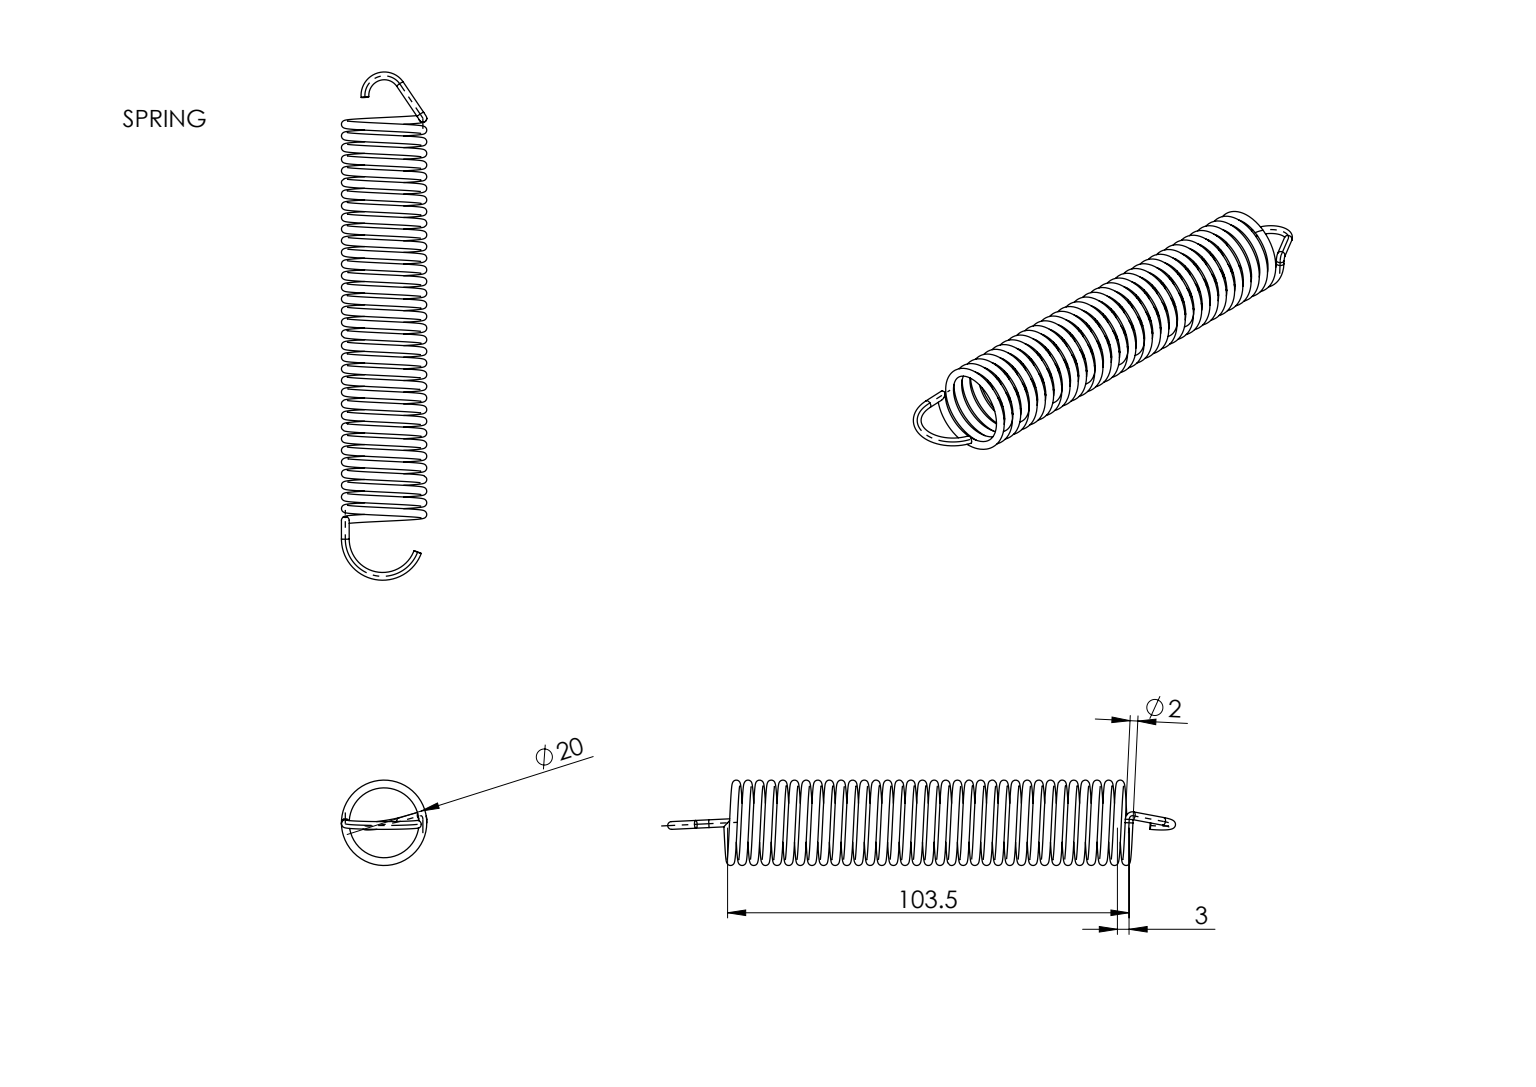
ISO-10303-21;
HEADER;
FILE_DESCRIPTION (('STEP AP214'),
    '1' );
FILE_NAME ('spring.step',
    '2026-10-08T07:58:12',
    ( '' ),
    ( '' ),
    'SwSTEP 2.0',
    'SolidWorks 2026',
    '' );
FILE_SCHEMA (( 'AUTOMOTIVE_DESIGN' ));
ENDSEC;

DATA;
#2=ORIENTED_EDGE ( 'NONE', *, *, #29028, .T. ) ;
#6=CARTESIAN_POINT ( 'NONE',  ( 2.517493886308900919, 214.5937144450984420, 40.40113791807857524 ) ) ;
#8=CARTESIAN_POINT ( 'NONE',  ( -10.00000000000000711, 206.9523078486584495, 26.49886208192143755 ) ) ;
#14=CARTESIAN_POINT ( 'NONE',  ( 6.500168698208244500, 202.3363017425938324, 1.298862081921434930 ) ) ;
#15=CARTESIAN_POINT ( 'NONE',  ( -8.118202686958039038, 201.1607312380087080, 39.20113791807857240 ) ) ;
#17=CARTESIAN_POINT ( 'NONE',  ( -8.118202686958039038, 201.1607312380087080, 30.20113791807856884 ) ) ;
#18=CARTESIAN_POINT ( 'NONE',  ( 6.220909254589680693, 198.5229672870052582, 103.4488620819214333 ) ) ;
#20=CARTESIAN_POINT ( 'NONE',  ( 4.903702542908435547, 213.8346818373419751, 96.54886208192142760 ) ) ;
#24=CARTESIAN_POINT ( 'NONE',  ( -12.00000000000000711, 207.0476921513413515, 12.50113791807856600 ) ) ;
#28=CARTESIAN_POINT ( 'NONE',  ( 0.05014649552810505201, 217.5146222423826714, 58.25113791807856245 ) ) ;
#35=CARTESIAN_POINT ( 'NONE',  ( -7.456977232089304408, 196.8216656703010301, 42.05113791807857382 ) ) ;
#38=CARTESIAN_POINT ( 'NONE',  ( -10.00000000000000711, 206.9523078486584495, 8.498862081921433997 ) ) ;
#41=CARTESIAN_POINT ( 'NONE',  ( -10.00000000000000711, 207.0476921513413515, 6.501137918078566003 ) ) ;
#42=CARTESIAN_POINT ( 'NONE',  ( -3.044812012440131443, 216.5253028482142952, 70.10113791807857808 ) ) ;
#45=CARTESIAN_POINT ( 'NONE',  ( -2.517493886309087880, 214.5937144450984135, 36.09886208192144608 ) ) ;
#48=CARTESIAN_POINT ( 'NONE',  ( 2.517493886308900919, 214.5937144450984420, 16.40113791807856458 ) ) ;
#49=CARTESIAN_POINT ( 'NONE',  ( -9.736236675708031640, 214.0148392665760753, 95.79886208192144181 ) ) ;
#54=CARTESIAN_POINT ( 'NONE',  ( 3.044812012440130555, 197.4746971517856764, 5.601137918078566535 ) ) ;
#55=CARTESIAN_POINT ( 'NONE',  ( 6.220909254589681581, 198.5229672870052582, 76.44886208192143329 ) ) ;
#58=CARTESIAN_POINT ( 'NONE',  ( 10.00000000000000711, 206.9523078486586201, 11.00113791807856600 ) ) ;
#61=CARTESIAN_POINT ( 'NONE',  ( -8.118202686958039038, 201.1607312380087080, 99.20113791807858661 ) ) ;
#63=CARTESIAN_POINT ( 'NONE',  ( 9.984503880673470277, 203.7031108863295401, 86.15113791807857524 ) ) ;
#66=CARTESIAN_POINT ( 'NONE',  ( -3.662846001189865142, 195.5725841191952838, 94.89886208192145034 ) ) ;
#71=CARTESIAN_POINT ( 'NONE',  ( -9.680171189290831535, 214.0920067884431148, 99.80113791807858092 ) ) ;
#74=CARTESIAN_POINT ( 'NONE',  ( -6.139770520408224463, 198.4640165459539105, 89.04886208192141339 ) ) ;
#76=CARTESIAN_POINT ( 'NONE',  ( 12.00000000000000711, 207.0476921513415220, 24.99886208192143400 ) ) ;
#78=CARTESIAN_POINT ( 'NONE',  ( 6.220909254589536808, 215.4770327129947702, 40.55113791807855250 ) ) ;
#80=CARTESIAN_POINT ( 'NONE',  ( -2.426778023690076225, 199.3768101843759553, 7.898862081921436129 ) ) ;
#83=CARTESIAN_POINT ( 'NONE',  ( 2.517493886309087436, 199.4062855549015865, 91.59886208192145318 ) ) ;
#86=CARTESIAN_POINT ( 'NONE',  ( 8.015496119326531499, 209.5516654185219636, 31.85113791807857453 ) ) ;
#92=CARTESIAN_POINT ( 'NONE',  ( 8.015496119326531499, 209.5516654185219636, 88.85113791807857808 ) ) ;
#96=CARTESIAN_POINT ( 'NONE',  ( 4.984841277089891776, 200.2242689037093726, 67.44886208192143329 ) ) ;
#99=CARTESIAN_POINT ( 'NONE',  ( 6.220909254589536808, 215.4770327129947987, 4.551137918078565825 ) ) ;
#104=CARTESIAN_POINT ( 'NONE',  ( -7.375838497908182134, 217.2372850707499765, 63.95113791807857240 ) ) ;
#106=CARTESIAN_POINT ( 'NONE',  ( -3.753561863808691168, 195.6020594897209435, 5.901137918078566358 ) ) ;
#107=CARTESIAN_POINT ( 'NONE',  ( 0.05014649552810506589, 217.5146222423826714, 88.25113791807858377 ) ) ;
#109=CARTESIAN_POINT ( 'NONE',  ( 12.00000000000000711, 207.0476921513415220, 48.99886208192143044 ) ) ;
#110=CARTESIAN_POINT ( 'NONE',  ( 3.135527875058981895, 197.5041725223112792, 61.59886208192143897 ) ) ;
#111=CARTESIAN_POINT ( 'NONE',  ( -0.05014649552807705357, 194.3824533091408000, 98.75113791807856956 ) ) ;
#113=CARTESIAN_POINT ( 'NONE',  ( -6.220909254589537696, 198.5229672870051161, 15.05113791807856671 ) ) ;
#114=CARTESIAN_POINT ( 'NONE',  ( 6.139770520408223575, 215.5359834540460611, 75.54886208192139918 ) ) ;
#117=CARTESIAN_POINT ( 'NONE',  ( -3.753561863808878130, 218.3979405102790281, 78.09886208192142476 ) ) ;
#119=CARTESIAN_POINT ( 'NONE',  ( -6.220909254589537696, 198.5229672870051161, 102.0511379180785383 ) ) ;
#122=CARTESIAN_POINT ( 'NONE',  ( 2.426778023690075337, 214.6231898156240447, 60.39886208192144323 ) ) ;
#130=CARTESIAN_POINT ( 'NONE',  ( 8.118202686958138514, 201.1607312380088501, 55.29886208192144181 ) ) ;
#135=CARTESIAN_POINT ( 'NONE',  ( -4.903702542908436435, 200.1653181626580249, 38.04886208192144892 ) ) ;
#136=CARTESIAN_POINT ( 'NONE',  ( 10.01549611932653860, 210.2015048109876716, 67.85113791807857808 ) ) ;
#138=CARTESIAN_POINT ( 'NONE',  ( 10.01549611932653860, 210.2015048109876716, 58.85113791807856387 ) ) ;
#140=CARTESIAN_POINT ( 'NONE',  ( -8.118202686958039038, 201.1607312380087080, 24.20113791807856884 ) ) ;
#141=CARTESIAN_POINT ( 'NONE',  ( -8.000000000000008882, 207.0476921513413515, 18.50113791807856956 ) ) ;
#145=CARTESIAN_POINT ( 'NONE',  ( -7.375838497908182134, 217.2372850707499765, 39.95113791807856529 ) ) ;
#147=CARTESIAN_POINT ( 'NONE',  ( 9.984503880673470277, 203.7031108863295401, 83.15113791807853261 ) ) ;
#148=CARTESIAN_POINT ( 'NONE',  ( -0.05014649552810635652, 196.4853777576173002, 56.75113791807856245 ) ) ;
#149=CARTESIAN_POINT ( 'NONE',  ( -9.736236675708031640, 214.0148392665760753, 23.79886208192143826 ) ) ;
#150=CARTESIAN_POINT ( 'NONE',  ( 0.05014649552828275014, 196.4853777576173002, 31.74886208192143044 ) ) ;
#153=CARTESIAN_POINT ( 'NONE',  ( -9.680171189290831535, 214.0920067884431148, 69.80113791807856671 ) ) ;
#154=CARTESIAN_POINT ( 'NONE',  ( -8.000000000000008882, 207.0476921513413515, 87.50113791807856956 ) ) ;
#156=CARTESIAN_POINT ( 'NONE',  ( 8.118202686958138514, 201.1607312380088501, 49.29886208192143471 ) ) ;
#160=CARTESIAN_POINT ( 'NONE',  ( -9.736236675708031640, 214.0148392665760753, 50.79886208192143471 ) ) ;
#164=EDGE_CURVE ( 'NONE', #11179, #4391, #29721, .T. ) ;
#167=CARTESIAN_POINT ( 'NONE',  ( -6.444103211791042618, 211.7408657792732356, 39.80113791807857382 ) ) ;
#169=CARTESIAN_POINT ( 'NONE',  ( -10.00000000000000711, 206.9523078486584495, 23.49886208192143755 ) ) ;
#176=CARTESIAN_POINT ( 'NONE',  ( -7.984503880673422316, 204.3529502787951628, 8.348862081921435419 ) ) ;
#178=CARTESIAN_POINT ( 'NONE',  ( -8.118202686958039038, 201.1607312380087080, 42.20113791807857240 ) ) ;
#180=CARTESIAN_POINT ( 'NONE',  ( -9.984503880673473830, 210.2968891136704315, 30.65113791807856813 ) ) ;
#181=CARTESIAN_POINT ( 'NONE',  ( -6.139770520408224463, 198.4640165459539105, 104.0488620819214276 ) ) ;
#184=CARTESIAN_POINT ( 'NONE',  ( -6.444103211790928043, 202.2591342207265939, 92.19886208192143329 ) ) ;
#188=CARTESIAN_POINT ( 'NONE',  ( 3.662846001190051659, 195.5725841191953691, 5.601137918078566535 ) ) ;
#192=CARTESIAN_POINT ( 'NONE',  ( 6.139770520408368348, 198.4640165459539674, 56.45113791807857950 ) ) ;
#193=CARTESIAN_POINT ( 'NONE',  ( -10.01549611932653860, 203.7984951890123000, 27.35113791807856742 ) ) ;
#200=CARTESIAN_POINT ( 'NONE',  ( 3.662846001190051659, 195.5725841191953691, 41.60113791807857098 ) ) ;
#202=CARTESIAN_POINT ( 'NONE',  ( -8.118202686958138514, 212.8392687619910930, 11.79886208192143471 ) ) ;
#205=CARTESIAN_POINT ( 'NONE',  ( 10.00000000000000711, 206.9523078486586201, 71.00113791807858377 ) ) ;
#208=CARTESIAN_POINT ( 'NONE',  ( 4.984841277089891776, 200.2242689037093726, 31.44886208192143684 ) ) ;
#211=CARTESIAN_POINT ( 'NONE',  ( -8.015496119326531499, 204.4483345814780364, 9.351137918078563871 ) ) ;
#214=CARTESIAN_POINT ( 'NONE',  ( 11.98450388067341876, 210.9467285061363953, 93.84886208192143897 ) ) ;
#219=CARTESIAN_POINT ( 'NONE',  ( -6.139770520408369237, 215.5359834540460042, 6.951137918078566180 ) ) ;
#221=CARTESIAN_POINT ( 'NONE',  ( 8.062137200540822946, 212.9164362838583315, 81.69886208192143329 ) ) ;
#225=CARTESIAN_POINT ( 'NONE',  ( 8.062137200540920645, 201.0835637161417822, 17.30113791807856671 ) ) ;
#232=CARTESIAN_POINT ( 'NONE',  ( -10.01549611932653860, 203.7984951890123284, 81.35113791807857808 ) ) ;
#236=CARTESIAN_POINT ( 'NONE',  ( 3.753561863808876797, 195.6020594897209719, 94.59886208192145318 ) ) ;
#242=CARTESIAN_POINT ( 'NONE',  ( -12.01549611932652972, 203.1486557965464499, 96.35113791807857808 ) ) ;
#246=CARTESIAN_POINT ( 'NONE',  ( -6.220909254589682469, 215.4770327129947134, 95.94886208192143329 ) ) ;
#247=CARTESIAN_POINT ( 'NONE',  ( -9.736236675708031640, 214.0148392665760753, 26.79886208192143826 ) ) ;
#249=CARTESIAN_POINT ( 'NONE',  ( 10.00000000000000711, 206.9523078486586201, 47.00113791807856956 ) ) ;
#251=CARTESIAN_POINT ( 'NONE',  ( -3.044812012439970683, 197.4746971517856196, 103.8988620819214361 ) ) ;
#254=CARTESIAN_POINT ( 'NONE',  ( -6.444103211790928043, 202.2591342207265939, 92.19886208192143329 ) ) ;
#256=CARTESIAN_POINT ( 'NONE',  ( 4.903702542908601636, 200.1653181626581102, 32.45113791807857240 ) ) ;
#262=CARTESIAN_POINT ( 'NONE',  ( 7.984503880673485376, 204.3529502787953902, 86.15113791807856103 ) ) ;
#266=CARTESIAN_POINT ( 'NONE',  ( 8.015496119326595448, 204.4483345814782638, 61.14886208192145034 ) ) ;
#269=CARTESIAN_POINT ( 'NONE',  ( 3.044812012440130555, 197.4746971517856764, -0.3988620819214342972 ) ) ;
#272=CARTESIAN_POINT ( 'NONE',  ( -7.375838497908182134, 217.2372850707499765, 66.95113791807857240 ) ) ;
#274=CARTESIAN_POINT ( 'NONE',  ( -8.062137200540920645, 212.9164362838581894, 87.80113791807856671 ) ) ;
#276=CARTESIAN_POINT ( 'NONE',  ( -9.680171189290716072, 199.9079932115567146, 50.19886208192144039 ) ) ;
#277=CARTESIAN_POINT ( 'NONE',  ( 3.044812012439969795, 216.5253028482143520, 57.39886208192143613 ) ) ;
#278=CARTESIAN_POINT ( 'NONE',  ( -12.01549611932652972, 203.1486557965464499, 93.35113791807857808 ) ) ;
#280=CARTESIAN_POINT ( 'NONE',  ( -10.00000000000000711, 207.0476921513413515, 12.50113791807856778 ) ) ;
#281=CARTESIAN_POINT ( 'NONE',  ( -3.044812012439970683, 197.4746971517856196, 76.89886208192143613 ) ) ;
#284=CARTESIAN_POINT ( 'NONE',  ( 8.118202686958039038, 212.8392687619912635, 100.7011379180785866 ) ) ;
#286=CARTESIAN_POINT ( 'NONE',  ( -0.05014649552828365914, 215.4116977939061144, 66.24886208192143044 ) ) ;
#289=DIRECTION ( 'NONE',  ( 0.000000000000000000, 0.9988620819214357738, 0.04769215134144196705 ) ) ;
#292=CARTESIAN_POINT ( 'NONE',  ( 6.444103211791042618, 202.2591342207267644, 59.30113791807857382 ) ) ;
#293=CARTESIAN_POINT ( 'NONE',  ( 3.135527875058981895, 197.5041725223112792, 52.59886208192143897 ) ) ;
#294=CARTESIAN_POINT ( 'NONE',  ( -9.945352646237287431, 205.9548993908332193, 104.4520571433695579 ) ) ;
#296=CARTESIAN_POINT ( 'NONE',  ( 2.426778023690075337, 214.6231898156240447, 36.39886208192144323 ) ) ;
#297=CARTESIAN_POINT ( 'NONE',  ( 9.984503880673470277, 203.7031108863295401, 83.15113791807853261 ) ) ;
#300=CARTESIAN_POINT ( 'NONE',  ( 9.984503880673470277, 203.7031108863295401, 56.15113791807856103 ) ) ;
#301=CARTESIAN_POINT ( 'NONE',  ( 8.118202686958039038, 212.8392687619912635, 25.70113791807856529 ) ) ;
#302=CARTESIAN_POINT ( 'NONE',  ( 4.984841277089725686, 213.7757310962907411, 13.55113791807856849 ) ) ;
#306=CARTESIAN_POINT ( 'NONE',  ( 7.375838497908181246, 196.7627149292499666, 35.45113791807855819 ) ) ;
#308=CARTESIAN_POINT ( 'NONE',  ( -6.220909254589537696, 198.5229672870051161, 90.05113791807858092 ) ) ;
#309=CARTESIAN_POINT ( 'NONE',  ( -10.00000000000000711, 207.0476921513413515, 60.50113791807857666 ) ) ;
#310=CARTESIAN_POINT ( 'NONE',  ( 12.01549611932659367, 203.1486557965466773, 22.14886208192143613 ) ) ;
#311=CARTESIAN_POINT ( 'NONE',  ( -0.05014649552828402690, 217.5146222423826714, 24.24886208192143044 ) ) ;
#313=CARTESIAN_POINT ( 'NONE',  ( 12.00000000000000711, 206.9523078486586485, 71.00113791807856956 ) ) ;
#314=CARTESIAN_POINT ( 'NONE',  ( 7.984503880673485376, 204.3529502787953902, 92.15113791807856103 ) ) ;
#315=CARTESIAN_POINT ( 'NONE',  ( -8.118202686958138514, 212.8392687619910930, 53.79886208192143471 ) ) ;
#318=CARTESIAN_POINT ( 'NONE',  ( -7.456977232089471386, 217.1783343296987709, 50.94886208192143329 ) ) ;
#323=CARTESIAN_POINT ( 'NONE',  ( 8.000000000000008882, 206.9523078486586485, 44.00113791807857666 ) ) ;
#326=CARTESIAN_POINT ( 'NONE',  ( 10.01549611932659545, 203.7984951890123853, 19.14886208192142902 ) ) ;
#332=CARTESIAN_POINT ( 'NONE',  ( 8.015496119326595448, 204.4483345814782638, 10.14886208192143435 ) ) ;
#333=CARTESIAN_POINT ( 'NONE',  ( -6.220909254589537696, 198.5229672870051161, 48.05113791807858092 ) ) ;
#336=CARTESIAN_POINT ( 'NONE',  ( 10.00000000000000711, 206.9523078486586201, 23.00113791807856600 ) ) ;
#339=CARTESIAN_POINT ( 'NONE',  ( 8.015496119326595448, 204.4483345814782638, 88.14886208192143613 ) ) ;
#343=CARTESIAN_POINT ( 'NONE',  ( 0.05014649552807549926, 219.6175466908591716, 7.251137918078565114 ) ) ;
#347=CARTESIAN_POINT ( 'NONE',  ( 6.139770520408368348, 198.4640165459539674, 59.45113791807855819 ) ) ;
#348=CARTESIAN_POINT ( 'NONE',  ( 8.062137200540920645, 201.0835637161417822, 32.30113791807857382 ) ) ;
#353=CARTESIAN_POINT ( 'NONE',  ( 10.01549611932659367, 203.7984951890124421, 4.148862081921434353 ) ) ;
#356=CARTESIAN_POINT ( 'NONE',  ( 7.375838497908181246, 196.7627149292499666, 38.45113791807856529 ) ) ;
#358=CARTESIAN_POINT ( 'NONE',  ( -10.01549611932659722, 210.2015048109875011, 23.64886208192142902 ) ) ;
#362=CARTESIAN_POINT ( 'NONE',  ( -6.139770520408369237, 215.5359834540460042, 66.95113791807858661 ) ) ;
#366=CARTESIAN_POINT ( 'NONE',  ( -2.517493886308901807, 199.4062855549015012, 17.90113791807856458 ) ) ;
#367=EDGE_CURVE ( 'NONE', #11826, #6694, #28121, .T. ) ;
#369=CARTESIAN_POINT ( 'NONE',  ( -12.00000000000000711, 206.9523078486584780, 101.4988620819214304 ) ) ;
#374=CARTESIAN_POINT ( 'NONE',  ( -6.139770520408369237, 215.5359834540460042, 9.951137918078567068 ) ) ;
#376=CARTESIAN_POINT ( 'NONE',  ( 6.220909254589681581, 198.5229672870052582, 82.44886208192141908 ) ) ;
#379=CARTESIAN_POINT ( 'NONE',  ( -10.01549611932653860, 203.7984951890123284, 9.351137918078569200 ) ) ;
#384=CARTESIAN_POINT ( 'NONE',  ( -6.220909254589537696, 198.5229672870051161, 99.05113791807858092 ) ) ;
#386=CARTESIAN_POINT ( 'NONE',  ( -8.118202686958039038, 201.1607312380087080, 81.20113791807857240 ) ) ;
#389=CARTESIAN_POINT ( 'NONE',  ( -7.456977232089471386, 217.1783343296987709, 92.94886208192144750 ) ) ;
#400=CARTESIAN_POINT ( 'NONE',  ( -8.062137200540822946, 201.0835637161416400, 95.19886208192143329 ) ) ;
#401=CARTESIAN_POINT ( 'NONE',  ( -3.753561863808878130, 218.3979405102790281, 33.09886208192143187 ) ) ;
#403=CARTESIAN_POINT ( 'NONE',  ( -8.118202686958039038, 201.1607312380087080, 39.20113791807857240 ) ) ;
#406=CARTESIAN_POINT ( 'NONE',  ( 4.984841277089891776, 200.2242689037093726, 1.448862081921434841 ) ) ;
#410=CARTESIAN_POINT ( 'NONE',  ( -2.517493886309087880, 214.5937144450984135, 90.09886208192143897 ) ) ;
#412=CARTESIAN_POINT ( 'NONE',  ( -8.000000000000008882, 207.0476921513413515, 27.50113791807856956 ) ) ;
#419=CARTESIAN_POINT ( 'NONE',  ( 7.984503880673485376, 204.3529502787953902, 89.15113791807856103 ) ) ;
#423=CARTESIAN_POINT ( 'NONE',  ( -8.015496119326597224, 209.5516654185217362, 77.64886208192143613 ) ) ;
#427=CARTESIAN_POINT ( 'NONE',  ( -9.984503880673475606, 210.2968891136704315, 15.65113791807856636 ) ) ;
#432=CARTESIAN_POINT ( 'NONE',  ( 12.01549611932652972, 210.8513442034534933, 76.85113791807856387 ) ) ;
#436=CARTESIAN_POINT ( 'NONE',  ( 10.01549611932653860, 210.2015048109876716, 97.85113791807857808 ) ) ;
#439=CARTESIAN_POINT ( 'NONE',  ( 7.375838497908012492, 217.2372850707501186, 51.54886208192144181 ) ) ;
#440=CARTESIAN_POINT ( 'NONE',  ( 6.139770520408223575, 215.5359834540460611, 69.54886208192142760 ) ) ;
#441=CARTESIAN_POINT ( 'NONE',  ( -3.753561863808878130, 218.3979405102790281, 6.098862081921433642 ) ) ;
#443=AXIS2_PLACEMENT_3D ( 'NONE', #26403, #3062, #13451 ) ;
#444=CARTESIAN_POINT ( 'NONE',  ( 3.135527875058820690, 216.4958274776887492, 10.40113791807856636 ) ) ;
#447=CARTESIAN_POINT ( 'NONE',  ( -3.044812012439970683, 197.4746971517856196, 79.89886208192143613 ) ) ;
#450=CARTESIAN_POINT ( 'NONE',  ( -6.139770520408369237, 215.5359834540460042, 99.95113791807855819 ) ) ;
#453=CARTESIAN_POINT ( 'NONE',  ( 6.444103211790928043, 211.7408657792734061, 60.69886208192144750 ) ) ;
#461=CARTESIAN_POINT ( 'NONE',  ( 8.015496119326531499, 209.5516654185219636, 58.85113791807857098 ) ) ;
#466=CARTESIAN_POINT ( 'NONE',  ( 7.984503880673422316, 209.6470497212048372, 36.84886208192142476 ) ) ;
#468=CARTESIAN_POINT ( 'NONE',  ( -10.00000000000000711, 207.0476921513413515, 84.50113791807856956 ) ) ;
#470=CARTESIAN_POINT ( 'NONE',  ( 8.118202686958039038, 212.8392687619912635, 70.70113791807857240 ) ) ;
#473=CARTESIAN_POINT ( 'NONE',  ( -2.426778023690262742, 214.6231898156240163, 19.10113791807856742 ) ) ;
#477=CARTESIAN_POINT ( 'NONE',  ( -12.01549611932652972, 203.1486557965464499, 39.35113791807856387 ) ) ;
#479=CARTESIAN_POINT ( 'NONE',  ( 3.044812012440130555, 197.4746971517856764, 98.60113791807857808 ) ) ;
#480=CARTESIAN_POINT ( 'NONE',  ( 10.01549611932653860, 210.2015048109876716, 61.85113791807857098 ) ) ;
#482=CARTESIAN_POINT ( 'NONE',  ( 9.736236675708031640, 199.9851607334238963, 22.29886208192143826 ) ) ;
#483=CARTESIAN_POINT ( 'NONE',  ( 10.00000000000000711, 207.0476921513415220, 36.99886208192143755 ) ) ;
#485=CARTESIAN_POINT ( 'NONE',  ( -11.98450388067348804, 210.9467285061362247, 69.65113791807856103 ) ) ;
#486=CARTESIAN_POINT ( 'NONE',  ( 8.015496119326531499, 209.5516654185219636, 85.85113791807857808 ) ) ;
#487=CARTESIAN_POINT ( 'NONE',  ( 6.139770520408223575, 215.5359834540460611, 48.54886208192143471 ) ) ;
#489=ORIENTED_EDGE ( 'NONE', *, *, #23335, .T. ) ;
#490=CARTESIAN_POINT ( 'NONE',  ( -3.662846001189865142, 195.5725841191952838, 52.89886208192143613 ) ) ;
#497=CARTESIAN_POINT ( 'NONE',  ( 11.98450388067341876, 210.9467285061363953, 54.84886208192143187 ) ) ;
#499=CARTESIAN_POINT ( 'NONE',  ( 6.500168698208129925, 211.6636982574063381, 37.70113791807857240 ) ) ;
#501=CARTESIAN_POINT ( 'NONE',  ( -3.044812012439970683, 197.4746971517856196, 22.89886208192143613 ) ) ;
#505=UNCERTAINTY_MEASURE_WITH_UNIT (LENGTH_MEASURE( 1.000000000000000082E-05 ), #16997, 'distance_accuracy_value', 'NONE');
#509=CARTESIAN_POINT ( 'NONE',  ( -4.984841277089891776, 213.7757310962905990, 2.948862081921435063 ) ) ;
#510=CARTESIAN_POINT ( 'NONE',  ( -9.984503880673473830, 210.2968891136704315, 54.65113791807858235 ) ) ;
#512=CARTESIAN_POINT ( 'NONE',  ( 0.05014649552810505201, 217.5146222423826714, 34.25113791807856956 ) ) ;
#515=CARTESIAN_POINT ( 'NONE',  ( -8.015496119326597224, 209.5516654185217362, 95.64886208192143613 ) ) ;
#519=CARTESIAN_POINT ( 'NONE',  ( 9.680171189290831535, 199.9079932115568852, 11.30113791807856671 ) ) ;
#520=AXIS2_PLACEMENT_3D ( 'NONE', #21332, #31728, #8401 ) ;
#523=CARTESIAN_POINT ( 'NONE',  ( -6.220909254589537696, 198.5229672870051161, 54.05113791807856671 ) ) ;
#524=CARTESIAN_POINT ( 'NONE',  ( -8.118202686958039038, 201.1607312380087080, 27.20113791807856884 ) ) ;
#530=CARTESIAN_POINT ( 'NONE',  ( -7.375838497908182134, 217.2372850707499765, 36.95113791807856529 ) ) ;
#532=CARTESIAN_POINT ( 'NONE',  ( 0.05014649552828275708, 196.4853777576173002, 25.74886208192143400 ) ) ;
#535=CARTESIAN_POINT ( 'NONE',  ( 3.135527875058820690, 216.4958274776887492, 82.40113791807857524 ) ) ;
#541=CARTESIAN_POINT ( 'NONE',  ( -6.444103211791042618, 211.7408657792732356, 9.801137918078564937 ) ) ;
#544=CARTESIAN_POINT ( 'NONE',  ( -9.680171189290716072, 199.9079932115567146, 98.19886208192144750 ) ) ;
#550=CARTESIAN_POINT ( 'NONE',  ( 6.139770520408223575, 215.5359834540460611, 81.54886208192144181 ) ) ;
#552=CARTESIAN_POINT ( 'NONE',  ( -8.118202686958039038, 201.1607312380087080, 18.20113791807856884 ) ) ;
#557=CARTESIAN_POINT ( 'NONE',  ( -6.220909254589537696, 198.5229672870051161, 87.05113791807856671 ) ) ;
#560=CARTESIAN_POINT ( 'NONE',  ( -9.736236675708031640, 214.0148392665760753, 95.79886208192144181 ) ) ;
#568=CARTESIAN_POINT ( 'NONE',  ( -8.062137200540822946, 201.0835637161416400, 92.19886208192143329 ) ) ;
#569=CARTESIAN_POINT ( 'NONE',  ( -7.375838497908014268, 196.7627149292498530, 35.04886208192143471 ) ) ;
#571=CARTESIAN_POINT ( 'NONE',  ( 3.044812012440130555, 197.4746971517856764, 56.60113791807857098 ) ) ;
#573=CARTESIAN_POINT ( 'NONE',  ( 8.015496119326595448, 204.4483345814782638, 7.148862081921435241 ) ) ;
#577=CARTESIAN_POINT ( 'NONE',  ( -4.903702542908436435, 200.1653181626580249, 95.04886208192144181 ) ) ;
#578=CARTESIAN_POINT ( 'NONE',  ( -4.984841277089726574, 200.2242689037092305, 33.05113791807857382 ) ) ;
#585=CARTESIAN_POINT ( 'NONE',  ( -4.984841277089726574, 200.2242689037092305, 96.05113791807858092 ) ) ;
#588=CARTESIAN_POINT ( 'NONE',  ( 7.984503880673422316, 209.6470497212048372, 69.84886208192143897 ) ) ;
#592=CARTESIAN_POINT ( 'NONE',  ( 10.01549611932653860, 210.2015048109876716, 10.85113791807856565 ) ) ;
#596=CARTESIAN_POINT ( 'NONE',  ( 0.05014649552807549926, 219.6175466908591716, 73.25113791807858377 ) ) ;
#599=CARTESIAN_POINT ( 'NONE',  ( 3.044812012440130555, 197.4746971517856764, 98.60113791807857808 ) ) ;
#602=CARTESIAN_POINT ( 'NONE',  ( -12.01549611932659722, 210.8513442034533227, 62.64886208192143613 ) ) ;
#603=CARTESIAN_POINT ( 'NONE',  ( -9.984503880673420539, 203.7031108863293980, 71.34886208192141055 ) ) ;
#604=CARTESIAN_POINT ( 'NONE',  ( -12.00000000000000711, 206.9523078486584780, 8.498862081921435774 ) ) ;
#606=CARTESIAN_POINT ( 'NONE',  ( -3.135527875058821579, 197.5041725223112223, 14.90113791807856636 ) ) ;
#607=CARTESIAN_POINT ( 'NONE',  ( -6.220909254589682469, 215.4770327129946850, 77.94886208192140487 ) ) ;
#609=CARTESIAN_POINT ( 'NONE',  ( 3.044812012440130555, 197.4746971517856764, 101.6011379180785781 ) ) ;
#612=CARTESIAN_POINT ( 'NONE',  ( -2.517493886309087880, 214.5937144450984135, 60.09886208192145318 ) ) ;
#621=CARTESIAN_POINT ( 'NONE',  ( -2.517493886308901807, 199.4062855549015012, 62.90113791807858945 ) ) ;
#627=CARTESIAN_POINT ( 'NONE',  ( 7.984503880673422316, 209.6470497212048372, 45.84886208192143897 ) ) ;
#628=CARTESIAN_POINT ( 'NONE',  ( -10.01549611932653860, 203.7984951890123284, 78.35113791807857808 ) ) ;
#630=CARTESIAN_POINT ( 'NONE',  ( -8.118202686958039038, 201.1607312380087080, 63.20113791807857240 ) ) ;
#632=CARTESIAN_POINT ( 'NONE',  ( 2.517493886308900919, 214.5937144450984420, 25.40113791807857169 ) ) ;
#635=CARTESIAN_POINT ( 'NONE',  ( -11.98450388067348804, 210.9467285061362247, 45.65113791807856813 ) ) ;
#638=CARTESIAN_POINT ( 'NONE',  ( 3.044812012440130555, 197.4746971517856764, 95.60113791807857808 ) ) ;
#639=CARTESIAN_POINT ( 'NONE',  ( 10.01549611932653860, 210.2015048109876716, 67.85113791807857808 ) ) ;
#640=CARTESIAN_POINT ( 'NONE',  ( -9.736236675708031640, 214.0148392665760753, 35.79886208192143471 ) ) ;
#641=CARTESIAN_POINT ( 'NONE',  ( 10.00000000000000711, 207.0476921513415220, 39.99886208192143755 ) ) ;
#644=CARTESIAN_POINT ( 'NONE',  ( -3.662846001190052991, 218.4274158808045740, 79.10113791807857808 ) ) ;
#645=CARTESIAN_POINT ( 'NONE',  ( -8.015496119326531499, 204.4483345814780364, 84.35113791807857808 ) ) ;
#647=CARTESIAN_POINT ( 'NONE',  ( 0.05014649552828275708, 196.4853777576173002, 46.74886208192143755 ) ) ;
#650=CARTESIAN_POINT ( 'NONE',  ( -3.662846001189865142, 195.5725841191952838, 64.89886208192143613 ) ) ;
#657=CARTESIAN_POINT ( 'NONE',  ( 4.903702542908601636, 200.1653181626581102, 47.45113791807857950 ) ) ;
#659=CARTESIAN_POINT ( 'NONE',  ( -10.00000000000000711, 206.9523078486584495, 35.49886208192143044 ) ) ;
#665=CARTESIAN_POINT ( 'NONE',  ( 4.984841277089891776, 200.2242689037093726, 19.44886208192143329 ) ) ;
#666=CARTESIAN_POINT ( 'NONE',  ( 6.139770520408368348, 198.4640165459539674, 47.45113791807857950 ) ) ;
#668=CARTESIAN_POINT ( 'NONE',  ( -6.220909254589537696, 198.5229672870051161, 39.05113791807856671 ) ) ;
#671=CARTESIAN_POINT ( 'NONE',  ( -2.517493886309087880, 214.5937144450984135, 96.09886208192143897 ) ) ;
#677=CARTESIAN_POINT ( 'NONE',  ( -3.662846001190052991, 218.4274158808045740, 22.10113791807856742 ) ) ;
#680=CARTESIAN_POINT ( 'NONE',  ( 3.135527875058820690, 216.4958274776887492, 64.40113791807857524 ) ) ;
#681=CARTESIAN_POINT ( 'NONE',  ( 8.062137200540920645, 201.0835637161417822, 41.30113791807857382 ) ) ;
#684=CARTESIAN_POINT ( 'NONE',  ( -10.01549611932659545, 210.2015048109875011, 8.648862081921434353 ) ) ;
#687=CARTESIAN_POINT ( 'NONE',  ( -0.05014649552807705357, 194.3824533091408000, 44.75113791807856956 ) ) ;
#689=CARTESIAN_POINT ( 'NONE',  ( 8.118202686958138514, 201.1607312380088501, 22.29886208192143826 ) ) ;
#693=CARTESIAN_POINT ( 'NONE',  ( -0.05014649552810635652, 196.4853777576173002, 83.75113791807856956 ) ) ;
#699=CARTESIAN_POINT ( 'NONE',  ( -6.500168698208129925, 202.3363017425936050, 21.20113791807856529 ) ) ;
#703=CARTESIAN_POINT ( 'NONE',  ( 3.135527875058981895, 197.5041725223112792, 7.598862081921435419 ) ) ;
#710=CARTESIAN_POINT ( 'NONE',  ( 10.01549611932659545, 203.7984951890123853, 85.14886208192143613 ) ) ;
#712=CARTESIAN_POINT ( 'NONE',  ( 10.01549611932653860, 210.2015048109876716, 25.85113791807856742 ) ) ;
#714=CARTESIAN_POINT ( 'NONE',  ( 3.662846001189864698, 218.4274158808046593, 75.39886208192143613 ) ) ;
#719=CARTESIAN_POINT ( 'NONE',  ( 10.00000000000000711, 206.9523078486586201, 86.00113791807858377 ) ) ;
#722=CARTESIAN_POINT ( 'NONE',  ( -8.062137200540920645, 212.9164362838581894, 39.80113791807857382 ) ) ;
#730=CARTESIAN_POINT ( 'NONE',  ( 7.456977232089302632, 217.1783343296989131, 7.551137918078564049 ) ) ;
#735=CARTESIAN_POINT ( 'NONE',  ( -6.139770520408224463, 198.4640165459539105, 98.04886208192142760 ) ) ;
#736=CARTESIAN_POINT ( 'NONE',  ( 12.01549611932659367, 203.1486557965466773, 37.14886208192143613 ) ) ;
#738=CARTESIAN_POINT ( 'NONE',  ( 10.01549611932653860, 210.2015048109876716, 55.85113791807857808 ) ) ;
#740=CARTESIAN_POINT ( 'NONE',  ( -4.984841277089891776, 213.7757310962905990, 14.94886208192143506 ) ) ;
#743=CARTESIAN_POINT ( 'NONE',  ( -6.444103211790928043, 202.2591342207265939, 86.19886208192144750 ) ) ;
#745=CARTESIAN_POINT ( 'NONE',  ( -2.426778023690262742, 214.6231898156240163, 34.10113791807857098 ) ) ;
#752=CARTESIAN_POINT ( 'NONE',  ( 4.903702542908601636, 200.1653181626581102, 95.45113791807858661 ) ) ;
#755=CARTESIAN_POINT ( 'NONE',  ( 8.000000000000008882, 207.0476921513415220, 75.99886208192144466 ) ) ;
#759=CARTESIAN_POINT ( 'NONE',  ( -9.984503880673475606, 210.2968891136704315, 6.651137918078565470 ) ) ;
#763=CARTESIAN_POINT ( 'NONE',  ( 7.456977232089302632, 217.1783343296989131, 73.55113791807856671 ) ) ;
#765=CARTESIAN_POINT ( 'NONE',  ( 10.01549611932653860, 210.2015048109876716, 100.8511379180785639 ) ) ;
#769=CARTESIAN_POINT ( 'NONE',  ( 10.00000000000000711, 207.0476921513415220, 0.9988620819214343305 ) ) ;
#770=CARTESIAN_POINT ( 'NONE',  ( 12.00000000000000711, 207.0476921513415220, 60.99886208192143044 ) ) ;
#771=CARTESIAN_POINT ( 'NONE',  ( -0.05014649552828402690, 217.5146222423826714, 66.24886208192143044 ) ) ;
#773=CARTESIAN_POINT ( 'NONE',  ( 7.456977232089471386, 196.8216656703012006, 4.448862081921434175 ) ) ;
#775=CARTESIAN_POINT ( 'NONE',  ( -8.118202686958039038, 201.1607312380087080, 21.20113791807856529 ) ) ;
#777=CARTESIAN_POINT ( 'NONE',  ( 8.118202686958138514, 201.1607312380088501, 82.29886208192144181 ) ) ;
#779=DIRECTION ( 'NONE',  ( -0.1461455375466716444, 0.9854922318508084755, -0.08629335326029916042 ) ) ;
#782=CARTESIAN_POINT ( 'NONE',  ( -7.984503880673422316, 204.3529502787951628, 62.34886208192144608 ) ) ;
#787=FACE_OUTER_BOUND ( 'NONE', #21644, .T. ) ;
#788=MECHANICAL_DESIGN_GEOMETRIC_PRESENTATION_REPRESENTATION('',(#15484),#5146);
#793=CARTESIAN_POINT ( 'NONE',  ( 4.984841277089725686, 213.7757310962907411, 67.55113791807856671 ) ) ;
#797=CARTESIAN_POINT ( 'NONE',  ( 8.015496119326595448, 204.4483345814782638, 40.14886208192143613 ) ) ;
#798=CARTESIAN_POINT ( 'NONE',  ( 0.05014649552810505201, 217.5146222423826714, 76.25113791807855534 ) ) ;
#799=CARTESIAN_POINT ( 'NONE',  ( -3.135527875058821579, 197.5041725223112223, 68.90113791807857524 ) ) ;
#800=DIRECTION ( 'NONE',  ( 0.9366133782696114407, 0.000000000000000000, 0.3503646381220365535 ) ) ;
#801=CARTESIAN_POINT ( 'NONE',  ( -2.517493886308901807, 199.4062855549015012, 23.90113791807857169 ) ) ;
#805=CARTESIAN_POINT ( 'NONE',  ( -11.98450388067348804, 210.9467285061362247, 51.65113791807857524 ) ) ;
#807=CARTESIAN_POINT ( 'NONE',  ( 6.220909254589536808, 215.4770327129947702, 94.55113791807858092 ) ) ;
#808=CARTESIAN_POINT ( 'NONE',  ( 6.220909254589536808, 215.4770327129947987, 64.55113791807858092 ) ) ;
#809=CARTESIAN_POINT ( 'NONE',  ( -12.01549611932659722, 210.8513442034533227, 29.64886208192143968 ) ) ;
#810=CARTESIAN_POINT ( 'NONE',  ( -8.062137200540822946, 201.0835637161416400, 38.19886208192143329 ) ) ;
#812=CARTESIAN_POINT ( 'NONE',  ( 3.662846001190051659, 195.5725841191953691, 77.60113791807854966 ) ) ;
#813=CARTESIAN_POINT ( 'NONE',  ( 2.426778023690261410, 199.3768101843759837, 101.6011379180785781 ) ) ;
#815=CARTESIAN_POINT ( 'NONE',  ( -6.220909254589682469, 215.4770327129946850, 47.94886208192144039 ) ) ;
#818=CARTESIAN_POINT ( 'NONE',  ( 3.753561863808876797, 195.6020594897209719, 61.59886208192143897 ) ) ;
#820=CARTESIAN_POINT ( 'NONE',  ( -6.444103211790928043, 202.2591342207265939, 32.19886208192144039 ) ) ;
#826=CARTESIAN_POINT ( 'NONE',  ( 7.984503880673485376, 204.3529502787953902, 56.15113791807857524 ) ) ;
#828=CARTESIAN_POINT ( 'NONE',  ( 3.044812012439969795, 216.5253028482143520, 30.39886208192143613 ) ) ;
#834=CARTESIAN_POINT ( 'NONE',  ( 2.517493886309087436, 199.4062855549015865, 16.59886208192143897 ) ) ;
#835=CARTESIAN_POINT ( 'NONE',  ( -3.044812012440131443, 216.5253028482142952, 49.10113791807857808 ) ) ;
#837=CARTESIAN_POINT ( 'NONE',  ( 8.062137200540920645, 201.0835637161417822, 35.30113791807857382 ) ) ;
#840=CARTESIAN_POINT ( 'NONE',  ( -4.903702542908436435, 200.1653181626580249, 104.0488620819214560 ) ) ;
#844=CARTESIAN_POINT ( 'NONE',  ( -7.456977232089304408, 196.8216656703010301, 21.05113791807857027 ) ) ;
#847=CARTESIAN_POINT ( 'NONE',  ( -6.139770520408369237, 215.5359834540460042, 66.95113791807858661 ) ) ;
#848=CARTESIAN_POINT ( 'NONE',  ( -10.01549611932653860, 203.7984951890123000, 39.35113791807857098 ) ) ;
#851=CARTESIAN_POINT ( 'NONE',  ( -3.662846001189865142, 195.5725841191952838, 4.898862081921434353 ) ) ;
#852=CARTESIAN_POINT ( 'NONE',  ( -3.044812012439970683, 197.4746971517856196, 10.89886208192143613 ) ) ;
#855=CARTESIAN_POINT ( 'NONE',  ( 0.05014649552807549926, 219.6175466908591716, 49.25113791807856956 ) ) ;
#857=CARTESIAN_POINT ( 'NONE',  ( -8.062137200540822946, 201.0835637161416400, 17.19886208192143684 ) ) ;
#860=VERTEX_POINT ( 'NONE', #29951 ) ;
#861=CARTESIAN_POINT ( 'NONE',  ( -9.984503880673473830, 210.2968891136704315, 84.65113791807857524 ) ) ;
#867=CARTESIAN_POINT ( 'NONE',  ( 4.903702542908601636, 200.1653181626581102, 23.45113791807856884 ) ) ;
#869=CARTESIAN_POINT ( 'NONE',  ( -9.984503880673420539, 203.7031108863293980, 2.348862081921433198 ) ) ;
#871=ORIENTED_EDGE ( 'NONE', *, *, #13443, .T. ) ;
#876=CARTESIAN_POINT ( 'NONE',  ( -8.062137200540822946, 201.0835637161416400, 86.19886208192144750 ) ) ;
#878=CARTESIAN_POINT ( 'NONE',  ( 6.139770520408368348, 198.4640165459539674, 26.45113791807856884 ) ) ;
#880=CARTESIAN_POINT ( 'NONE',  ( -7.456977232089471386, 217.1783343296987709, 77.94886208192143329 ) ) ;
#884=CARTESIAN_POINT ( 'NONE',  ( 6.220909254589536808, 215.4770327129947702, 91.55113791807858092 ) ) ;
#887=CARTESIAN_POINT ( 'NONE',  ( -3.135527875058821579, 197.5041725223112223, 32.90113791807857524 ) ) ;
#892=CARTESIAN_POINT ( 'NONE',  ( -12.01549611932652972, 203.1486557965464499, 24.35113791807856742 ) ) ;
#896=CARTESIAN_POINT ( 'NONE',  ( -12.01549611932659722, 210.8513442034533227, 29.64886208192143968 ) ) ;
#898=CARTESIAN_POINT ( 'NONE',  ( -8.062137200540920645, 212.9164362838581894, 48.80113791807857382 ) ) ;
#900=CARTESIAN_POINT ( 'NONE',  ( 4.903702542908435547, 213.8346818373419751, 12.54886208192143826 ) ) ;
#906=CARTESIAN_POINT ( 'NONE',  ( 0.05014649552828262524, 198.5883022060938572, 103.7488620819214304 ) ) ;
#907=CARTESIAN_POINT ( 'NONE',  ( -0.05014649552807731031, 198.5883022060938572, 38.75113791807856956 ) ) ;
#912=CARTESIAN_POINT ( 'NONE',  ( 9.984503880673420539, 210.2968891136705167, 63.84886208192142476 ) ) ;
#915=CARTESIAN_POINT ( 'NONE',  ( -6.500168698208129925, 202.3363017425936050, 102.2011379180785866 ) ) ;
#918=CARTESIAN_POINT ( 'NONE',  ( 6.500168698208244500, 202.3363017425938324, 73.29886208192142760 ) ) ;
#919=DIRECTION ( 'NONE',  ( 0.000000000000000000, 0.9949972439410068592, -0.09990237509589369735 ) ) ;
#923=CARTESIAN_POINT ( 'NONE',  ( 10.01549611932653860, 210.2015048109876716, 7.851137918078565647 ) ) ;
#924=ORIENTED_EDGE ( 'NONE', *, *, #32237, .F. ) ;
#928=CARTESIAN_POINT ( 'NONE',  ( -12.00000000000000711, 207.0476921513413515, 75.50113791807856956 ) ) ;
#929=CARTESIAN_POINT ( 'NONE',  ( 8.118202686958039038, 212.8392687619912635, 97.70113791807857240 ) ) ;
#932=CARTESIAN_POINT ( 'NONE',  ( -6.220909254589682469, 215.4770327129946850, 2.948862081921434175 ) ) ;
#933=CARTESIAN_POINT ( 'NONE',  ( -9.680171189290716072, 199.9079932115567146, 59.19886208192144750 ) ) ;
#934=CARTESIAN_POINT ( 'NONE',  ( 0.05014649552828275014, 196.4853777576173002, 70.74886208192143044 ) ) ;
#935=CARTESIAN_POINT ( 'NONE',  ( 9.680171189290716072, 214.0920067884432854, 6.698862081921434175 ) ) ;
#937=CARTESIAN_POINT ( 'NONE',  ( -6.220909254589537696, 198.5229672870051161, 27.05113791807856671 ) ) ;
#938=CARTESIAN_POINT ( 'NONE',  ( 9.984503880673420539, 210.2968891136705167, 90.84886208192143897 ) ) ;
#943=CARTESIAN_POINT ( 'NONE',  ( -2.517493886309087880, 214.5937144450984135, 72.09886208192142476 ) ) ;
#953=CARTESIAN_POINT ( 'NONE',  ( -8.015496119326531499, 204.4483345814780364, 69.35113791807857808 ) ) ;
#956=DIRECTION ( 'NONE',  ( 1.000000000000000000, 2.912190848224676732E-17, -6.099278249758083281E-16 ) ) ;
#958=CARTESIAN_POINT ( 'NONE',  ( -6.500168698208244500, 211.6636982574061676, 41.79886208192144181 ) ) ;
#959=CARTESIAN_POINT ( 'NONE',  ( 10.01549611932653860, 210.2015048109876716, 76.85113791807857808 ) ) ;
#960=CARTESIAN_POINT ( 'NONE',  ( -8.118202686958039038, 201.1607312380087080, 69.20113791807858661 ) ) ;
#962=CARTESIAN_POINT ( 'NONE',  ( 2.426778023690261410, 199.3768101843759837, 20.60113791807856742 ) ) ;
#966=CARTESIAN_POINT ( 'NONE',  ( 11.98450388067348271, 203.0532714938637753, 47.15113791807857524 ) ) ;
#969=CARTESIAN_POINT ( 'NONE',  ( 3.044812012440130555, 197.4746971517856764, 92.60113791807857808 ) ) ;
#970=CARTESIAN_POINT ( 'NONE',  ( -10.01549611932653860, 203.7984951890123000, 72.35113791807857808 ) ) ;
#973=CARTESIAN_POINT ( 'NONE',  ( -3.662846001189865142, 195.5725841191952838, 31.89886208192143613 ) ) ;
#974=CARTESIAN_POINT ( 'NONE',  ( 8.062137200540822946, 212.9164362838583315, 39.69886208192143329 ) ) ;
#976=CARTESIAN_POINT ( 'NONE',  ( -11.98450388067348804, 210.9467285061362247, 81.65113791807856103 ) ) ;
#977=CARTESIAN_POINT ( 'NONE',  ( 7.984503880673485376, 204.3529502787953902, 101.1511379180785895 ) ) ;
#979=CARTESIAN_POINT ( 'NONE',  ( 9.984503880673420539, 210.2968891136705167, 57.84886208192143897 ) ) ;
#983=CARTESIAN_POINT ( 'NONE',  ( 3.662846001189864698, 218.4274158808046593, 57.39886208192143613 ) ) ;
#986=CARTESIAN_POINT ( 'NONE',  ( 7.984503880673422316, 209.6470497212048372, 36.84886208192142476 ) ) ;
#992=CARTESIAN_POINT ( 'NONE',  ( -2.517493886308901807, 199.4062855549015012, 50.90113791807858235 ) ) ;
#996=CARTESIAN_POINT ( 'NONE',  ( 10.01549611932659545, 203.7984951890123853, 37.14886208192142192 ) ) ;
#1004=CARTESIAN_POINT ( 'NONE',  ( 7.984503880673422316, 209.6470497212048372, 18.84886208192143187 ) ) ;
#1005=CARTESIAN_POINT ( 'NONE',  ( -6.139770520408369237, 215.5359834540460042, 54.95113791807856529 ) ) ;
#1006=CARTESIAN_POINT ( 'NONE',  ( 3.044812012440130555, 197.4746971517856764, 41.60113791807857808 ) ) ;
#1009=CARTESIAN_POINT ( 'NONE',  ( -4.984841277089891776, 213.7757310962905990, 98.94886208192143329 ) ) ;
#1013=CARTESIAN_POINT ( 'NONE',  ( -11.98450388067348804, 210.9467285061362247, 21.65113791807856813 ) ) ;
#1016=CARTESIAN_POINT ( 'NONE',  ( -3.135527875058821579, 197.5041725223112223, 68.90113791807857524 ) ) ;
#1018=CARTESIAN_POINT ( 'NONE',  ( 3.044812012440130555, 197.4746971517856764, 41.60113791807857808 ) ) ;
#1021=CARTESIAN_POINT ( 'NONE',  ( -3.753561863808878130, 218.3979405102790281, 6.098862081921433642 ) ) ;
#1022=CARTESIAN_POINT ( 'NONE',  ( -10.00000000000000711, 206.9523078486584495, 11.49886208192143577 ) ) ;
#1025=CARTESIAN_POINT ( 'NONE',  ( -3.662846001190052991, 218.4274158808045740, 46.10113791807857098 ) ) ;
#1027=CARTESIAN_POINT ( 'NONE',  ( 8.015496119326531499, 209.5516654185219636, 67.85113791807857808 ) ) ;
#1030=CARTESIAN_POINT ( 'NONE',  ( 8.118202686958138514, 201.1607312380088501, 28.29886208192143471 ) ) ;
#1034=CARTESIAN_POINT ( 'NONE',  ( -10.01549611932653860, 203.7984951890123284, 78.35113791807857808 ) ) ;
#1040=CARTESIAN_POINT ( 'NONE',  ( 4.984841277089725686, 213.7757310962907411, 19.55113791807856671 ) ) ;
#1042=CARTESIAN_POINT ( 'NONE',  ( 8.118202686958138514, 201.1607312380088501, 4.298862081921434708 ) ) ;
#1050=CARTESIAN_POINT ( 'NONE',  ( -6.220909254589682469, 215.4770327129946850, 92.94886208192143329 ) ) ;
#1052=CARTESIAN_POINT ( 'NONE',  ( -3.044812012440131443, 216.5253028482142952, 19.10113791807856742 ) ) ;
#1056=CARTESIAN_POINT ( 'NONE',  ( -12.01549611932659722, 210.8513442034533227, 77.64886208192143613 ) ) ;
#1060=CARTESIAN_POINT ( 'NONE',  ( -8.062137200540920645, 212.9164362838581894, 96.80113791807858092 ) ) ;
#1064=CARTESIAN_POINT ( 'NONE',  ( -8.118202686958039038, 201.1607312380087080, 39.20113791807857240 ) ) ;
#1069=CARTESIAN_POINT ( 'NONE',  ( 0.05014649552807549926, 219.6175466908591716, 16.25113791807856600 ) ) ;
#1074=CARTESIAN_POINT ( 'NONE',  ( 9.680171189290716072, 214.0920067884432854, 33.69886208192142618 ) ) ;
#1077=CARTESIAN_POINT ( 'NONE',  ( -8.118202686958039038, 201.1607312380087080, 54.20113791807857240 ) ) ;
#1079=CARTESIAN_POINT ( 'NONE',  ( 7.984503880673422316, 209.6470497212048372, 15.84886208192143719 ) ) ;
#1082=CARTESIAN_POINT ( 'NONE',  ( 8.000000000000008882, 207.0476921513415220, 102.9988620819214304 ) ) ;
#1083=CARTESIAN_POINT ( 'NONE',  ( 0.05014649552807626948, 215.4116977939061144, 43.25113791807856956 ) ) ;
#1088=CARTESIAN_POINT ( 'NONE',  ( -3.135527875058982783, 216.4958274776886924, 63.09886208192143187 ) ) ;
#1091=CARTESIAN_POINT ( 'NONE',  ( 2.426778023690261410, 199.3768101843759837, 98.60113791807857808 ) ) ;
#1095=CARTESIAN_POINT ( 'NONE',  ( -8.000000000000008882, 206.9523078486584780, 74.49886208192144466 ) ) ;
#1097=CARTESIAN_POINT ( 'NONE',  ( -0.3755270751584372513, 206.7692714347155629, 108.3323677711371573 ) ) ;
#1099=CARTESIAN_POINT ( 'NONE',  ( -6.220909254589537696, 198.5229672870051445, 9.051137918078566713 ) ) ;
#1103=CARTESIAN_POINT ( 'NONE',  ( 12.00000000000000711, 206.9523078486586485, 77.00113791807858377 ) ) ;
#1104=CARTESIAN_POINT ( 'NONE',  ( 6.220909254589536808, 215.4770327129947987, 94.55113791807858092 ) ) ;
#1107=CARTESIAN_POINT ( 'NONE',  ( 9.680171189290716072, 214.0920067884432854, 102.6988620819214475 ) ) ;
#1108=CARTESIAN_POINT ( 'NONE',  ( 0.05014649552828288198, 194.3824533091408000, 61.74886208192143755 ) ) ;
#1109=CARTESIAN_POINT ( 'NONE',  ( -6.220909254589682469, 215.4770327129947134, 68.94886208192143329 ) ) ;
#1110=CARTESIAN_POINT ( 'NONE',  ( 12.00000000000000711, 207.0476921513415220, 6.998862081921433997 ) ) ;
#1112=CARTESIAN_POINT ( 'NONE',  ( -8.062137200540920645, 212.9164362838581894, 27.80113791807856671 ) ) ;
#1113=CARTESIAN_POINT ( 'NONE',  ( 8.062137200540822946, 212.9164362838583315, 87.69886208192144750 ) ) ;
#1118=CARTESIAN_POINT ( 'NONE',  ( -4.903702542908436435, 200.1653181626580249, 74.04886208192142760 ) ) ;
#1125=CARTESIAN_POINT ( 'NONE',  ( -6.500168698208129925, 202.3363017425936050, 69.20113791807857240 ) ) ;
#1128=CARTESIAN_POINT ( 'NONE',  ( 8.000000000000008882, 207.0476921513415220, 42.99886208192143755 ) ) ;
#1129=CARTESIAN_POINT ( 'NONE',  ( 0.05014649552810505201, 217.5146222423826714, 91.25113791807858377 ) ) ;
#1130=CARTESIAN_POINT ( 'NONE',  ( -10.01549611932653860, 203.7984951890123284, 69.35113791807857808 ) ) ;
#1132=CARTESIAN_POINT ( 'NONE',  ( -8.015496119326531499, 204.4483345814780364, 24.35113791807856742 ) ) ;
#1136=CARTESIAN_POINT ( 'NONE',  ( -3.662846001190052991, 218.4274158808045740, 49.10113791807857808 ) ) ;
#1138=CARTESIAN_POINT ( 'NONE',  ( 3.135527875058820690, 216.4958274776887492, 94.40113791807857524 ) ) ;
#1140=CARTESIAN_POINT ( 'NONE',  ( 8.062137200540920645, 201.0835637161417822, 65.30113791807858092 ) ) ;
#1141=CARTESIAN_POINT ( 'NONE',  ( 7.456977232089471386, 196.8216656703012006, 28.44886208192142973 ) ) ;
#1142=CARTESIAN_POINT ( 'NONE',  ( 0.05014649552828275014, 196.4853777576173002, 37.74886208192144466 ) ) ;
#1144=CARTESIAN_POINT ( 'NONE',  ( -3.662846001190052991, 218.4274158808045740, 82.10113791807857808 ) ) ;
#1145=CARTESIAN_POINT ( 'NONE',  ( 6.444103211791042618, 202.2591342207267644, 98.30113791807858092 ) ) ;
#1146=CARTESIAN_POINT ( 'NONE',  ( -8.062137200540822946, 201.0835637161416400, 62.19886208192143329 ) ) ;
#1149=CARTESIAN_POINT ( 'NONE',  ( 9.736236675708031640, 199.9851607334238963, 64.29886208192144181 ) ) ;
#1153=CARTESIAN_POINT ( 'NONE',  ( -7.984503880673422316, 204.3529502787951628, 41.34886208192143897 ) ) ;
#1158=CARTESIAN_POINT ( 'NONE',  ( -8.000000000000008882, 207.0476921513413515, 54.50113791807857666 ) ) ;
#1159=CARTESIAN_POINT ( 'NONE',  ( 10.00000000000000711, 207.0476921513415220, 33.99886208192143044 ) ) ;
#1165=CARTESIAN_POINT ( 'NONE',  ( 8.015496119326595448, 204.4483345814782638, 16.14886208192143968 ) ) ;
#1166=CARTESIAN_POINT ( 'NONE',  ( 8.062137200540920645, 201.0835637161417822, 59.30113791807857382 ) ) ;
#1167=CARTESIAN_POINT ( 'NONE',  ( -9.984503880673473830, 210.2968891136704315, 39.65113791807857524 ) ) ;
#1170=CARTESIAN_POINT ( 'NONE',  ( 2.517493886309087436, 199.4062855549015865, 103.5988620819214532 ) ) ;
#1173=CARTESIAN_POINT ( 'NONE',  ( 7.375838497908181246, 196.7627149292499666, 23.45113791807856884 ) ) ;
#1175=CARTESIAN_POINT ( 'NONE',  ( 0.05014649552810505201, 217.5146222423826714, 67.25113791807856956 ) ) ;
#1177=CARTESIAN_POINT ( 'NONE',  ( 9.984503880673473830, 203.7031108863295401, 44.15113791807856813 ) ) ;
#1180=CARTESIAN_POINT ( 'NONE',  ( 7.456977232089471386, 196.8216656703012006, 7.448862081921435951 ) ) ;
#1181=CARTESIAN_POINT ( 'NONE',  ( -3.135527875058982783, 216.4958274776886924, 12.09886208192143542 ) ) ;
#1184=CARTESIAN_POINT ( 'NONE',  ( -12.01549611932652972, 203.1486557965464499, 51.35113791807857098 ) ) ;
#1185=CARTESIAN_POINT ( 'NONE',  ( -4.984841277089726574, 200.2242689037092305, 66.05113791807858092 ) ) ;
#1187=CARTESIAN_POINT ( 'NONE',  ( 6.220909254589681581, 198.5229672870052582, 28.44886208192143684 ) ) ;
#1190=CARTESIAN_POINT ( 'NONE',  ( -10.01549611932653860, 203.7984951890123284, 81.35113791807857808 ) ) ;
#1193=DIRECTION ( 'NONE',  ( 5.620504062164857944E-16, -0.9988620819214347746, 0.04769215134146256169 ) ) ;
#1194=EDGE_LOOP ( 'NONE', ( #3412, #16477, #22110, #1374, #13596 ) ) ;
#1195=CARTESIAN_POINT ( 'NONE',  ( 2.426778023690261410, 199.3768101843759837, 26.60113791807856742 ) ) ;
#1198=CARTESIAN_POINT ( 'NONE',  ( 10.01549611932659545, 203.7984951890123853, 4.148862081921434353 ) ) ;
#1202=CARTESIAN_POINT ( 'NONE',  ( 6.444103211791042618, 202.2591342207267644, 47.30113791807858092 ) ) ;
#1207=CARTESIAN_POINT ( 'NONE',  ( 8.062137200540822946, 212.9164362838583315, 90.69886208192143329 ) ) ;
#1211=CARTESIAN_POINT ( 'NONE',  ( 8.118202686958039038, 212.8392687619912635, 19.70113791807856884 ) ) ;
#1213=CARTESIAN_POINT ( 'NONE',  ( 3.753561863808876797, 195.6020594897209719, 82.59886208192143897 ) ) ;
#1217=CARTESIAN_POINT ( 'NONE',  ( 0.05014649552810505201, 217.5146222423826714, 97.25113791807854113 ) ) ;
#1220=CARTESIAN_POINT ( 'NONE',  ( 9.984503880673470277, 203.7031108863295401, 35.15113791807856813 ) ) ;
#1228=CARTESIAN_POINT ( 'NONE',  ( -9.736236675707914401, 199.9851607334237542, 21.20113791807856529 ) ) ;
#1233=CARTESIAN_POINT ( 'NONE',  ( -7.375838497908014268, 196.7627149292498530, 47.04886208192144181 ) ) ;
#1235=CARTESIAN_POINT ( 'NONE',  ( 9.984503880673470277, 203.7031108863295401, 50.15113791807855392 ) ) ;
#1237=CARTESIAN_POINT ( 'NONE',  ( -8.015496119326597224, 209.5516654185217362, 14.64886208192143258 ) ) ;
#1243=CARTESIAN_POINT ( 'NONE',  ( 2.426778023690075337, 214.6231898156240447, 96.39886208192146455 ) ) ;
#1246=CARTESIAN_POINT ( 'NONE',  ( 2.426778023690261410, 199.3768101843759837, 44.60113791807857098 ) ) ;
#1252=CARTESIAN_POINT ( 'NONE',  ( 10.01549611932659545, 203.7984951890123853, 61.14886208192144323 ) ) ;
#1253=ADVANCED_FACE ( 'NONE', ( #13725 ), #13394, .T. ) ;
#1256=CARTESIAN_POINT ( 'NONE',  ( -8.015496119326531499, 204.4483345814780364, 99.35113791807857808 ) ) ;
#1261=CARTESIAN_POINT ( 'NONE',  ( 8.000000000000008882, 207.0476921513415220, 81.99886208192144466 ) ) ;
#1267=CARTESIAN_POINT ( 'NONE',  ( 10.00000000000000711, 206.9523078486586201, 20.00113791807856600 ) ) ;
#1271=CARTESIAN_POINT ( 'NONE',  ( -9.680171189290831535, 214.0920067884431148, 84.80113791807858092 ) ) ;
#1275=CARTESIAN_POINT ( 'NONE',  ( 3.753561863808876797, 195.6020594897209719, 58.59886208192143897 ) ) ;
#1277=CARTESIAN_POINT ( 'NONE',  ( -6.220909254589682469, 215.4770327129947134, 71.94886208192144750 ) ) ;
#1278=CARTESIAN_POINT ( 'NONE',  ( -12.01549611932659722, 210.8513442034533227, 11.64886208192143613 ) ) ;
#1280=CARTESIAN_POINT ( 'NONE',  ( -10.00000000000000711, 207.0476921513413515, 21.50113791807856956 ) ) ;
#1281=CARTESIAN_POINT ( 'NONE',  ( 9.984503880673420539, 210.2968891136705167, 87.84886208192141055 ) ) ;
#1284=LINE ( 'NONE', #32113, #20847 ) ;
#1288=CARTESIAN_POINT ( 'NONE',  ( -8.000000000000008882, 206.9523078486584780, 71.49886208192144466 ) ) ;
#1296=MANIFOLD_SOLID_BREP ( 'Fillet2', #22105 ) ;
#1299=CARTESIAN_POINT ( 'NONE',  ( -2.517493886308901807, 199.4062855549015012, 65.90113791807856103 ) ) ;
#1304=CARTESIAN_POINT ( 'NONE',  ( -7.984503880673422316, 204.3529502787951628, 44.34886208192144608 ) ) ;
#1305=CARTESIAN_POINT ( 'NONE',  ( -0.05014649552810635652, 196.4853777576173002, 74.75113791807858377 ) ) ;
#1311=CARTESIAN_POINT ( 'NONE',  ( 12.00000000000000711, 206.9523078486586485, 53.00113791807857666 ) ) ;
#1314=CARTESIAN_POINT ( 'NONE',  ( -6.139770520408369237, 215.5359834540460042, 99.95113791807855819 ) ) ;
#1315=CARTESIAN_POINT ( 'NONE',  ( 9.984503880673473830, 203.7031108863295401, 65.15113791807856103 ) ) ;
#1316=CARTESIAN_POINT ( 'NONE',  ( -12.00000000000000711, 206.9523078486584780, 32.49886208192143044 ) ) ;
#1317=CARTESIAN_POINT ( 'NONE',  ( 3.044812012439969795, 216.5253028482143520, 51.39886208192143613 ) ) ;
#1319=CARTESIAN_POINT ( 'NONE',  ( -0.05014649552807705357, 194.3824533091408000, 80.75113791807856956 ) ) ;
#1320=CARTESIAN_POINT ( 'NONE',  ( -0.05014649552807731031, 198.5883022060938572, 95.75113791807856956 ) ) ;
#1321=CARTESIAN_POINT ( 'NONE',  ( 8.118202686958138514, 201.1607312380088501, 61.29886208192143471 ) ) ;
#1324=CARTESIAN_POINT ( 'NONE',  ( 7.456977232089471386, 196.8216656703012006, 61.44886208192143329 ) ) ;
#1325=EDGE_LOOP ( 'NONE', ( #5593, #15241, #7416, #14552 ) ) ;
#1327=CARTESIAN_POINT ( 'NONE',  ( 8.015496119326595448, 204.4483345814782638, 46.14886208192143613 ) ) ;
#1332=CARTESIAN_POINT ( 'NONE',  ( -2.426778023690262742, 214.6231898156240163, 49.10113791807857808 ) ) ;
#1335=CARTESIAN_POINT ( 'NONE',  ( 9.984503880673420539, 210.2968891136705167, 30.84886208192142831 ) ) ;
#1341=CARTESIAN_POINT ( 'NONE',  ( 6.500168698208244500, 202.3363017425938324, 16.29886208192143471 ) ) ;
#1342=CARTESIAN_POINT ( 'NONE',  ( 9.984503880673470277, 203.7031108863295401, 62.15113791807856813 ) ) ;
#1343=CARTESIAN_POINT ( 'NONE',  ( -6.220909254589537696, 198.5229672870051161, 51.05113791807856671 ) ) ;
#1345=CARTESIAN_POINT ( 'NONE',  ( -0.05014649552828365914, 215.4116977939061144, 99.24886208192143044 ) ) ;
#1349=CARTESIAN_POINT ( 'NONE',  ( -0.05014649552807705357, 194.3824533091408000, 20.75113791807856600 ) ) ;
#1351=CARTESIAN_POINT ( 'NONE',  ( 3.044812012440130555, 197.4746971517856764, 62.60113791807857098 ) ) ;
#1352=CARTESIAN_POINT ( 'NONE',  ( -8.118202686958039038, 201.1607312380087080, 39.20113791807857240 ) ) ;
#1354=CARTESIAN_POINT ( 'NONE',  ( -12.00000000000000711, 206.9523078486584780, 8.498862081921435774 ) ) ;
#1355=CARTESIAN_POINT ( 'NONE',  ( 8.118202686958138514, 201.1607312380088501, 13.29886208192143648 ) ) ;
#1358=CARTESIAN_POINT ( 'NONE',  ( 3.662846001190051659, 195.5725841191953691, 50.60113791807857808 ) ) ;
#1359=CARTESIAN_POINT ( 'NONE',  ( -2.426778023690262742, 214.6231898156240163, 73.10113791807857808 ) ) ;
#1361=CARTESIAN_POINT ( 'NONE',  ( -10.00000000000000711, 206.9523078486584495, 29.49886208192143400 ) ) ;
#1364=CARTESIAN_POINT ( 'NONE',  ( 9.984503880673470277, 203.7031108863295401, 89.15113791807857524 ) ) ;
#1369=CARTESIAN_POINT ( 'NONE',  ( -2.517493886308901807, 199.4062855549015012, 26.90113791807856813 ) ) ;
#1372=CARTESIAN_POINT ( 'NONE',  ( 0.05014649552828275708, 196.4853777576173002, 1.748862081921434219 ) ) ;
#1374=ORIENTED_EDGE ( 'NONE', *, *, #24292, .T. ) ;
#1375=CARTESIAN_POINT ( 'NONE',  ( 7.984503880673485376, 204.3529502787953902, 47.15113791807857524 ) ) ;
#1378=CARTESIAN_POINT ( 'NONE',  ( -8.062137200540822946, 201.0835637161416400, 95.19886208192143329 ) ) ;
#1380=CARTESIAN_POINT ( 'NONE',  ( -9.984503880673473830, 210.2968891136704315, 27.65113791807855748 ) ) ;
#1382=CARTESIAN_POINT ( 'NONE',  ( -3.662846001189865142, 195.5725841191952838, 82.89886208192143613 ) ) ;
#1387=CARTESIAN_POINT ( 'NONE',  ( -4.945910536743085117, 206.2642604888503968, -6.000000000000014211 ) ) ;
#1388=CARTESIAN_POINT ( 'NONE',  ( -6.139770520408369237, 215.5359834540460042, 93.95113791807854398 ) ) ;
#1391=CARTESIAN_POINT ( 'NONE',  ( 3.044812012440130555, 197.4746971517856764, 38.60113791807857098 ) ) ;
#1399=CARTESIAN_POINT ( 'NONE',  ( 12.00000000000000711, 206.9523078486586485, 20.00113791807856956 ) ) ;
#1403=CARTESIAN_POINT ( 'NONE',  ( -9.736236675708031640, 214.0148392665760753, 41.79886208192143471 ) ) ;
#1404=CARTESIAN_POINT ( 'NONE',  ( -8.118202686958039038, 201.1607312380087080, 6.201137918078566180 ) ) ;
#1405=CARTESIAN_POINT ( 'NONE',  ( -0.05014649552810635652, 196.4853777576173002, 59.75113791807857666 ) ) ;
#1407=CARTESIAN_POINT ( 'NONE',  ( -8.000000000000008882, 206.9523078486584780, 17.49886208192143400 ) ) ;
#1410=CARTESIAN_POINT ( 'NONE',  ( -6.500168698208244500, 211.6636982574061676, 95.79886208192144181 ) ) ;
#1413=CARTESIAN_POINT ( 'NONE',  ( -7.984503880673488041, 209.6470497212046098, 39.65113791807857524 ) ) ;
#1418=CARTESIAN_POINT ( 'NONE',  ( 9.984503880673470277, 203.7031108863295401, -0.8488620819214341973 ) ) ;
#1419=CARTESIAN_POINT ( 'NONE',  ( -3.135527875058982783, 216.4958274776886924, 66.09886208192143897 ) ) ;
#1422=CARTESIAN_POINT ( 'NONE',  ( -9.984503880673473830, 210.2968891136704315, 6.651137918078564581 ) ) ;
#1426=CARTESIAN_POINT ( 'NONE',  ( 6.500168698208244500, 202.3363017425938324, 85.29886208192145602 ) ) ;
#1430=CARTESIAN_POINT ( 'NONE',  ( -3.044812012440131443, 216.5253028482142952, 19.10113791807856742 ) ) ;
#1434=CARTESIAN_POINT ( 'NONE',  ( -11.98450388067348804, 210.9467285061362247, 84.65113791807856103 ) ) ;
#1440=CARTESIAN_POINT ( 'NONE',  ( 7.375838497908012492, 217.2372850707501186, 69.54886208192141339 ) ) ;
#1441=CARTESIAN_POINT ( 'NONE',  ( -3.044812012439970683, 197.4746971517856196, 79.89886208192143613 ) ) ;
#1442=CARTESIAN_POINT ( 'NONE',  ( 11.98450388067341876, 210.9467285061363953, 12.84886208192143719 ) ) ;
#1444=CARTESIAN_POINT ( 'NONE',  ( 6.220909254589536808, 215.4770327129947702, 25.55113791807856671 ) ) ;
#1447=CARTESIAN_POINT ( 'NONE',  ( -8.118202686958138514, 212.8392687619910930, 89.79886208192144181 ) ) ;
#1452=CARTESIAN_POINT ( 'NONE',  ( 4.984841277089891776, 200.2242689037093726, 67.44886208192143329 ) ) ;
#1459=CARTESIAN_POINT ( 'NONE',  ( 7.984503880673485376, 204.3529502787953902, 80.15113791807857524 ) ) ;
#1463=CARTESIAN_POINT ( 'NONE',  ( 6.500168698208244500, 202.3363017425938324, 52.29886208192144892 ) ) ;
#1472=CARTESIAN_POINT ( 'NONE',  ( 7.375838497908181246, 196.7627149292499666, 56.45113791807857240 ) ) ;
#1475=CARTESIAN_POINT ( 'NONE',  ( 11.98450388067348271, 203.0532714938637753, 2.151137918078565914 ) ) ;
#1477=CARTESIAN_POINT ( 'NONE',  ( -6.139770520408368348, 215.5359834540460042, 78.95113791807857240 ) ) ;
#1478=CARTESIAN_POINT ( 'NONE',  ( -7.456977232089471386, 217.1783343296987709, 38.94886208192143329 ) ) ;
#1479=CARTESIAN_POINT ( 'NONE',  ( 6.139770520408223575, 215.5359834540460611, 48.54886208192143471 ) ) ;
#1481=CARTESIAN_POINT ( 'NONE',  ( 12.00000000000000711, 206.9523078486586485, 89.00113791807858377 ) ) ;
#1483=CARTESIAN_POINT ( 'NONE',  ( -6.444103211791042618, 211.7408657792732356, 93.80113791807858092 ) ) ;
#1484=CARTESIAN_POINT ( 'NONE',  ( -3.135527875058982783, 216.4958274776886924, 63.09886208192143187 ) ) ;
#1488=CARTESIAN_POINT ( 'NONE',  ( -0.05014649552828442242, 219.6175466908591716, 69.24886208192143044 ) ) ;
#1491=CARTESIAN_POINT ( 'NONE',  ( 4.903702542908435547, 213.8346818373419751, 42.54886208192144181 ) ) ;
#1496=CARTESIAN_POINT ( 'NONE',  ( -9.207158067219113562, 207.6631797465213651, 102.8962158735644579 ) ) ;
#1497=CARTESIAN_POINT ( 'NONE',  ( 8.000000000000008882, 206.9523078486586485, 62.00113791807856956 ) ) ;
#1499=CARTESIAN_POINT ( 'NONE',  ( -8.062137200540822946, 201.0835637161416400, 47.19886208192143329 ) ) ;
#1504=CARTESIAN_POINT ( 'NONE',  ( -6.500168698208244500, 211.6636982574061676, 26.79886208192143826 ) ) ;
#1505=CARTESIAN_POINT ( 'NONE',  ( 3.044812012440130555, 197.4746971517856764, 62.60113791807857098 ) ) ;
#1506=CARTESIAN_POINT ( 'NONE',  ( 3.044812012440130555, 197.4746971517856764, 44.60113791807857098 ) ) ;
#1510=CARTESIAN_POINT ( 'NONE',  ( -10.00000000000000711, 207.0476921513413515, 18.50113791807856956 ) ) ;
#1511=CARTESIAN_POINT ( 'NONE',  ( 7.984503880673422316, 209.6470497212048372, 99.84886208192143897 ) ) ;
#1514=CARTESIAN_POINT ( 'NONE',  ( -9.680171189290831535, 214.0920067884431148, 24.80113791807857027 ) ) ;
#1516=CARTESIAN_POINT ( 'NONE',  ( -3.044812012440131443, 216.5253028482142952, 76.10113791807856387 ) ) ;
#1517=CARTESIAN_POINT ( 'NONE',  ( -9.984503880673475606, 210.2968891136704315, 48.65113791807857524 ) ) ;
#1521=CARTESIAN_POINT ( 'NONE',  ( 7.456977232089471386, 196.8216656703012006, 1.448862081921433953 ) ) ;
#1522=CARTESIAN_POINT ( 'NONE',  ( -8.118202686958138514, 212.8392687619910930, 23.79886208192143471 ) ) ;
#1525=CARTESIAN_POINT ( 'NONE',  ( -7.375838497908182134, 217.2372850707499765, 57.95113791807855819 ) ) ;
#1526=CARTESIAN_POINT ( 'NONE',  ( -2.517493886308901807, 199.4062855549015012, 68.90113791807856103 ) ) ;
#1527=CARTESIAN_POINT ( 'NONE',  ( 3.135527875058981895, 197.5041725223112792, 28.59886208192143897 ) ) ;
#1529=CARTESIAN_POINT ( 'NONE',  ( -10.00000000000000711, 207.0476921513413515, 90.50113791807858377 ) ) ;
#1537=CARTESIAN_POINT ( 'NONE',  ( -6.444103211791042618, 211.7408657792732356, 30.80113791807857027 ) ) ;
#1539=CARTESIAN_POINT ( 'NONE',  ( 6.139770520408223575, 215.5359834540460611, 12.54886208192143648 ) ) ;
#1543=CARTESIAN_POINT ( 'NONE',  ( -7.984503880673488041, 209.6470497212046098, 45.65113791807857524 ) ) ;
#1546=CARTESIAN_POINT ( 'NONE',  ( 8.118202686958138514, 201.1607312380088501, 88.29886208192142760 ) ) ;
#1548=CARTESIAN_POINT ( 'NONE',  ( 6.139770520408368348, 198.4640165459539674, 29.45113791807856529 ) ) ;
#1549=CARTESIAN_POINT ( 'NONE',  ( -11.00000000000000178, 206.7692714347155629, 108.3323677711372000 ) ) ;
#1550=CARTESIAN_POINT ( 'NONE',  ( 3.135527875058820690, 216.4958274776887492, 19.40113791807856813 ) ) ;
#1555=CARTESIAN_POINT ( 'NONE',  ( -0.05014649552807705357, 194.3824533091408000, 2.751137918078565114 ) ) ;
#1559=CARTESIAN_POINT ( 'NONE',  ( -0.05014649552810635652, 196.4853777576173002, 44.75113791807858377 ) ) ;
#1567=CARTESIAN_POINT ( 'NONE',  ( -12.01549611932652972, 203.1486557965464499, 18.35113791807856387 ) ) ;
#1572=CARTESIAN_POINT ( 'NONE',  ( 11.98450388067341876, 210.9467285061363953, 42.84886208192143187 ) ) ;
#1573=CARTESIAN_POINT ( 'NONE',  ( 10.00000000000000711, 206.9523078486586201, 2.001137918078565558 ) ) ;
#1574=CARTESIAN_POINT ( 'NONE',  ( -3.044812012440131443, 216.5253028482142952, 64.10113791807857808 ) ) ;
#1575=CARTESIAN_POINT ( 'NONE',  ( 8.015496119326595448, 204.4483345814782638, 19.14886208192143968 ) ) ;
#1578=CARTESIAN_POINT ( 'NONE',  ( 4.984841277089891776, 200.2242689037093726, 100.4488620819214475 ) ) ;
#1581=CARTESIAN_POINT ( 'NONE',  ( 0.05014649552807626948, 215.4116977939061144, 40.25113791807856956 ) ) ;
#1586=CARTESIAN_POINT ( 'NONE',  ( -10.00000000000000711, 207.0476921513413515, 0.5011379180785656695 ) ) ;
#1588=CARTESIAN_POINT ( 'NONE',  ( -9.984503880673420539, 203.7031108863293980, 65.34886208192143897 ) ) ;
#1591=CARTESIAN_POINT ( 'NONE',  ( -8.118202686958039038, 201.1607312380087080, 3.201137918078566180 ) ) ;
#1596=CARTESIAN_POINT ( 'NONE',  ( 2.517493886309087436, 199.4062855549015865, 82.59886208192143897 ) ) ;
#1600=CARTESIAN_POINT ( 'NONE',  ( 10.01549611932653860, 210.2015048109876716, 16.85113791807856387 ) ) ;
#1604=CARTESIAN_POINT ( 'NONE',  ( 11.98450388067348271, 203.0532714938637753, 83.15113791807856103 ) ) ;
#1609=CARTESIAN_POINT ( 'NONE',  ( -11.98450388067341876, 203.0532714938636047, 74.34886208192142476 ) ) ;
#1610=CARTESIAN_POINT ( 'NONE',  ( -8.062137200540822946, 201.0835637161416400, 80.19886208192143329 ) ) ;
#1611=CARTESIAN_POINT ( 'NONE',  ( -12.01549611932659722, 210.8513442034533227, 17.64886208192143968 ) ) ;
#1613=CARTESIAN_POINT ( 'NONE',  ( 10.00000000000000711, 206.9523078486586201, 35.00113791807856956 ) ) ;
#1614=CARTESIAN_POINT ( 'NONE',  ( 9.984503880673420539, 210.2968891136705167, 93.84886208192143897 ) ) ;
#1619=CARTESIAN_POINT ( 'NONE',  ( -2.426778023690076225, 199.3768101843759553, 70.89886208192143613 ) ) ;
#1627=CARTESIAN_POINT ( 'NONE',  ( 8.015496119326531499, 209.5516654185219636, 79.85113791807857808 ) ) ;
#1630=CARTESIAN_POINT ( 'NONE',  ( 0.05014649552828262524, 198.5883022060938572, 55.74886208192144466 ) ) ;
#1637=CARTESIAN_POINT ( 'NONE',  ( 11.98450388067348271, 203.0532714938637753, 62.15113791807858945 ) ) ;
#1639=CARTESIAN_POINT ( 'NONE',  ( -0.05014649552807705357, 194.3824533091408000, -0.2488620819214344970 ) ) ;
#1641=CARTESIAN_POINT ( 'NONE',  ( -0.05014649552810635652, 196.4853777576173002, 80.75113791807855534 ) ) ;
#1642=CARTESIAN_POINT ( 'NONE',  ( -12.01549611932659722, 210.8513442034533227, 44.64886208192143613 ) ) ;
#1643=CARTESIAN_POINT ( 'NONE',  ( 0.05014649552828275014, 196.4853777576173002, 46.74886208192143755 ) ) ;
#1645=CARTESIAN_POINT ( 'NONE',  ( -12.00000000000000711, 207.0476921513413515, 84.50113791807856956 ) ) ;
#1646=CARTESIAN_POINT ( 'NONE',  ( -9.984503880673473830, 210.2968891136704315, 0.6511379180785656917 ) ) ;
#1647=CARTESIAN_POINT ( 'NONE',  ( 6.139770520408223575, 215.5359834540460611, 60.54886208192143471 ) ) ;
#1649=CARTESIAN_POINT ( 'NONE',  ( 9.680171189290716072, 214.0920067884432854, 69.69886208192143329 ) ) ;
#1652=CARTESIAN_POINT ( 'NONE',  ( -2.426778023690076225, 199.3768101843759553, 46.89886208192144323 ) ) ;
#1654=EDGE_CURVE ( 'NONE', #6694, #31012, #5880, .T. ) ;
#1659=CARTESIAN_POINT ( 'NONE',  ( 6.444103211791042618, 202.2591342207267644, 62.30113791807858092 ) ) ;
#1660=PRODUCT_DEFINITION ( 'UNKNOWN', '', #2328, #24753 ) ;
#1663=CARTESIAN_POINT ( 'NONE',  ( -0.05014649552828403384, 217.5146222423826714, 39.24886208192142334 ) ) ;
#1666=PRESENTATION_STYLE_ASSIGNMENT (( #4217 ) ) ;
#1669=CARTESIAN_POINT ( 'NONE',  ( -8.000000000000008882, 206.9523078486584780, 26.49886208192143400 ) ) ;
#1671=CARTESIAN_POINT ( 'NONE',  ( -3.135527875058821579, 197.5041725223112223, 56.90113791807857524 ) ) ;
#1672=CARTESIAN_POINT ( 'NONE',  ( -6.220909254589537696, 198.5229672870051161, 45.05113791807855961 ) ) ;
#1674=CARTESIAN_POINT ( 'NONE',  ( 10.00000000000000711, 206.9523078486586201, 17.00113791807856600 ) ) ;
#1675=CARTESIAN_POINT ( 'NONE',  ( 0.05014649552807626948, 215.4116977939061144, 10.25113791807856600 ) ) ;
#1679=CARTESIAN_POINT ( 'NONE',  ( 3.662846001190051659, 195.5725841191953691, 29.60113791807856742 ) ) ;
#1681=CARTESIAN_POINT ( 'NONE',  ( -8.062137200540920645, 212.9164362838581894, 72.80113791807856671 ) ) ;
#1682=CARTESIAN_POINT ( 'NONE',  ( 8.062137200540920645, 201.0835637161417822, 50.30113791807857382 ) ) ;
#1685=CARTESIAN_POINT ( 'NONE',  ( -0.05014649552828442242, 219.6175466908591716, 18.24886208192143755 ) ) ;
#1686=CARTESIAN_POINT ( 'NONE',  ( -9.984503880673420539, 203.7031108863293980, 17.34886208192143542 ) ) ;
#1689=CARTESIAN_POINT ( 'NONE',  ( 9.736236675707914401, 214.0148392665762458, 61.70113791807857240 ) ) ;
#1690=CARTESIAN_POINT ( 'NONE',  ( -2.426778023690262742, 214.6231898156240163, 67.10113791807857808 ) ) ;
#1691=CARTESIAN_POINT ( 'NONE',  ( -6.220909254589682469, 215.4770327129946850, 29.94886208192142973 ) ) ;
#1696=CARTESIAN_POINT ( 'NONE',  ( 6.220909254589536808, 215.4770327129947702, 91.55113791807858092 ) ) ;
#1701=CARTESIAN_POINT ( 'NONE',  ( -2.426778023690262742, 214.6231898156240163, 28.10113791807856742 ) ) ;
#1703=CARTESIAN_POINT ( 'NONE',  ( 10.00000000000000711, 207.0476921513415220, 15.99886208192143400 ) ) ;
#1706=CARTESIAN_POINT ( 'NONE',  ( -4.984841277089726574, 200.2242689037092305, 48.05113791807858092 ) ) ;
#1709=CARTESIAN_POINT ( 'NONE',  ( -8.118202686958138514, 212.8392687619910930, 95.79886208192144181 ) ) ;
#1711=CARTESIAN_POINT ( 'NONE',  ( 8.062137200540920645, 201.0835637161417822, 29.30113791807857027 ) ) ;
#1713=CARTESIAN_POINT ( 'NONE',  ( 6.139770520408368348, 198.4640165459539674, 20.45113791807855819 ) ) ;
#1718=CARTESIAN_POINT ( 'NONE',  ( -9.736236675707914401, 199.9851607334237542, 0.2011379180785655418 ) ) ;
#1721=CARTESIAN_POINT ( 'NONE',  ( -8.062137200540920645, 212.9164362838581894, 42.80113791807857382 ) ) ;
#1727=CARTESIAN_POINT ( 'NONE',  ( 12.01549611932652972, 210.8513442034534933, 28.85113791807856032 ) ) ;
#1729=CARTESIAN_POINT ( 'NONE',  ( -6.139770520408224463, 198.4640165459539389, 2.048862081921434264 ) ) ;
#1734=CARTESIAN_POINT ( 'NONE',  ( 0.05014649552810505201, 217.5146222423826714, 64.25113791807856956 ) ) ;
#1736=CARTESIAN_POINT ( 'NONE',  ( 0.05014649552828262524, 198.5883022060938572, 19.74886208192143400 ) ) ;
#1740=CARTESIAN_POINT ( 'NONE',  ( -7.984503880673488041, 209.6470497212046098, 0.6511379180785660248 ) ) ;
#1742=CARTESIAN_POINT ( 'NONE',  ( 7.375838497908012492, 217.2372850707501186, 87.54886208192142760 ) ) ;
#1747=CARTESIAN_POINT ( 'NONE',  ( 6.139770520408368348, 198.4640165459539674, -0.5488620819214343749 ) ) ;
#1748=CARTESIAN_POINT ( 'NONE',  ( -8.118202686958138514, 212.8392687619910930, 68.79886208192144181 ) ) ;
#1751=CARTESIAN_POINT ( 'NONE',  ( 0.05014649552810505201, 217.5146222423826714, 7.251137918078566003 ) ) ;
#1756=CARTESIAN_POINT ( 'NONE',  ( 10.01549611932653860, 210.2015048109876716, 85.85113791807857808 ) ) ;
#1758=CARTESIAN_POINT ( 'NONE',  ( -6.500168698208244500, 211.6636982574061676, 86.79886208192142760 ) ) ;
#1761=CARTESIAN_POINT ( 'NONE',  ( -9.736236675708031640, 214.0148392665760753, 83.79886208192144181 ) ) ;
#1763=CARTESIAN_POINT ( 'NONE',  ( -6.220909254589537696, 198.5229672870051445, 18.05113791807856671 ) ) ;
#1768=CARTESIAN_POINT ( 'NONE',  ( 7.456977232089302632, 217.1783343296989131, 82.55113791807858092 ) ) ;
#1769=CARTESIAN_POINT ( 'NONE',  ( -9.996365641501871124, 207.8097375604742467, 102.5363179372327096 ) ) ;
#1771=CARTESIAN_POINT ( 'NONE',  ( 0.05014649552828288198, 194.3824533091408000, 67.74886208192143044 ) ) ;
#1772=CARTESIAN_POINT ( 'NONE',  ( -10.00000000000000711, 206.9523078486584495, 80.49886208192143044 ) ) ;
#1773=CARTESIAN_POINT ( 'NONE',  ( -7.456977232089471386, 217.1783343296987709, 14.94886208192143506 ) ) ;
#1775=CARTESIAN_POINT ( 'NONE',  ( 10.00000000000000711, 206.9523078486586201, 29.00113791807856956 ) ) ;
#1777=CARTESIAN_POINT ( 'NONE',  ( 10.00000000000000711, 207.0476921513415220, 93.99886208192144466 ) ) ;
#1782=CARTESIAN_POINT ( 'NONE',  ( 7.984503880673422316, 209.6470497212048372, 81.84886208192142476 ) ) ;
#1783=ORIENTED_EDGE ( 'NONE', *, *, #27467, .F. ) ;
#1791=CARTESIAN_POINT ( 'NONE',  ( 2.517493886308900919, 214.5937144450984420, 76.40113791807856103 ) ) ;
#1796=CARTESIAN_POINT ( 'NONE',  ( -0.05014649552828365914, 215.4116977939061144, 57.24886208192145887 ) ) ;
#1805=CARTESIAN_POINT ( 'NONE',  ( 7.375838497908181246, 196.7627149292499666, 53.45113791807857240 ) ) ;
#1807=CARTESIAN_POINT ( 'NONE',  ( -11.98450388067348804, 210.9467285061362247, 0.6511379180785656917 ) ) ;
#1809=CARTESIAN_POINT ( 'NONE',  ( 3.135527875058820690, 216.4958274776887492, 82.40113791807857524 ) ) ;
#1810=CARTESIAN_POINT ( 'NONE',  ( -12.01549611932659722, 210.8513442034533227, 41.64886208192143613 ) ) ;
#1811=CARTESIAN_POINT ( 'NONE',  ( 10.01549611932659367, 203.7984951890124421, 43.14886208192142902 ) ) ;
#1814=CARTESIAN_POINT ( 'NONE',  ( 9.736236675707914401, 214.0148392665762458, 82.70113791807858661 ) ) ;
#1816=CARTESIAN_POINT ( 'NONE',  ( -8.062137200540920645, 212.9164362838581894, 6.801137918078565825 ) ) ;
#1819=CARTESIAN_POINT ( 'NONE',  ( -3.044812012439970683, 197.4746971517856196, 64.89886208192145034 ) ) ;
#1822=CARTESIAN_POINT ( 'NONE',  ( -7.456977232089471386, 217.1783343296987709, 74.94886208192143329 ) ) ;
#1825=CARTESIAN_POINT ( 'NONE',  ( -6.500168698208244500, 211.6636982574061676, 44.79886208192144181 ) ) ;
#1836=CARTESIAN_POINT ( 'NONE',  ( 3.135527875058981895, 197.5041725223112792, 40.59886208192143187 ) ) ;
#1842=CARTESIAN_POINT ( 'NONE',  ( -2.426778023690076225, 199.3768101843759553, 22.89886208192143613 ) ) ;
#1844=CARTESIAN_POINT ( 'NONE',  ( 3.044812012440130555, 197.4746971517856764, 59.60113791807857808 ) ) ;
#1845=CARTESIAN_POINT ( 'NONE',  ( -8.118202686958039038, 201.1607312380087080, 48.20113791807857950 ) ) ;
#1846=CARTESIAN_POINT ( 'NONE',  ( 10.01549611932653860, 210.2015048109876716, 13.85113791807856742 ) ) ;
#1847=CARTESIAN_POINT ( 'NONE',  ( -8.015496119326531499, 204.4483345814780364, 3.351137918078566535 ) ) ;
#1851=CARTESIAN_POINT ( 'NONE',  ( 0.05014649552807549926, 219.6175466908591716, 28.25113791807856245 ) ) ;
#1854=CARTESIAN_POINT ( 'NONE',  ( 3.044812012440130555, 197.4746971517856764, 74.60113791807856387 ) ) ;
#1855=CARTESIAN_POINT ( 'NONE',  ( 6.139770520408367460, 198.4640165459539389, 50.45113791807857240 ) ) ;
#1859=CARTESIAN_POINT ( 'NONE',  ( 11.98450388067341876, 210.9467285061363953, 9.848862081921433642 ) ) ;
#1860=CARTESIAN_POINT ( 'NONE',  ( -6.220909254589682469, 215.4770327129947134, 14.94886208192143329 ) ) ;
#1863=CARTESIAN_POINT ( 'NONE',  ( -3.753561863808691168, 195.6020594897209435, 62.90113791807858945 ) ) ;
#1864=CARTESIAN_POINT ( 'NONE',  ( -6.500168698208129925, 202.3363017425936050, 78.20113791807857240 ) ) ;
#1866=CARTESIAN_POINT ( 'NONE',  ( -6.220909254589682469, 215.4770327129946850, 38.94886208192144039 ) ) ;
#1867=CARTESIAN_POINT ( 'NONE',  ( -9.521242624480144912, 207.9188892840786878, 102.6634595774070533 ) ) ;
#1877=CARTESIAN_POINT ( 'NONE',  ( 2.426778023690261410, 199.3768101843759837, 32.60113791807857098 ) ) ;
#1880=CARTESIAN_POINT ( 'NONE',  ( -3.135527875058982783, 216.4958274776886924, 12.09886208192143542 ) ) ;
#1883=CARTESIAN_POINT ( 'NONE',  ( -2.517493886308901807, 199.4062855549015012, 47.90113791807857524 ) ) ;
#1887=CARTESIAN_POINT ( 'NONE',  ( -3.135527875058982783, 216.4958274776886924, 102.0988620819214390 ) ) ;
#1889=CARTESIAN_POINT ( 'NONE',  ( -6.139770520408369237, 215.5359834540460042, 27.95113791807856174 ) ) ;
#1891=CARTESIAN_POINT ( 'NONE',  ( 6.139770520408368348, 198.4640165459539674, 17.45113791807855819 ) ) ;
#1896=CARTESIAN_POINT ( 'NONE',  ( 3.662846001190051659, 195.5725841191953691, -0.3988620819214345747 ) ) ;
#1900=CARTESIAN_POINT ( 'NONE',  ( -6.220909254589537696, 198.5229672870051161, 51.05113791807856671 ) ) ;
#1907=CARTESIAN_POINT ( 'NONE',  ( -9.680171189290831535, 214.0920067884431148, 24.80113791807857027 ) ) ;
#1910=CARTESIAN_POINT ( 'NONE',  ( -11.00000000000000355, 206.9999999999998863, 103.5000000000000142 ) ) ;
#1911=CARTESIAN_POINT ( 'NONE',  ( 10.01549611932659545, 203.7984951890123853, 7.148862081921433465 ) ) ;
#1915=CARTESIAN_POINT ( 'NONE',  ( -3.135527875058821579, 197.5041725223112223, 62.90113791807858235 ) ) ;
#1917=CARTESIAN_POINT ( 'NONE',  ( 2.426778023690075337, 214.6231898156240447, 21.39886208192143613 ) ) ;
#1920=CARTESIAN_POINT ( 'NONE',  ( 8.000000000000008882, 206.9523078486586485, 2.001137918078566003 ) ) ;
#1922=CARTESIAN_POINT ( 'NONE',  ( 3.753561863808876797, 195.6020594897209719, 91.59886208192145318 ) ) ;
#1927=CARTESIAN_POINT ( 'NONE',  ( 0.05014649552810505201, 217.5146222423826714, 1.251137918078566003 ) ) ;
#1928=CARTESIAN_POINT ( 'NONE',  ( 8.118202686958138514, 201.1607312380088501, 73.29886208192142760 ) ) ;
#1931=CARTESIAN_POINT ( 'NONE',  ( 0.05014649552810505201, 217.5146222423826714, 4.251137918078566003 ) ) ;
#1934=CARTESIAN_POINT ( 'NONE',  ( 10.00000000000000711, 206.9523078486586201, 86.00113791807858377 ) ) ;
#1936=CARTESIAN_POINT ( 'NONE',  ( 6.139770520408368348, 198.4640165459539674, 71.45113791807857240 ) ) ;
#1939=CARTESIAN_POINT ( 'NONE',  ( 11.98450388067341876, 210.9467285061363953, 87.84886208192142476 ) ) ;
#1941=CARTESIAN_POINT ( 'NONE',  ( -8.062137200540920645, 212.9164362838581894, 21.80113791807856671 ) ) ;
#1946=CARTESIAN_POINT ( 'NONE',  ( 3.753561863808689836, 218.3979405102790565, 88.40113791807857524 ) ) ;
#1950=CARTESIAN_POINT ( 'NONE',  ( 3.753561863808876797, 195.6020594897209719, 73.59886208192142476 ) ) ;
#1951=CARTESIAN_POINT ( 'NONE',  ( 10.00000000000000711, 207.0476921513415220, 78.99886208192144466 ) ) ;
#1952=CARTESIAN_POINT ( 'NONE',  ( -7.375838497908014268, 196.7627149292498530, 14.04886208192143471 ) ) ;
#1954=CARTESIAN_POINT ( 'NONE',  ( -8.118202686958039038, 201.1607312380087080, 30.20113791807856884 ) ) ;
#1956=CARTESIAN_POINT ( 'NONE',  ( -6.139770520408224463, 198.4640165459539389, 95.04886208192144181 ) ) ;
#1960=CARTESIAN_POINT ( 'NONE',  ( -6.500168698208244500, 211.6636982574061676, 77.79886208192142760 ) ) ;
#1963=ORIENTED_EDGE ( 'NONE', *, *, #19778, .T. ) ;
#1967=CARTESIAN_POINT ( 'NONE',  ( -0.3755270751584372513, 206.7692714347155629, 108.3323677711371573 ) ) ;
#1968=CARTESIAN_POINT ( 'NONE',  ( 8.015496119326531499, 209.5516654185219636, 82.85113791807857808 ) ) ;
#1972=CARTESIAN_POINT ( 'NONE',  ( -8.015496119326597224, 209.5516654185217362, 56.64886208192143613 ) ) ;
#1979=CARTESIAN_POINT ( 'NONE',  ( -0.05014649552807705357, 194.3824533091408000, 59.75113791807856245 ) ) ;
#1982=CARTESIAN_POINT ( 'NONE',  ( 3.662846001190051659, 195.5725841191953691, 2.601137918078566091 ) ) ;
#1983=CARTESIAN_POINT ( 'NONE',  ( 3.135527875058820690, 216.4958274776887492, 73.40113791807857524 ) ) ;
#1985=CARTESIAN_POINT ( 'NONE',  ( 12.00000000000000711, 207.0476921513415220, 42.99886208192143044 ) ) ;
#1986=CARTESIAN_POINT ( 'NONE',  ( 8.118202686958138514, 201.1607312380088501, 43.29886208192143471 ) ) ;
#1988=CARTESIAN_POINT ( 'NONE',  ( 9.736236675707914401, 214.0148392665762458, 85.70113791807858661 ) ) ;
#1990=CARTESIAN_POINT ( 'NONE',  ( 3.135527875058820690, 216.4958274776887492, 4.401137918078565470 ) ) ;
#1991=CARTESIAN_POINT ( 'NONE',  ( -0.05014649552828403384, 217.5146222423826714, 72.24886208192140202 ) ) ;
#1995=CARTESIAN_POINT ( 'NONE',  ( -9.736236675708031640, 214.0148392665760753, 71.79886208192142760 ) ) ;
#1998=CARTESIAN_POINT ( 'NONE',  ( -8.015496119326597224, 209.5516654185217362, 56.64886208192143613 ) ) ;
#2008=CARTESIAN_POINT ( 'NONE',  ( 9.984503880673420539, 210.2968891136705167, 39.84886208192141765 ) ) ;
#2014=CARTESIAN_POINT ( 'NONE',  ( -7.984503880673422316, 204.3529502787951628, 29.34886208192143897 ) ) ;
#2015=CARTESIAN_POINT ( 'NONE',  ( -9.984503880673473830, 210.2968891136704315, 69.65113791807854682 ) ) ;
#2017=CARTESIAN_POINT ( 'NONE',  ( 3.135527875058820690, 216.4958274776887492, 49.40113791807857524 ) ) ;
#2020=CARTESIAN_POINT ( 'NONE',  ( -8.062137200540920645, 212.9164362838581894, 21.80113791807856671 ) ) ;
#2021=CARTESIAN_POINT ( 'NONE',  ( 8.000000000000008882, 206.9523078486586485, 8.001137918078566003 ) ) ;
#2024=CARTESIAN_POINT ( 'NONE',  ( 12.00000000000000711, 206.9523078486586485, 29.00113791807856956 ) ) ;
#2028=CARTESIAN_POINT ( 'NONE',  ( 10.00000000000000711, 206.9523078486586201, 74.00113791807858377 ) ) ;
#2029=CARTESIAN_POINT ( 'NONE',  ( -9.984503880673475606, 210.2968891136704315, 45.65113791807856813 ) ) ;
#2033=CARTESIAN_POINT ( 'NONE',  ( 11.98450388067341876, 210.9467285061363953, 15.84886208192143719 ) ) ;
#2034=CARTESIAN_POINT ( 'NONE',  ( -3.044812012439970683, 197.4746971517856196, 22.89886208192143613 ) ) ;
#2037=CARTESIAN_POINT ( 'NONE',  ( -11.98450388067348804, 210.9467285061362247, 57.65113791807858945 ) ) ;
#2038=CARTESIAN_POINT ( 'NONE',  ( 6.500168698208129925, 211.6636982574063381, 76.70113791807857240 ) ) ;
#2039=CARTESIAN_POINT ( 'NONE',  ( -3.044812012439970683, 197.4746971517856196, 37.89886208192143613 ) ) ;
#2050=CARTESIAN_POINT ( 'NONE',  ( 7.984503880673485376, 204.3529502787953902, 29.15113791807857169 ) ) ;
#2052=CARTESIAN_POINT ( 'NONE',  ( 10.00000000000000711, 207.0476921513415220, 9.998862081921435774 ) ) ;
#2055=CARTESIAN_POINT ( 'NONE',  ( -2.426778023690262742, 214.6231898156240163, 61.10113791807857808 ) ) ;
#2059=CARTESIAN_POINT ( 'NONE',  ( 3.135527875058981895, 197.5041725223112792, 100.5988620819214390 ) ) ;
#2061=CARTESIAN_POINT ( 'NONE',  ( -10.00000000000000711, 207.0476921513413515, 39.50113791807856956 ) ) ;
#2062=DIRECTION ( 'NONE',  ( -0.08583835255247916629, -0.09953364313786493278, -0.9913247858874408847 ) ) ;
#2064=CARTESIAN_POINT ( 'NONE',  ( 6.220909254589536808, 215.4770327129947702, 16.55113791807857027 ) ) ;
#2068=CARTESIAN_POINT ( 'NONE',  ( -9.949154985843399857, 217.7087784572769067, 102.9933096652613074 ) ) ;
#2072=CARTESIAN_POINT ( 'NONE',  ( -8.062137200540920645, 212.9164362838581894, 45.80113791807856671 ) ) ;
#2078=CARTESIAN_POINT ( 'NONE',  ( -12.00000000000000711, 207.0476921513413515, 33.50113791807857666 ) ) ;
#2079=AXIS2_PLACEMENT_3D ( 'NONE', #27844, #33644, #25468 ) ;
#2082=CARTESIAN_POINT ( 'NONE',  ( 8.118202686958138514, 201.1607312380088501, 13.29886208192143648 ) ) ;
#2086=CARTESIAN_POINT ( 'NONE',  ( 10.01549611932653860, 210.2015048109876716, 7.851137918078566535 ) ) ;
#2087=CARTESIAN_POINT ( 'NONE',  ( 6.139770520408368348, 198.4640165459539674, 59.45113791807855819 ) ) ;
#2089=CARTESIAN_POINT ( 'NONE',  ( 8.000000000000008882, 207.0476921513415220, 21.99886208192143400 ) ) ;
#2093=CARTESIAN_POINT ( 'NONE',  ( 8.000000000000008882, 206.9523078486586485, 5.001137918078565114 ) ) ;
#2097=CARTESIAN_POINT ( 'NONE',  ( -9.736236675708031640, 214.0148392665760753, 92.79886208192142760 ) ) ;
#2104=CARTESIAN_POINT ( 'NONE',  ( 8.118202686958138514, 201.1607312380088501, 67.29886208192144181 ) ) ;
#2107=CARTESIAN_POINT ( 'NONE',  ( 10.00000000000000711, 206.9523078486586201, -0.9988620819214343305 ) ) ;
#2108=CARTESIAN_POINT ( 'NONE',  ( 8.551039143100586770, 208.8253170565643302, -0.4549153643320096307 ) ) ;
#2112=CARTESIAN_POINT ( 'NONE',  ( 8.118202686958039038, 212.8392687619912635, 91.70113791807857240 ) ) ;
#2114=CARTESIAN_POINT ( 'NONE',  ( 8.118202686958039038, 212.8392687619912635, 73.70113791807857240 ) ) ;
#2118=CARTESIAN_POINT ( 'NONE',  ( 3.662846001189864698, 218.4274158808046593, 84.39886208192143613 ) ) ;
#2121=CARTESIAN_POINT ( 'NONE',  ( 3.135527875058820690, 216.4958274776887492, 34.40113791807856813 ) ) ;
#2125=CARTESIAN_POINT ( 'NONE',  ( 3.753561863808689836, 218.3979405102790565, 97.40113791807858945 ) ) ;
#2128=CARTESIAN_POINT ( 'NONE',  ( 3.044812012439969795, 216.5253028482143520, 90.39886208192143613 ) ) ;
#2129=CARTESIAN_POINT ( 'NONE',  ( 9.680171189290716072, 214.0920067884432854, 27.69886208192143684 ) ) ;
#2132=CARTESIAN_POINT ( 'NONE',  ( 3.135527875058820690, 216.4958274776887492, 37.40113791807857524 ) ) ;
#2134=CARTESIAN_POINT ( 'NONE',  ( 10.01549611932659545, 203.7984951890123853, 94.14886208192143613 ) ) ;
#2138=CARTESIAN_POINT ( 'NONE',  ( -2.426778023690076225, 199.3768101843759553, 79.89886208192143613 ) ) ;
#2146=CARTESIAN_POINT ( 'NONE',  ( -7.984503880673488041, 209.6470497212046098, 78.65113791807858945 ) ) ;
#2150=CARTESIAN_POINT ( 'NONE',  ( -6.444103211790928043, 202.2591342207265939, 53.19886208192144039 ) ) ;
#2151=AXIS2_PLACEMENT_3D ( 'NONE', #32067, #18460, #11129 ) ;
#2157=CARTESIAN_POINT ( 'NONE',  ( 0.05014649552807549926, 219.6175466908591716, 64.25113791807856956 ) ) ;
#2159=CARTESIAN_POINT ( 'NONE',  ( 3.753561863808689836, 218.3979405102790565, 7.401137918078566358 ) ) ;
#2160=CARTESIAN_POINT ( 'NONE',  ( 9.984503880673473830, 203.7031108863295401, 77.15113791807857524 ) ) ;
#2161=CARTESIAN_POINT ( 'NONE',  ( -3.753561863808878130, 218.3979405102790281, 39.09886208192143187 ) ) ;
#2162=CARTESIAN_POINT ( 'NONE',  ( 8.062137200540822946, 212.9164362838583315, 60.69886208192143329 ) ) ;
#2164=CARTESIAN_POINT ( 'NONE',  ( -0.05014649552807705357, 194.3824533091408000, 83.75113791807856956 ) ) ;
#2166=CARTESIAN_POINT ( 'NONE',  ( 3.044812012440130555, 197.4746971517856764, 8.601137918078565647 ) ) ;
#2167=CARTESIAN_POINT ( 'NONE',  ( 3.044812012439969795, 216.5253028482143520, 66.39886208192143613 ) ) ;
#2170=CARTESIAN_POINT ( 'NONE',  ( -11.98450388067341876, 203.0532714938636047, 71.34886208192142476 ) ) ;
#2173=CARTESIAN_POINT ( 'NONE',  ( -6.444103211790928043, 202.2591342207265939, 50.19886208192144750 ) ) ;
#2181=CARTESIAN_POINT ( 'NONE',  ( 8.118202686958138514, 201.1607312380088501, 46.29886208192143471 ) ) ;
#2187=CARTESIAN_POINT ( 'NONE',  ( -0.05014649552828365914, 215.4116977939061144, 27.24886208192143755 ) ) ;
#2188=CARTESIAN_POINT ( 'NONE',  ( 3.044812012440130555, 197.4746971517856764, 68.60113791807857808 ) ) ;
#2191=CARTESIAN_POINT ( 'NONE',  ( -9.984503880673473830, 210.2968891136704315, 54.65113791807858235 ) ) ;
#2193=CARTESIAN_POINT ( 'NONE',  ( 8.118202686958039038, 212.8392687619912635, 19.70113791807856884 ) ) ;
#2194=CARTESIAN_POINT ( 'NONE',  ( 0.05014649552807626948, 215.4116977939061144, 7.251137918078565114 ) ) ;
#2197=CARTESIAN_POINT ( 'NONE',  ( 3.662846001190051659, 195.5725841191953691, 32.60113791807857098 ) ) ;
#2199=CARTESIAN_POINT ( 'NONE',  ( -6.139770520408369237, 215.5359834540460042, 75.95113791807857240 ) ) ;
#2200=CARTESIAN_POINT ( 'NONE',  ( 9.984503880673473830, 203.7031108863295401, 47.15113791807857524 ) ) ;
#2202=CARTESIAN_POINT ( 'NONE',  ( 7.456977232089471386, 196.8216656703012006, 10.44886208192143506 ) ) ;
#2203=CARTESIAN_POINT ( 'NONE',  ( 8.062137200540822946, 212.9164362838583315, 24.69886208192143684 ) ) ;
#2206=CARTESIAN_POINT ( 'NONE',  ( 3.662846001190051659, 195.5725841191953691, 53.60113791807856387 ) ) ;
#2207=CARTESIAN_POINT ( 'NONE',  ( 7.984503880673485376, 204.3529502787953902, 80.15113791807857524 ) ) ;
#2208=CARTESIAN_POINT ( 'NONE',  ( 8.118202686958138514, 201.1607312380088501, 40.29886208192143471 ) ) ;
#2211=CARTESIAN_POINT ( 'NONE',  ( -3.662846001189865142, 195.5725841191952838, 43.89886208192143613 ) ) ;
#2217=CARTESIAN_POINT ( 'NONE',  ( -6.500168698208129925, 202.3363017425936050, 36.20113791807857240 ) ) ;
#2219=CARTESIAN_POINT ( 'NONE',  ( 10.01549611932659545, 203.7984951890123853, 13.14886208192143258 ) ) ;
#2222=CARTESIAN_POINT ( 'NONE',  ( 2.517493886308900919, 214.5937144450984420, 55.40113791807858235 ) ) ;
#2226=CARTESIAN_POINT ( 'NONE',  ( 10.00000000000000711, 207.0476921513415220, 96.99886208192143044 ) ) ;
#2228=CARTESIAN_POINT ( 'NONE',  ( 8.062137200540920645, 201.0835637161417822, 38.30113791807857382 ) ) ;
#2229=DIRECTION ( 'NONE',  ( 0.000000000000000000, 0.9949972439410067482, -0.09990237509589337817 ) ) ;
#2231=CARTESIAN_POINT ( 'NONE',  ( -10.00000000000000711, 207.0476921513413515, 21.50113791807856956 ) ) ;
#2232=CARTESIAN_POINT ( 'NONE',  ( -10.00000000000000711, 206.9523078486584495, 101.4988620819214304 ) ) ;
#2236=CARTESIAN_POINT ( 'NONE',  ( 8.118202686958039038, 212.8392687619912635, 100.7011379180785866 ) ) ;
#2240=CARTESIAN_POINT ( 'NONE',  ( 0.05014649552810505201, 217.5146222423826714, 49.25113791807857666 ) ) ;
#2247=CARTESIAN_POINT ( 'NONE',  ( 7.456977232089302632, 217.1783343296989131, 25.55113791807857027 ) ) ;
#2249=CARTESIAN_POINT ( 'NONE',  ( -10.01549611932659722, 210.2015048109875011, 8.648862081921436129 ) ) ;
#2252=CARTESIAN_POINT ( 'NONE',  ( 0.05014649552810505201, 217.5146222423826714, 10.25113791807856778 ) ) ;
#2253=CARTESIAN_POINT ( 'NONE',  ( -10.00000000000000711, 207.0476921513413515, 75.50113791807858377 ) ) ;
#2256=CARTESIAN_POINT ( 'NONE',  ( 8.000000000000008882, 207.0476921513415220, 24.99886208192143400 ) ) ;
#2260=CARTESIAN_POINT ( 'NONE',  ( -4.984841277089726574, 200.2242689037092305, 3.051137918078566269 ) ) ;
#2262=CARTESIAN_POINT ( 'NONE',  ( -12.00000000000000711, 206.9523078486584780, 86.49886208192144466 ) ) ;
#2267=CARTESIAN_POINT ( 'NONE',  ( 10.00000000000000711, 206.9523078486586201, 8.001137918078566003 ) ) ;
#2268=CARTESIAN_POINT ( 'NONE',  ( 9.984503880673420539, 210.2968891136705167, 69.84886208192143897 ) ) ;
#2271=CARTESIAN_POINT ( 'NONE',  ( 3.044812012440130555, 197.4746971517856764, 17.60113791807856742 ) ) ;
#2274=CARTESIAN_POINT ( 'NONE',  ( 8.118202686958039038, 212.8392687619912635, 94.70113791807857240 ) ) ;
#2276=CARTESIAN_POINT ( 'NONE',  ( 0.05014649552810505201, 217.5146222423826714, 76.25113791807855534 ) ) ;
#2279=CARTESIAN_POINT ( 'NONE',  ( -11.98450388067341876, 203.0532714938636047, 83.34886208192143897 ) ) ;
#2281=CARTESIAN_POINT ( 'NONE',  ( 10.01549611932653860, 210.2015048109876716, 28.85113791807856387 ) ) ;
#2286=CARTESIAN_POINT ( 'NONE',  ( -3.753561863808691168, 195.6020594897209435, 98.90113791807858945 ) ) ;
#2289=ORIENTED_EDGE ( 'NONE', *, *, #7532, .F. ) ;
#2290=CARTESIAN_POINT ( 'NONE',  ( 3.135527875058981895, 197.5041725223112792, 85.59886208192143897 ) ) ;
#2292=CARTESIAN_POINT ( 'NONE',  ( 11.98450388067341876, 210.9467285061363953, 21.84886208192143542 ) ) ;
#2294=CARTESIAN_POINT ( 'NONE',  ( -10.00000000000000711, 207.0476921513413515, 30.50113791807856600 ) ) ;
#2297=CARTESIAN_POINT ( 'NONE',  ( -10.00000000000000711, 206.9523078486584495, 95.49886208192144466 ) ) ;
#2301=CARTESIAN_POINT ( 'NONE',  ( -2.426778023690076225, 199.3768101843759553, 82.89886208192143613 ) ) ;
#2307=CARTESIAN_POINT ( 'NONE',  ( -6.444103211791042618, 211.7408657792732356, 60.80113791807858092 ) ) ;
#2310=CARTESIAN_POINT ( 'NONE',  ( 0.05014649552807626948, 215.4116977939061144, 88.25113791807856956 ) ) ;
#2315=CARTESIAN_POINT ( 'NONE',  ( 7.984503880673422316, 209.6470497212048372, 63.84886208192143187 ) ) ;
#2317=CARTESIAN_POINT ( 'NONE',  ( 9.984503880673473830, 203.7031108863295401, 2.151137918078566358 ) ) ;
#2322=CARTESIAN_POINT ( 'NONE',  ( -7.456977232089304408, 196.8216656703010301, 63.05113791807858092 ) ) ;
#2324=CARTESIAN_POINT ( 'NONE',  ( 12.01549611932652972, 210.8513442034534933, 10.85113791807856565 ) ) ;
#2326=CARTESIAN_POINT ( 'NONE',  ( 6.139770520408367460, 198.4640165459539389, 92.45113791807857240 ) ) ;
#2327=CARTESIAN_POINT ( 'NONE',  ( 3.662846001189864698, 218.4274158808046593, 48.39886208192143613 ) ) ;
#2328=PRODUCT_DEFINITION_FORMATION_WITH_SPECIFIED_SOURCE ( 'ANY', '', #23052, .NOT_KNOWN. ) ;
#2329=CARTESIAN_POINT ( 'NONE',  ( -6.220909254589682469, 215.4770327129947134, 56.94886208192143329 ) ) ;
#2331=CARTESIAN_POINT ( 'NONE',  ( -3.753561863808691168, 195.6020594897209435, 98.90113791807858945 ) ) ;
#2333=CARTESIAN_POINT ( 'NONE',  ( -3.044812012440131443, 216.5253028482142952, 4.101137918078565647 ) ) ;
#2335=CARTESIAN_POINT ( 'NONE',  ( 0.05014649552828275708, 196.4853777576173002, 70.74886208192143044 ) ) ;
#2338=CARTESIAN_POINT ( 'NONE',  ( 9.680171189290716072, 214.0920067884432854, 81.69886208192144750 ) ) ;
#2339=CARTESIAN_POINT ( 'NONE',  ( 3.044812012440130555, 197.4746971517856764, 92.60113791807857808 ) ) ;
#2343=CARTESIAN_POINT ( 'NONE',  ( 4.903702542908435547, 213.8346818373419751, 54.54886208192144181 ) ) ;
#2350=CARTESIAN_POINT ( 'NONE',  ( -0.05014649552828403384, 217.5146222423826714, 48.24886208192142334 ) ) ;
#2355=CARTESIAN_POINT ( 'NONE',  ( -6.500168698208244500, 211.6636982574061676, 38.79886208192143471 ) ) ;
#2356=CARTESIAN_POINT ( 'NONE',  ( -8.062137200540920645, 212.9164362838581894, 69.80113791807856671 ) ) ;
#2358=CARTESIAN_POINT ( 'NONE',  ( 6.139770520408368348, 198.4640165459539674, 53.45113791807855108 ) ) ;
#2360=CARTESIAN_POINT ( 'NONE',  ( 3.135527875058820690, 216.4958274776887492, 31.40113791807857524 ) ) ;
#2361=CARTESIAN_POINT ( 'NONE',  ( -2.426778023690262742, 214.6231898156240163, 1.101137918078566091 ) ) ;
#2366=CARTESIAN_POINT ( 'NONE',  ( -7.375838497908182134, 217.2372850707499765, 36.95113791807856529 ) ) ;
#2369=CARTESIAN_POINT ( 'NONE',  ( 3.044812012440130555, 197.4746971517856764, 86.60113791807857808 ) ) ;
#2370=CARTESIAN_POINT ( 'NONE',  ( -3.044812012440131443, 216.5253028482142952, 61.10113791807857098 ) ) ;
#2373=CARTESIAN_POINT ( 'NONE',  ( -9.680171189290716072, 199.9079932115567146, 17.19886208192143684 ) ) ;
#2374=CARTESIAN_POINT ( 'NONE',  ( 6.220909254589680693, 198.5229672870052582, 25.44886208192143684 ) ) ;
#2377=CARTESIAN_POINT ( 'NONE',  ( -0.05014649552807705357, 194.3824533091408000, 71.75113791807856956 ) ) ;
#2378=CARTESIAN_POINT ( 'NONE',  ( 0.05014649552807626948, 215.4116977939061144, 76.25113791807856956 ) ) ;
#2379=CARTESIAN_POINT ( 'NONE',  ( -9.984503880673420539, 203.7031108863293980, 38.34886208192143897 ) ) ;
#2382=CARTESIAN_POINT ( 'NONE',  ( -7.456977232089471386, 217.1783343296987709, 38.94886208192143329 ) ) ;
#2390=CARTESIAN_POINT ( 'NONE',  ( 4.984841277089725686, 213.7757310962907411, 37.55113791807855961 ) ) ;
#2393=CARTESIAN_POINT ( 'NONE',  ( 8.062137200540822946, 212.9164362838583315, 27.69886208192143684 ) ) ;
#2400=CARTESIAN_POINT ( 'NONE',  ( -3.135527875058982783, 216.4958274776886924, 99.09886208192143897 ) ) ;
#2401=CARTESIAN_POINT ( 'NONE',  ( -3.044812012440131443, 216.5253028482142952, 46.10113791807857098 ) ) ;
#2402=CARTESIAN_POINT ( 'NONE',  ( 10.01549611932653860, 210.2015048109876716, 22.85113791807856742 ) ) ;
#2404=AXIS2_PLACEMENT_3D ( 'NONE', #8872, #11941, #4266 ) ;
#2405=CARTESIAN_POINT ( 'NONE',  ( 8.000000000000008882, 207.0476921513415220, 84.99886208192144466 ) ) ;
#2409=CARTESIAN_POINT ( 'NONE',  ( 9.736236675707914401, 214.0148392665762458, 13.70113791807856707 ) ) ;
#2412=CARTESIAN_POINT ( 'NONE',  ( -9.984503880673473830, 210.2968891136704315, 60.65113791807856103 ) ) ;
#2419=CARTESIAN_POINT ( 'NONE',  ( 0.05014649552807549926, 219.6175466908591716, 25.25113791807856956 ) ) ;
#2423=CARTESIAN_POINT ( 'NONE',  ( -6.139770520408224463, 198.4640165459539389, 8.048862081921434708 ) ) ;
#2426=CARTESIAN_POINT ( 'NONE',  ( -8.062137200540920645, 212.9164362838581894, 12.80113791807856671 ) ) ;
#2427=CARTESIAN_POINT ( 'NONE',  ( 10.00000000000000711, 206.9523078486586201, 74.00113791807858377 ) ) ;
#2429=CARTESIAN_POINT ( 'NONE',  ( -7.984503880673422316, 204.3529502787951628, 35.34886208192144608 ) ) ;
#2435=CARTESIAN_POINT ( 'NONE',  ( 2.517493886308900919, 214.5937144450984420, 7.401137918078566358 ) ) ;
#2436=CARTESIAN_POINT ( 'NONE',  ( 12.01549611932659367, 203.1486557965466773, 97.14886208192146455 ) ) ;
#2442=CARTESIAN_POINT ( 'NONE',  ( 3.135527875058820690, 216.4958274776887492, 10.40113791807856636 ) ) ;
#2443=AXIS2_PLACEMENT_3D ( 'NONE', #24136, #3023, #21414 ) ;
#2444=CARTESIAN_POINT ( 'NONE',  ( 6.139770520408223575, 215.5359834540460611, 75.54886208192139918 ) ) ;
#2447=CARTESIAN_POINT ( 'NONE',  ( -0.05014649552810635652, 196.4853777576173002, 8.751137918078562450 ) ) ;
#2450=CARTESIAN_POINT ( 'NONE',  ( 6.220909254589536808, 215.4770327129947702, 100.5511379180785809 ) ) ;
#2452=CARTESIAN_POINT ( 'NONE',  ( 10.00000000000000711, 206.9523078486586201, 80.00113791807856956 ) ) ;
#2455=CARTESIAN_POINT ( 'NONE',  ( -0.05014649552828442242, 219.6175466908591716, 93.24886208192143044 ) ) ;
#2460=CARTESIAN_POINT ( 'NONE',  ( 9.736236675707914401, 214.0148392665762458, 91.70113791807857240 ) ) ;
#2464=CARTESIAN_POINT ( 'NONE',  ( 3.135527875058981895, 197.5041725223112792, 82.59886208192143897 ) ) ;
#2465=CARTESIAN_POINT ( 'NONE',  ( 7.375838497908012492, 217.2372850707501186, 21.54886208192143471 ) ) ;
#2467=CARTESIAN_POINT ( 'NONE',  ( -3.135527875058821579, 197.5041725223112223, 44.90113791807857524 ) ) ;
#2469=CARTESIAN_POINT ( 'NONE',  ( 6.500168698208244500, 202.3363017425938324, 1.298862081921434930 ) ) ;
#2473=CARTESIAN_POINT ( 'NONE',  ( -8.015496119326597224, 209.5516654185217362, 83.64886208192143613 ) ) ;
#2479=CARTESIAN_POINT ( 'NONE',  ( -8.000000000000008882, 207.0476921513413515, 57.50113791807857666 ) ) ;
#2482=CARTESIAN_POINT ( 'NONE',  ( 2.426778023690261410, 199.3768101843759837, 89.60113791807857808 ) ) ;
#2486=CARTESIAN_POINT ( 'NONE',  ( -7.984503880673422316, 204.3529502787951628, 62.34886208192144608 ) ) ;
#2487=CARTESIAN_POINT ( 'NONE',  ( -1.474514954580286030E-14, 206.9977241638431167, -6.000000000000014211 ) ) ;
#2494=CARTESIAN_POINT ( 'NONE',  ( 12.01549611932652972, 210.8513442034534933, 70.85113791807857808 ) ) ;
#2496=CARTESIAN_POINT ( 'NONE',  ( 12.01549611932652972, 210.8513442034534933, 7.851137918078565647 ) ) ;
#2497=CARTESIAN_POINT ( 'NONE',  ( -8.118202686958039038, 201.1607312380087080, 84.20113791807858661 ) ) ;
#2498=CARTESIAN_POINT ( 'NONE',  ( 9.736236675708031640, 199.9851607334238963, 52.29886208192143471 ) ) ;
#2499=CARTESIAN_POINT ( 'NONE',  ( -0.05014649552828402690, 217.5146222423826714, 57.24886208192143755 ) ) ;
#2501=CARTESIAN_POINT ( 'NONE',  ( 12.00000000000000711, 206.9523078486586485, 95.00113791807856956 ) ) ;
#2503=CARTESIAN_POINT ( 'NONE',  ( -6.220909254589537696, 198.5229672870051161, 18.05113791807856671 ) ) ;
#2504=CARTESIAN_POINT ( 'NONE',  ( -0.05014649552828403384, 217.5146222423826714, 66.24886208192143044 ) ) ;
#2506=CARTESIAN_POINT ( 'NONE',  ( 12.00000000000000711, 207.0476921513415220, 81.99886208192144466 ) ) ;
#2507=CARTESIAN_POINT ( 'NONE',  ( -9.984503880673473830, 210.2968891136704315, 87.65113791807854682 ) ) ;
#2510=CARTESIAN_POINT ( 'NONE',  ( -8.015496119326597224, 209.5516654185217362, 47.64886208192145034 ) ) ;
#2519=CARTESIAN_POINT ( 'NONE',  ( -6.139770520408224463, 198.4640165459539389, 50.04886208192143471 ) ) ;
#2524=CARTESIAN_POINT ( 'NONE',  ( -6.500168698208244500, 211.6636982574061676, 32.79886208192143471 ) ) ;
#2526=CARTESIAN_POINT ( 'NONE',  ( -6.220909254589537696, 198.5229672870051161, 69.05113791807858092 ) ) ;
#2529=CARTESIAN_POINT ( 'NONE',  ( 10.00000000000000711, 206.9523078486586201, 53.00113791807857666 ) ) ;
#2531=CARTESIAN_POINT ( 'NONE',  ( -0.05014649552810635652, 196.4853777576173002, 26.75113791807856956 ) ) ;
#2532=CARTESIAN_POINT ( 'NONE',  ( 7.984503880673485376, 204.3529502787953902, 11.15113791807856636 ) ) ;
#2536=CARTESIAN_POINT ( 'NONE',  ( -11.98450388067348804, 210.9467285061362247, 39.65113791807857524 ) ) ;
#2539=CARTESIAN_POINT ( 'NONE',  ( 10.01549611932653860, 210.2015048109876716, 88.85113791807857808 ) ) ;
#2540=CARTESIAN_POINT ( 'NONE',  ( 6.220909254589536808, 215.4770327129947987, 58.55113791807858092 ) ) ;
#2542=CARTESIAN_POINT ( 'NONE',  ( 7.456977232089471386, 196.8216656703012006, 22.44886208192143329 ) ) ;
#2543=CARTESIAN_POINT ( 'NONE',  ( -9.984503880673420539, 203.7031108863293980, 32.34886208192143187 ) ) ;
#2545=CARTESIAN_POINT ( 'NONE',  ( 11.98450388067348271, 203.0532714938637753, 68.15113791807856103 ) ) ;
#2546=CARTESIAN_POINT ( 'NONE',  ( 4.903702542908601636, 200.1653181626581102, 80.45113791807857240 ) ) ;
#2547=CARTESIAN_POINT ( 'NONE',  ( 3.044812012439969795, 216.5253028482143520, 39.39886208192143613 ) ) ;
#2551=CARTESIAN_POINT ( 'NONE',  ( -7.375838497908014268, 196.7627149292498530, 50.04886208192142760 ) ) ;
#2559=CARTESIAN_POINT ( 'NONE',  ( 4.903702542908601636, 200.1653181626581102, 38.45113791807856529 ) ) ;
#2561=CARTESIAN_POINT ( 'NONE',  ( -8.118202686958138514, 212.8392687619910930, 23.79886208192143471 ) ) ;
#2567=CARTESIAN_POINT ( 'NONE',  ( -2.517493886309087880, 214.5937144450984135, 3.098862081921434974 ) ) ;
#2568=CARTESIAN_POINT ( 'NONE',  ( 10.00000000000000711, 206.9523078486586201, 44.00113791807857666 ) ) ;
#2570=CARTESIAN_POINT ( 'NONE',  ( -0.05014649552810635652, 196.4853777576173002, 29.75113791807856956 ) ) ;
#2575=CARTESIAN_POINT ( 'NONE',  ( -8.000000000000008882, 206.9523078486584780, 92.49886208192144466 ) ) ;
#2579=CARTESIAN_POINT ( 'NONE',  ( 7.456977232089302632, 217.1783343296989131, 7.551137918078564049 ) ) ;
#2582=CARTESIAN_POINT ( 'NONE',  ( -8.062137200540920645, 212.9164362838581894, 57.80113791807857382 ) ) ;
#2589=CARTESIAN_POINT ( 'NONE',  ( 9.736236675707914401, 214.0148392665762458, 37.70113791807857240 ) ) ;
#2591=CARTESIAN_POINT ( 'NONE',  ( -0.05014649552828403384, 217.5146222423826714, 12.24886208192143755 ) ) ;
#2593=EDGE_LOOP ( 'NONE', ( #30834, #2607, #27081, #23781 ) ) ;
#2594=CARTESIAN_POINT ( 'NONE',  ( 0.05014649552810505201, 217.5146222423826714, 13.25113791807856778 ) ) ;
#2595=CARTESIAN_POINT ( 'NONE',  ( -3.135527875058821579, 197.5041725223112223, 74.90113791807857524 ) ) ;
#2598=CARTESIAN_POINT ( 'NONE',  ( 6.500168698208244500, 202.3363017425938324, 34.29886208192144181 ) ) ;
#2603=CARTESIAN_POINT ( 'NONE',  ( -2.517493886308901807, 199.4062855549015012, 14.90113791807856636 ) ) ;
#2604=CARTESIAN_POINT ( 'NONE',  ( -3.662846001189865142, 195.5725841191952838, 97.89886208192146455 ) ) ;
#2606=AXIS2_PLACEMENT_3D ( 'NONE', #2487, #31106, #7768 ) ;
#2607=ORIENTED_EDGE ( 'NONE', *, *, #7532, .T. ) ;
#2610=CARTESIAN_POINT ( 'NONE',  ( -10.01549611932653860, 203.7984951890123284, 9.351137918078569200 ) ) ;
#2611=CARTESIAN_POINT ( 'NONE',  ( 6.139770520408223575, 215.5359834540460611, 84.54886208192141339 ) ) ;
#2614=CARTESIAN_POINT ( 'NONE',  ( -3.044812012440131443, 216.5253028482142952, 13.10113791807856742 ) ) ;
#2617=CARTESIAN_POINT ( 'NONE',  ( -10.00000000000000711, 207.0476921513413515, 96.50113791807856956 ) ) ;
#2619=CARTESIAN_POINT ( 'NONE',  ( 10.00000000000000711, 206.9523078486586201, 83.00113791807856956 ) ) ;
#2623=CARTESIAN_POINT ( 'NONE',  ( -7.375838497908014268, 196.7627149292498530, 92.04886208192142760 ) ) ;
#2631=CARTESIAN_POINT ( 'NONE',  ( 12.00000000000000711, 206.9523078486586485, 98.00113791807856956 ) ) ;
#2635=CARTESIAN_POINT ( 'NONE',  ( 10.00000000000000711, 207.0476921513415220, 90.99886208192144466 ) ) ;
#2636=CARTESIAN_POINT ( 'NONE',  ( -3.662846001189865142, 195.5725841191952838, 19.89886208192143613 ) ) ;
#2638=CARTESIAN_POINT ( 'NONE',  ( 10.01549611932653860, 210.2015048109876716, 40.85113791807857098 ) ) ;
#2640=CARTESIAN_POINT ( 'NONE',  ( 0.05014649552828262524, 198.5883022060938572, 1.748862081921434886 ) ) ;
#2643=CARTESIAN_POINT ( 'NONE',  ( 8.000000000000008882, 207.0476921513415220, 87.99886208192144466 ) ) ;
#2644=CIRCLE ( 'NONE', #443, 0.9999999999999992228 ) ;
#2647=CARTESIAN_POINT ( 'NONE',  ( 8.000000000000008882, 206.9523078486586485, 35.00113791807857666 ) ) ;
#2653=CARTESIAN_POINT ( 'NONE',  ( 4.984841277089725686, 213.7757310962907411, 88.55113791807858092 ) ) ;
#2658=CARTESIAN_POINT ( 'NONE',  ( 8.000000000000008882, 207.0476921513415220, 63.99886208192143044 ) ) ;
#2662=CARTESIAN_POINT ( 'NONE',  ( -8.062137200540920645, 212.9164362838581894, 0.8011379180785658249 ) ) ;
#2666=CARTESIAN_POINT ( 'NONE',  ( 7.375838497908181246, 196.7627149292499666, 71.45113791807854398 ) ) ;
#2668=AXIS2_PLACEMENT_3D ( 'NONE', #29695, #24760, #11645 ) ;
#2669=CARTESIAN_POINT ( 'NONE',  ( -3.753561863808691168, 195.6020594897209435, 11.90113791807856813 ) ) ;
#2670=CARTESIAN_POINT ( 'NONE',  ( 10.00000000000000711, 206.9523078486586201, 83.00113791807856956 ) ) ;
#2674=CARTESIAN_POINT ( 'NONE',  ( 7.456977232089471386, 196.8216656703012006, 49.44886208192144039 ) ) ;
#2675=CARTESIAN_POINT ( 'NONE',  ( 0.05014649552828275014, 196.4853777576173002, 58.74886208192143044 ) ) ;
#2676=CARTESIAN_POINT ( 'NONE',  ( -3.662846001190052991, 218.4274158808045740, 94.10113791807857808 ) ) ;
#2678=CARTESIAN_POINT ( 'NONE',  ( -9.984503880673473830, 210.2968891136704315, 9.651137918078568134 ) ) ;
#2679=CARTESIAN_POINT ( 'NONE',  ( 0.05014649552828275708, 196.4853777576173002, 79.74886208192143044 ) ) ;
#2683=CARTESIAN_POINT ( 'NONE',  ( 0.05014649552828288198, 194.3824533091408000, 79.74886208192143044 ) ) ;
#2687=CARTESIAN_POINT ( 'NONE',  ( 2.517493886309087436, 199.4062855549015865, 58.59886208192145318 ) ) ;
#2697=CARTESIAN_POINT ( 'NONE',  ( -3.044812012439970683, 197.4746971517856196, 49.89886208192143613 ) ) ;
#2702=CARTESIAN_POINT ( 'NONE',  ( 4.984841277089891776, 200.2242689037093726, 37.44886208192144039 ) ) ;
#2703=CARTESIAN_POINT ( 'NONE',  ( -6.220909254589537696, 198.5229672870051161, 75.05113791807858092 ) ) ;
#2705=CARTESIAN_POINT ( 'NONE',  ( 10.00000000000000711, 206.9523078486586201, 56.00113791807856956 ) ) ;
#2706=CARTESIAN_POINT ( 'NONE',  ( -3.044812012440131443, 216.5253028482142952, 28.10113791807857098 ) ) ;
#2707=CARTESIAN_POINT ( 'NONE',  ( 2.517493886308900919, 214.5937144450984420, 16.40113791807856458 ) ) ;
#2712=CARTESIAN_POINT ( 'NONE',  ( -9.736236675707914401, 199.9851607334237542, 39.20113791807857240 ) ) ;
#2714=CARTESIAN_POINT ( 'NONE',  ( 10.00000000000000711, 206.9523078486586201, 86.00113791807858377 ) ) ;
#2715=CARTESIAN_POINT ( 'NONE',  ( 0.05014649552810506589, 217.5146222423826714, 58.25113791807856956 ) ) ;
#2716=CARTESIAN_POINT ( 'NONE',  ( 12.01549611932659367, 203.1486557965466773, 19.14886208192143968 ) ) ;
#2717=CARTESIAN_POINT ( 'NONE',  ( -3.135527875058982783, 216.4958274776886924, 33.09886208192143187 ) ) ;
#2719=CARTESIAN_POINT ( 'NONE',  ( -3.662846001190052991, 218.4274158808045740, 70.10113791807857808 ) ) ;
#2721=CARTESIAN_POINT ( 'NONE',  ( -2.426778023690262742, 214.6231898156240163, 85.10113791807857808 ) ) ;
#2723=CARTESIAN_POINT ( 'NONE',  ( -0.05014649552828403384, 217.5146222423826714, 51.24886208192143755 ) ) ;
#2727=CARTESIAN_POINT ( 'NONE',  ( 9.736236675708031640, 199.9851607334238963, 55.29886208192143471 ) ) ;
#2734=CARTESIAN_POINT ( 'NONE',  ( -2.426778023690262742, 214.6231898156240163, 46.10113791807857098 ) ) ;
#2737=CARTESIAN_POINT ( 'NONE',  ( 8.062137200540822946, 212.9164362838583315, 18.69886208192143329 ) ) ;
#2743=CARTESIAN_POINT ( 'NONE',  ( -6.444103211790928043, 202.2591342207265939, 5.198862081921435063 ) ) ;
#2744=CARTESIAN_POINT ( 'NONE',  ( -8.062137200540920645, 212.9164362838581894, 42.80113791807857382 ) ) ;
#2746=CARTESIAN_POINT ( 'NONE',  ( -0.05014649552810635652, 196.4853777576173002, 26.75113791807856956 ) ) ;
#2747=CARTESIAN_POINT ( 'NONE',  ( 8.118202686958138514, 201.1607312380088501, 103.2988620819214418 ) ) ;
#2749=CARTESIAN_POINT ( 'NONE',  ( -2.517493886309087880, 214.5937144450984135, 90.09886208192143897 ) ) ;
#2752=CARTESIAN_POINT ( 'NONE',  ( -12.01549611932652972, 203.1486557965464499, 12.35113791807856565 ) ) ;
#2755=CARTESIAN_POINT ( 'NONE',  ( 10.01549611932653860, 210.2015048109876716, 55.85113791807857808 ) ) ;
#2758=CARTESIAN_POINT ( 'NONE',  ( 10.01549611932659367, 203.7984951890124421, 1.148862081921434131 ) ) ;
#2761=CARTESIAN_POINT ( 'NONE',  ( 3.753561863808689836, 218.3979405102790565, 34.40113791807856813 ) ) ;
#2763=CARTESIAN_POINT ( 'NONE',  ( 6.139770520408223575, 215.5359834540460611, 12.54886208192143648 ) ) ;
#2767=CARTESIAN_POINT ( 'NONE',  ( 8.118202686958039038, 212.8392687619912635, 73.70113791807857240 ) ) ;
#2769=CARTESIAN_POINT ( 'NONE',  ( -4.903702542908436435, 200.1653181626580249, 29.04886208192143471 ) ) ;
#2772=CARTESIAN_POINT ( 'NONE',  ( 0.05014649552807626948, 215.4116977939061144, 13.25113791807856423 ) ) ;
#2773=CARTESIAN_POINT ( 'NONE',  ( -0.05014649552828442242, 219.6175466908591716, 99.24886208192143044 ) ) ;
#2779=CARTESIAN_POINT ( 'NONE',  ( -8.118202686958039038, 201.1607312380087080, 6.201137918078566180 ) ) ;
#2780=CARTESIAN_POINT ( 'NONE',  ( -8.118202686958138514, 212.8392687619910930, 77.79886208192144181 ) ) ;
#2783=CARTESIAN_POINT ( 'NONE',  ( -8.118202686958039038, 201.1607312380087080, 12.20113791807856707 ) ) ;
#2788=CARTESIAN_POINT ( 'NONE',  ( 6.220909254589536808, 215.4770327129947702, 88.55113791807853829 ) ) ;
#2791=CARTESIAN_POINT ( 'NONE',  ( -9.680171189290716072, 199.9079932115567146, 95.19886208192144750 ) ) ;
#2796=CARTESIAN_POINT ( 'NONE',  ( -0.05014649552807705357, 194.3824533091408000, 92.75113791807858377 ) ) ;
#2799=CARTESIAN_POINT ( 'NONE',  ( -6.220909254589682469, 215.4770327129947134, 98.94886208192143329 ) ) ;
#2800=CARTESIAN_POINT ( 'NONE',  ( 0.05014649552828288198, 194.3824533091408000, 22.74886208192143755 ) ) ;
#2802=CARTESIAN_POINT ( 'NONE',  ( -6.139770520408369237, 215.5359834540460042, 39.95113791807857240 ) ) ;
#2804=CARTESIAN_POINT ( 'NONE',  ( -2.517493886309087880, 214.5937144450984135, 3.098862081921434974 ) ) ;
#2807=CARTESIAN_POINT ( 'NONE',  ( -6.500168698208244500, 211.6636982574061676, 92.79886208192142760 ) ) ;
#2809=CARTESIAN_POINT ( 'NONE',  ( 8.015496119326531499, 209.5516654185219636, 28.85113791807856032 ) ) ;
#2815=CARTESIAN_POINT ( 'NONE',  ( 2.517493886308900919, 214.5937144450984420, 85.40113791807856103 ) ) ;
#2818=CARTESIAN_POINT ( 'NONE',  ( -8.000000000000008882, 206.9523078486584780, 59.49886208192144466 ) ) ;
#2821=CARTESIAN_POINT ( 'NONE',  ( 3.044812012440130555, 197.4746971517856764, 5.601137918078566535 ) ) ;
#2825=CARTESIAN_POINT ( 'NONE',  ( 0.05014649552807549926, 219.6175466908591716, 70.25113791807856956 ) ) ;
#2827=CARTESIAN_POINT ( 'NONE',  ( 6.139770520408367460, 198.4640165459539389, 83.45113791807858661 ) ) ;
#2829=CARTESIAN_POINT ( 'NONE',  ( -11.98450388067341876, 203.0532714938636047, 56.34886208192143187 ) ) ;
#2830=CARTESIAN_POINT ( 'NONE',  ( -9.984503880673420539, 203.7031108863293980, 56.34886208192142476 ) ) ;
#2831=CARTESIAN_POINT ( 'NONE',  ( -0.05014649552807705357, 194.3824533091408000, 95.75113791807856956 ) ) ;
#2833=CARTESIAN_POINT ( 'NONE',  ( 9.984503880673470277, 203.7031108863295401, 11.15113791807856636 ) ) ;
#2834=CARTESIAN_POINT ( 'NONE',  ( 8.118202686958138514, 201.1607312380088501, 76.29886208192144181 ) ) ;
#2836=CARTESIAN_POINT ( 'NONE',  ( 9.984503880673470277, 203.7031108863295401, 98.15113791807858945 ) ) ;
#2839=CARTESIAN_POINT ( 'NONE',  ( 7.984503880673422316, 209.6470497212048372, 57.84886208192144608 ) ) ;
#2849=CARTESIAN_POINT ( 'NONE',  ( -4.984841277089726574, 200.2242689037092305, 57.05113791807856671 ) ) ;
#2851=CARTESIAN_POINT ( 'NONE',  ( -8.118202686958138514, 212.8392687619910930, 47.79886208192143471 ) ) ;
#2852=CARTESIAN_POINT ( 'NONE',  ( -9.297231092197758784, 206.2510696422452838, 104.2062683007240338 ) ) ;
#2855=CARTESIAN_POINT ( 'NONE',  ( -6.444103211790928043, 202.2591342207265939, 35.19886208192144039 ) ) ;
#2856=CARTESIAN_POINT ( 'NONE',  ( 0.05014649552810505201, 217.5146222423826714, 82.25113791807858377 ) ) ;
#2858=CARTESIAN_POINT ( 'NONE',  ( 0.05014649552810505201, 217.5146222423826714, 58.25113791807856245 ) ) ;
#2860=CARTESIAN_POINT ( 'NONE',  ( -3.135527875058821579, 197.5041725223112223, 23.90113791807856813 ) ) ;
#2861=CARTESIAN_POINT ( 'NONE',  ( -6.500168698208129925, 202.3363017425936050, 15.20113791807857062 ) ) ;
#2865=CARTESIAN_POINT ( 'NONE',  ( -9.680171189290831535, 214.0920067884431148, 42.80113791807857382 ) ) ;
#2867=CARTESIAN_POINT ( 'NONE',  ( -3.135527875058821579, 197.5041725223112223, 86.90113791807857524 ) ) ;
#2868=CARTESIAN_POINT ( 'NONE',  ( 8.118202686958039038, 212.8392687619912635, 58.70113791807857240 ) ) ;
#2869=CARTESIAN_POINT ( 'NONE',  ( 12.00000000000000711, 207.0476921513415220, 24.99886208192143400 ) ) ;
#2870=CARTESIAN_POINT ( 'NONE',  ( -10.00000000000000711, 206.9523078486584495, 32.49886208192143044 ) ) ;
#2873=CARTESIAN_POINT ( 'NONE',  ( -9.736236675707914401, 199.9851607334237542, 69.20113791807857240 ) ) ;
#2874=CARTESIAN_POINT ( 'NONE',  ( -6.500168698208129925, 202.3363017425936050, 90.20113791807857240 ) ) ;
#2877=CARTESIAN_POINT ( 'NONE',  ( -9.984503880673420539, 203.7031108863293980, 53.34886208192143897 ) ) ;
#2880=CARTESIAN_POINT ( 'NONE',  ( -0.05014649552828442242, 219.6175466908591716, 48.24886208192144466 ) ) ;
#2886=CARTESIAN_POINT ( 'NONE',  ( 2.517493886308900919, 214.5937144450984420, 46.40113791807856813 ) ) ;
#2887=CARTESIAN_POINT ( 'NONE',  ( 10.00000000000000711, 207.0476921513415220, 27.99886208192143755 ) ) ;
#2890=DIRECTION ( 'NONE',  ( -6.106226635438360972E-16, 0.04769215134144213358, -0.9988620819214358848 ) ) ;
#2893=CARTESIAN_POINT ( 'NONE',  ( 8.015496119326595448, 204.4483345814782638, 1.148862081921434797 ) ) ;
#2895=CARTESIAN_POINT ( 'NONE',  ( 10.00000000000000711, 206.9523078486586201, 56.00113791807856956 ) ) ;
#2898=CARTESIAN_POINT ( 'NONE',  ( 9.984503880673470277, 203.7031108863295401, 32.15113791807857524 ) ) ;
#2902=CARTESIAN_POINT ( 'NONE',  ( -0.05014649552828365914, 215.4116977939061144, 90.24886208192144466 ) ) ;
#2906=CARTESIAN_POINT ( 'NONE',  ( 12.00000000000000711, 206.9523078486586485, 8.001137918078566003 ) ) ;
#2910=CARTESIAN_POINT ( 'NONE',  ( -6.220909254589537696, 198.5229672870051161, 60.05113791807855961 ) ) ;
#2911=CARTESIAN_POINT ( 'NONE',  ( 10.00000000000000711, 206.9523078486586201, 32.00113791807856956 ) ) ;
#2918=CARTESIAN_POINT ( 'NONE',  ( 0.05014649552807549926, 219.6175466908591716, 43.25113791807856245 ) ) ;
#2921=CARTESIAN_POINT ( 'NONE',  ( -0.05014649552828403384, 217.5146222423826714, 21.24886208192143400 ) ) ;
#2925=CARTESIAN_POINT ( 'NONE',  ( -0.05014649552810635652, 196.4853777576173002, 71.75113791807858377 ) ) ;
#2929=DIRECTION ( 'NONE',  ( -0.9891821073486152249, -0.1466927349985424900, -2.962715634069391535E-17 ) ) ;
#2932=CARTESIAN_POINT ( 'NONE',  ( 2.517493886308900919, 214.5937144450984420, 13.40113791807856636 ) ) ;
#2933=CARTESIAN_POINT ( 'NONE',  ( 9.736236675708031640, 199.9851607334238963, 100.2988620819214276 ) ) ;
#2938=CARTESIAN_POINT ( 'NONE',  ( -0.05014649552810635652, 196.4853777576173002, 8.751137918078562450 ) ) ;
#2940=CARTESIAN_POINT ( 'NONE',  ( -6.220909254589682469, 215.4770327129946850, 80.94886208192143329 ) ) ;
#2943=CARTESIAN_POINT ( 'NONE',  ( -3.135527875058821579, 197.5041725223112223, 8.901137918078566358 ) ) ;
#2949=CARTESIAN_POINT ( 'NONE',  ( 9.984503880673470277, 203.7031108863295401, 95.15113791807854682 ) ) ;
#2951=CARTESIAN_POINT ( 'NONE',  ( -6.220909254589537696, 198.5229672870051161, 84.05113791807855250 ) ) ;
#2956=CARTESIAN_POINT ( 'NONE',  ( 0.05014649552828288198, 194.3824533091408000, 97.74886208192141623 ) ) ;
#2961=CARTESIAN_POINT ( 'NONE',  ( 11.98450388067341876, 210.9467285061363953, 3.848862081921433642 ) ) ;
#2964=COLOUR_RGB ( '', 0.08235294, 0.09019608, 0.10196078) ;
#2965=CARTESIAN_POINT ( 'NONE',  ( -6.220909254589682469, 215.4770327129947134, 92.94886208192143329 ) ) ;
#2966=CARTESIAN_POINT ( 'NONE',  ( 0.05014649552828288198, 194.3824533091408000, 31.74886208192143755 ) ) ;
#2968=CARTESIAN_POINT ( 'NONE',  ( 3.044812012440130555, 197.4746971517856764, 41.60113791807857808 ) ) ;
#2970=CARTESIAN_POINT ( 'NONE',  ( 4.984841277089891776, 200.2242689037093726, 4.448862081921435063 ) ) ;
#2974=CARTESIAN_POINT ( 'NONE',  ( 4.984841277089891776, 200.2242689037093726, 94.44886208192143329 ) ) ;
#2975=CARTESIAN_POINT ( 'NONE',  ( 8.000000000000008882, 206.9523078486586485, 32.00113791807856956 ) ) ;
#2981=CARTESIAN_POINT ( 'NONE',  ( -4.903702542908602524, 213.8346818373418898, 87.95113791807857240 ) ) ;
#2983=CARTESIAN_POINT ( 'NONE',  ( 2.426778023690075337, 214.6231898156240447, 63.39886208192144323 ) ) ;
#2986=CARTESIAN_POINT ( 'NONE',  ( -3.135527875058821579, 197.5041725223112223, 8.901137918078566358 ) ) ;
#2990=CARTESIAN_POINT ( 'NONE',  ( -3.662846001190052991, 218.4274158808045740, 76.10113791807854966 ) ) ;
#2993=CARTESIAN_POINT ( 'NONE',  ( 9.984503880673473830, 203.7031108863295401, 86.15113791807857524 ) ) ;
#2996=CARTESIAN_POINT ( 'NONE',  ( -3.662846001189865142, 195.5725841191952838, 55.89886208192143613 ) ) ;
#2997=CARTESIAN_POINT ( 'NONE',  ( 8.118202686958138514, 201.1607312380088501, 64.29886208192144181 ) ) ;
#2998=CARTESIAN_POINT ( 'NONE',  ( 11.98450388067348271, 203.0532714938637753, 95.15113791807856103 ) ) ;
#3000=CARTESIAN_POINT ( 'NONE',  ( -8.118202686958039038, 201.1607312380087080, 15.20113791807856884 ) ) ;
#3001=CARTESIAN_POINT ( 'NONE',  ( -0.05014649552828403384, 217.5146222423826714, 81.24886208192140202 ) ) ;
#3003=CARTESIAN_POINT ( 'NONE',  ( -6.220909254589537696, 198.5229672870051161, 96.05113791807858092 ) ) ;
#3006=CARTESIAN_POINT ( 'NONE',  ( 2.426778023690075337, 214.6231898156240447, 66.39886208192143613 ) ) ;
#3012=CARTESIAN_POINT ( 'NONE',  ( 0.05014649552807626948, 215.4116977939061144, 58.25113791807857666 ) ) ;
#3016=CARTESIAN_POINT ( 'NONE',  ( 6.500168698208244500, 202.3363017425938324, 37.29886208192144181 ) ) ;
#3017=CARTESIAN_POINT ( 'NONE',  ( -9.984503880673473830, 210.2968891136704315, 78.65113791807854682 ) ) ;
#3019=CARTESIAN_POINT ( 'NONE',  ( -3.044812012440131443, 216.5253028482142952, 67.10113791807857808 ) ) ;
#3020=CARTESIAN_POINT ( 'NONE',  ( -10.01549611932653860, 203.7984951890123284, 30.35113791807856742 ) ) ;
#3021=CARTESIAN_POINT ( 'NONE',  ( 4.984841277089725686, 213.7757310962907411, 10.55113791807856671 ) ) ;
#3023=DIRECTION ( 'NONE',  ( 5.620504062164857944E-16, -0.9988620819214347746, 0.04769215134146256169 ) ) ;
#3025=CARTESIAN_POINT ( 'NONE',  ( 3.662846001190051659, 195.5725841191953691, 41.60113791807857098 ) ) ;
#3027=CARTESIAN_POINT ( 'NONE',  ( 10.00000000000000711, 206.9523078486586201, 92.00113791807858377 ) ) ;
#3029=CARTESIAN_POINT ( 'NONE',  ( 6.220909254589536808, 215.4770327129947987, 61.55113791807857382 ) ) ;
#3030=CARTESIAN_POINT ( 'NONE',  ( 12.00000000000000711, 207.0476921513415220, 21.99886208192143400 ) ) ;
#3031=CARTESIAN_POINT ( 'NONE',  ( -8.062137200540822946, 201.0835637161416400, 41.19886208192144039 ) ) ;
#3033=CARTESIAN_POINT ( 'NONE',  ( 7.375838497908181246, 196.7627149292499666, 68.45113791807857240 ) ) ;
#3034=CARTESIAN_POINT ( 'NONE',  ( 4.984841277089725686, 213.7757310962907411, 91.55113791807858092 ) ) ;
#3036=CARTESIAN_POINT ( 'NONE',  ( 10.00000000000000711, 207.0476921513415220, 54.99886208192143755 ) ) ;
#3039=CARTESIAN_POINT ( 'NONE',  ( 7.456977232089471386, 196.8216656703012006, 55.44886208192143329 ) ) ;
#3046=CARTESIAN_POINT ( 'NONE',  ( -8.015496119326531499, 204.4483345814780364, 39.35113791807857098 ) ) ;
#3047=CARTESIAN_POINT ( 'NONE',  ( -6.139770520408224463, 198.4640165459539389, 20.04886208192142760 ) ) ;
#3052=CARTESIAN_POINT ( 'NONE',  ( 8.015496119326595448, 204.4483345814782638, 7.148862081921435241 ) ) ;
#3054=CARTESIAN_POINT ( 'NONE',  ( 3.135527875058820690, 216.4958274776887492, 49.40113791807857524 ) ) ;
#3056=CARTESIAN_POINT ( 'NONE',  ( 3.135527875058820690, 216.4958274776887492, 25.40113791807856813 ) ) ;
#3059=CARTESIAN_POINT ( 'NONE',  ( 2.517493886309087436, 199.4062855549015865, 94.59886208192145318 ) ) ;
#3062=DIRECTION ( 'NONE',  ( 5.170793409489829447E-18, -0.9988620819214357738, 0.04769215134144141888 ) ) ;
#3063=CARTESIAN_POINT ( 'NONE',  ( -9.736236675707914401, 199.9851607334237542, 9.201137918078563516 ) ) ;
#3066=CARTESIAN_POINT ( 'NONE',  ( 8.118202686958039038, 212.8392687619912635, 58.70113791807857240 ) ) ;
#3068=CARTESIAN_POINT ( 'NONE',  ( 3.135527875058820690, 216.4958274776887492, 28.40113791807856813 ) ) ;
#3076=CARTESIAN_POINT ( 'NONE',  ( 3.662846001190051659, 195.5725841191953691, 35.60113791807855677 ) ) ;
#3078=CARTESIAN_POINT ( 'NONE',  ( -9.984503880673420539, 203.7031108863293980, 20.34886208192143187 ) ) ;
#3083=CARTESIAN_POINT ( 'NONE',  ( 6.139770520408368348, 198.4640165459539674, 80.45113791807857240 ) ) ;
#3088=CARTESIAN_POINT ( 'NONE',  ( -6.444103211791042618, 211.7408657792732356, 12.80113791807856849 ) ) ;
#3090=CARTESIAN_POINT ( 'NONE',  ( -3.662846001189865142, 195.5725841191952838, 94.89886208192145034 ) ) ;
#3097=CARTESIAN_POINT ( 'NONE',  ( 3.044812012439969795, 216.5253028482143520, 84.39886208192143613 ) ) ;
#3100=CARTESIAN_POINT ( 'NONE',  ( -3.135527875058821579, 197.5041725223112223, 20.90113791807856813 ) ) ;
#3106=CARTESIAN_POINT ( 'NONE',  ( -6.139770520408369237, 215.5359834540460042, 84.95113791807858661 ) ) ;
#3109=CARTESIAN_POINT ( 'NONE',  ( -7.456977232089471386, 217.1783343296987709, 95.94886208192144750 ) ) ;
#3120=CARTESIAN_POINT ( 'NONE',  ( 6.220909254589680693, 198.5229672870052582, 94.44886208192141908 ) ) ;
#3121=CARTESIAN_POINT ( 'NONE',  ( -7.456977232089471386, 217.1783343296987709, 35.94886208192142618 ) ) ;
#3123=CARTESIAN_POINT ( 'NONE',  ( 10.01549611932653860, 210.2015048109876716, 37.85113791807854966 ) ) ;
#3125=CARTESIAN_POINT ( 'NONE',  ( 7.984503880673422316, 209.6470497212048372, 6.848862081921435419 ) ) ;
#3131=CARTESIAN_POINT ( 'NONE',  ( -2.426778023690076225, 199.3768101843759553, 94.89886208192145034 ) ) ;
#3134=CARTESIAN_POINT ( 'NONE',  ( 6.500168698208129925, 211.6636982574063381, 28.70113791807857240 ) ) ;
#3142=CARTESIAN_POINT ( 'NONE',  ( 7.984503880673485376, 204.3529502787953902, 101.1511379180785895 ) ) ;
#3144=CARTESIAN_POINT ( 'NONE',  ( -8.015496119326597224, 209.5516654185217362, 74.64886208192143613 ) ) ;
#3148=CARTESIAN_POINT ( 'NONE',  ( -8.062137200540920645, 212.9164362838581894, 9.801137918078566713 ) ) ;
#3153=CARTESIAN_POINT ( 'NONE',  ( -7.456977232089304408, 196.8216656703010301, 78.05113791807858092 ) ) ;
#3155=CARTESIAN_POINT ( 'NONE',  ( -10.00000000000000711, 207.0476921513413515, 99.50113791807856956 ) ) ;
#3158=CARTESIAN_POINT ( 'NONE',  ( -0.05014649552828442242, 219.6175466908591716, 66.24886208192143044 ) ) ;
#3159=CARTESIAN_POINT ( 'NONE',  ( -8.118202686958138514, 212.8392687619910930, 68.79886208192144181 ) ) ;
#3160=CARTESIAN_POINT ( 'NONE',  ( 0.05014649552828288198, 194.3824533091408000, 4.748862081921433109 ) ) ;
#3163=CARTESIAN_POINT ( 'NONE',  ( 3.044812012440130555, 197.4746971517856764, 17.60113791807856742 ) ) ;
#3164=CARTESIAN_POINT ( 'NONE',  ( -3.044812012439970683, 197.4746971517856196, 82.89886208192145034 ) ) ;
#3167=CARTESIAN_POINT ( 'NONE',  ( -3.135527875058821579, 197.5041725223112223, 101.9011379180785752 ) ) ;
#3170=CARTESIAN_POINT ( 'NONE',  ( 8.000000000000008882, 207.0476921513415220, 57.99886208192144466 ) ) ;
#3172=CIRCLE ( 'NONE', #26045, 3.999999999999996003 ) ;
#3178=CARTESIAN_POINT ( 'NONE',  ( 2.426778023690261410, 199.3768101843759837, 59.60113791807857808 ) ) ;
#3179=CARTESIAN_POINT ( 'NONE',  ( -9.000000000000001776, 206.9999999999998863, 103.5000000000000426 ) ) ;
#3181=CARTESIAN_POINT ( 'NONE',  ( -6.444103211790928043, 202.2591342207265939, 41.19886208192144750 ) ) ;
#3183=CARTESIAN_POINT ( 'NONE',  ( -10.00000000000000711, 207.0476921513413515, 81.50113791807856956 ) ) ;
#3185=CARTESIAN_POINT ( 'NONE',  ( 8.062137200540920645, 201.0835637161417822, 65.30113791807858092 ) ) ;
#3189=CARTESIAN_POINT ( 'NONE',  ( 2.517493886308900919, 214.5937144450984420, 19.40113791807856813 ) ) ;
#3193=CARTESIAN_POINT ( 'NONE',  ( 12.01549611932652972, 210.8513442034534933, 43.85113791807856387 ) ) ;
#3195=CARTESIAN_POINT ( 'NONE',  ( 9.984503880673470277, 203.7031108863295401, 92.15113791807856103 ) ) ;
#3196=CARTESIAN_POINT ( 'NONE',  ( -6.220909254589537696, 198.5229672870051445, 66.05113791807858092 ) ) ;
#3198=CARTESIAN_POINT ( 'NONE',  ( -9.736236675708031640, 214.0148392665760753, 29.79886208192143826 ) ) ;
#3199=CARTESIAN_POINT ( 'NONE',  ( -6.139770520408224463, 198.4640165459539105, 41.04886208192143471 ) ) ;
#3201=CARTESIAN_POINT ( 'NONE',  ( -0.05014649552807705357, 194.3824533091408000, 74.75113791807856956 ) ) ;
#3202=CARTESIAN_POINT ( 'NONE',  ( 4.984841277089725686, 213.7757310962907411, 85.55113791807858092 ) ) ;
#3203=CARTESIAN_POINT ( 'NONE',  ( -9.984503880673420539, 203.7031108863293980, 47.34886208192143187 ) ) ;
#3206=CARTESIAN_POINT ( 'NONE',  ( 12.00000000000000711, 207.0476921513415220, 51.99886208192143044 ) ) ;
#3213=CARTESIAN_POINT ( 'NONE',  ( 8.000000000000008882, 206.9523078486586485, 56.00113791807857666 ) ) ;
#3215=CARTESIAN_POINT ( 'NONE',  ( -0.05014649552828403384, 217.5146222423826714, 33.24886208192142334 ) ) ;
#3220=CARTESIAN_POINT ( 'NONE',  ( -2.426778023690076225, 199.3768101843759553, 1.898862081921434797 ) ) ;
#3221=CARTESIAN_POINT ( 'NONE',  ( -8.062137200540920645, 212.9164362838581894, 54.80113791807857382 ) ) ;
#3223=CARTESIAN_POINT ( 'NONE',  ( 0.05014649552810505201, 217.5146222423826714, 40.25113791807856956 ) ) ;
#3225=CARTESIAN_POINT ( 'NONE',  ( -4.903702542908436435, 200.1653181626580249, 89.04886208192142760 ) ) ;
#3229=CARTESIAN_POINT ( 'NONE',  ( -9.736236675707914401, 199.9851607334237542, 24.20113791807856529 ) ) ;
#3233=CARTESIAN_POINT ( 'NONE',  ( 3.135527875058820690, 216.4958274776887492, 67.40113791807857524 ) ) ;
#3234=CARTESIAN_POINT ( 'NONE',  ( -3.135527875058821579, 197.5041725223112223, 29.90113791807856813 ) ) ;
#3237=CARTESIAN_POINT ( 'NONE',  ( -6.220909254589682469, 215.4770327129947134, 11.94886208192143684 ) ) ;
#3240=CARTESIAN_POINT ( 'NONE',  ( -3.753561863808691168, 195.6020594897209435, 38.90113791807856813 ) ) ;
#3242=CARTESIAN_POINT ( 'NONE',  ( 6.139770520408223575, 215.5359834540460611, 18.54886208192143826 ) ) ;
#3245=CARTESIAN_POINT ( 'NONE',  ( -3.135527875058821579, 197.5041725223112223, 83.90113791807857524 ) ) ;
#3250=CARTESIAN_POINT ( 'NONE',  ( -8.000000000000008882, 207.0476921513413515, 27.50113791807856956 ) ) ;
#3253=CARTESIAN_POINT ( 'NONE',  ( 9.984503880673420539, 210.2968891136705167, 6.848862081921434530 ) ) ;
#3260=CARTESIAN_POINT ( 'NONE',  ( 6.139770520408223575, 215.5359834540460611, 78.54886208192144181 ) ) ;
#3262=CARTESIAN_POINT ( 'NONE',  ( -0.05014649552810635652, 196.4853777576173002, 23.75113791807855890 ) ) ;
#3264=CARTESIAN_POINT ( 'NONE',  ( 0.05014649552828288198, 194.3824533091408000, 82.74886208192144466 ) ) ;
#3269=CARTESIAN_POINT ( 'NONE',  ( -10.00000000000000711, 207.0476921513413515, 81.50113791807856956 ) ) ;
#3272=CARTESIAN_POINT ( 'NONE',  ( -10.01549611932653860, 203.7984951890123284, 39.35113791807857098 ) ) ;
#3277=CARTESIAN_POINT ( 'NONE',  ( -7.456977232089304408, 196.8216656703010301, 6.051137918078566713 ) ) ;
#3283=CARTESIAN_POINT ( 'NONE',  ( 3.044812012439969795, 216.5253028482143520, 96.39886208192145034 ) ) ;
#3284=CARTESIAN_POINT ( 'NONE',  ( 12.01549611932659367, 203.1486557965466773, 31.14886208192143968 ) ) ;
#3286=CARTESIAN_POINT ( 'NONE',  ( -0.05014649552810635652, 196.4853777576173002, 53.75113791807857666 ) ) ;
#3289=CARTESIAN_POINT ( 'NONE',  ( 6.444103211790928043, 211.7408657792734061, 15.69886208192143684 ) ) ;
#3293=CARTESIAN_POINT ( 'NONE',  ( -4.903702542908436435, 200.1653181626580249, 89.04886208192142760 ) ) ;
#3294=CARTESIAN_POINT ( 'NONE',  ( 2.426778023690261410, 199.3768101843759837, 26.60113791807856742 ) ) ;
#3300=CARTESIAN_POINT ( 'NONE',  ( 4.984841277089725686, 213.7757310962907411, 100.5511379180785809 ) ) ;
#3303=CARTESIAN_POINT ( 'NONE',  ( 6.500168698208244500, 202.3363017425938324, 76.29886208192142760 ) ) ;
#3307=CARTESIAN_POINT ( 'NONE',  ( -3.044812012440131443, 216.5253028482142952, 7.101137918078566535 ) ) ;
#3312=CARTESIAN_POINT ( 'NONE',  ( -9.736236675707914401, 199.9851607334237542, 75.20113791807857240 ) ) ;
#3315=CARTESIAN_POINT ( 'NONE',  ( 0.05014649552810506589, 217.5146222423826714, 100.2511379180785696 ) ) ;
#3318=CARTESIAN_POINT ( 'NONE',  ( 0.05014649552828288198, 194.3824533091408000, 103.7488620819214304 ) ) ;
#3319=CARTESIAN_POINT ( 'NONE',  ( 9.736236675708031640, 199.9851607334238963, 58.29886208192143471 ) ) ;
#3320=CARTESIAN_POINT ( 'NONE',  ( 9.984503880673420539, 210.2968891136705736, 69.84886208192143897 ) ) ;
#3321=CARTESIAN_POINT ( 'NONE',  ( -12.01549611932652972, 203.1486557965464499, 102.3511379180785639 ) ) ;
#3323=CARTESIAN_POINT ( 'NONE',  ( 10.01549611932653860, 210.2015048109876716, 25.85113791807856742 ) ) ;
#3325=CARTESIAN_POINT ( 'NONE',  ( 10.00000000000000711, 207.0476921513415220, 75.99886208192144466 ) ) ;
#3327=CARTESIAN_POINT ( 'NONE',  ( -10.01549611932653860, 203.7984951890123284, 99.35113791807857808 ) ) ;
#3330=CARTESIAN_POINT ( 'NONE',  ( -6.500168698208244500, 211.6636982574061676, 59.79886208192143471 ) ) ;
#3334=CYLINDRICAL_SURFACE ( 'NONE', #3651, 1.000000000000000222 ) ;
#3338=CARTESIAN_POINT ( 'NONE',  ( 6.500168698208129925, 211.6636982574063381, 73.70113791807857240 ) ) ;
#3342=CARTESIAN_POINT ( 'NONE',  ( 7.984503880673422316, 209.6470497212048372, 42.84886208192143897 ) ) ;
#3343=CARTESIAN_POINT ( 'NONE',  ( -6.139770520408369237, 215.5359834540460042, 75.95113791807857240 ) ) ;
#3344=CARTESIAN_POINT ( 'NONE',  ( 10.00000000000000711, 206.9523078486586201, 65.00113791807856956 ) ) ;
#3347=CARTESIAN_POINT ( 'NONE',  ( 0.05014649552807626948, 215.4116977939061144, 22.25113791807856956 ) ) ;
#3351=CARTESIAN_POINT ( 'NONE',  ( -3.753561863808691168, 195.6020594897209435, 50.90113791807858235 ) ) ;
#3353=CARTESIAN_POINT ( 'NONE',  ( -8.118202686958039038, 201.1607312380087080, 93.20113791807857240 ) ) ;
#3355=CARTESIAN_POINT ( 'NONE',  ( 8.118202686958039038, 212.8392687619912635, 67.70113791807858661 ) ) ;
#3356=CARTESIAN_POINT ( 'NONE',  ( 12.01549611932659367, 203.1486557965466773, 31.14886208192143968 ) ) ;
#3357=CARTESIAN_POINT ( 'NONE',  ( 10.00000000000000711, 207.0476921513415220, 33.99886208192143044 ) ) ;
#3360=CARTESIAN_POINT ( 'NONE',  ( 3.753561863808689836, 218.3979405102790565, 73.40113791807856103 ) ) ;
#3361=CARTESIAN_POINT ( 'NONE',  ( -2.426778023690262742, 214.6231898156240163, 88.10113791807857808 ) ) ;
#3362=CARTESIAN_POINT ( 'NONE',  ( 8.118202686958138514, 201.1607312380088501, 52.29886208192143471 ) ) ;
#3364=EDGE_LOOP ( 'NONE', ( #33433, #32436, #8382, #28584, #8212, #13173, #31098 ) ) ;
#3365=CARTESIAN_POINT ( 'NONE',  ( -7.456977232089471386, 217.1783343296987709, 59.94886208192143329 ) ) ;
#3368=CARTESIAN_POINT ( 'NONE',  ( 4.984841277089891776, 200.2242689037093726, 37.44886208192144039 ) ) ;
#3373=CARTESIAN_POINT ( 'NONE',  ( 8.015496119326531499, 209.5516654185219636, 52.85113791807857098 ) ) ;
#3375=CARTESIAN_POINT ( 'NONE',  ( -8.118202686958138514, 212.8392687619910930, 35.79886208192143471 ) ) ;
#3381=CARTESIAN_POINT ( 'NONE',  ( 8.015496119326595448, 204.4483345814782638, 13.14886208192143613 ) ) ;
#3382=CARTESIAN_POINT ( 'NONE',  ( 10.01549611932653860, 210.2015048109876716, 49.85113791807857808 ) ) ;
#3384=CARTESIAN_POINT ( 'NONE',  ( 8.118202686958039038, 212.8392687619912635, 40.70113791807857240 ) ) ;
#3387=CARTESIAN_POINT ( 'NONE',  ( 2.426778023690075337, 214.6231898156240447, 102.3988620819214361 ) ) ;
#3392=CARTESIAN_POINT ( 'NONE',  ( 3.662846001190051659, 195.5725841191953691, 20.60113791807856742 ) ) ;
#3396=CARTESIAN_POINT ( 'NONE',  ( -8.118202686958039038, 201.1607312380087080, 63.20113791807857240 ) ) ;
#3397=CARTESIAN_POINT ( 'NONE',  ( -0.05014649552810635652, 196.4853777576173002, 35.75113791807857666 ) ) ;
#3400=CARTESIAN_POINT ( 'NONE',  ( -6.220909254589682469, 215.4770327129947134, 8.948862081921435063 ) ) ;
#3403=CARTESIAN_POINT ( 'NONE',  ( -11.98450388067348804, 210.9467285061362247, 51.65113791807857524 ) ) ;
#3405=CARTESIAN_POINT ( 'NONE',  ( -6.220909254589682469, 215.4770327129946850, 17.94886208192143684 ) ) ;
#3408=CARTESIAN_POINT ( 'NONE',  ( 10.01549611932653860, 210.2015048109876716, 79.85113791807853545 ) ) ;
#3412=ORIENTED_EDGE ( 'NONE', *, *, #18364, .F. ) ;
#3414=CARTESIAN_POINT ( 'NONE',  ( -4.984841277089726574, 200.2242689037092305, 24.05113791807857027 ) ) ;
#3417=CARTESIAN_POINT ( 'NONE',  ( 3.135527875058981895, 197.5041725223112792, 1.598862081921434530 ) ) ;
#3425=CARTESIAN_POINT ( 'NONE',  ( -0.05014649552828403384, 217.5146222423826714, 87.24886208192143044 ) ) ;
#3427=CARTESIAN_POINT ( 'NONE',  ( 10.00000000000000711, 206.9523078486586201, 20.00113791807856600 ) ) ;
#3429=CARTESIAN_POINT ( 'NONE',  ( -0.05014649552828442242, 219.6175466908591716, 75.24886208192143044 ) ) ;
#3434=CARTESIAN_POINT ( 'NONE',  ( 0.05014649552810505201, 217.5146222423826714, 91.25113791807858377 ) ) ;
#3437=CARTESIAN_POINT ( 'NONE',  ( 6.220909254589536808, 215.4770327129947702, 34.55113791807855250 ) ) ;
#3442=CARTESIAN_POINT ( 'NONE',  ( -9.680171189290831535, 214.0920067884431148, 15.80113791807856849 ) ) ;
#3449=CARTESIAN_POINT ( 'NONE',  ( -10.01549611932659545, 210.2015048109875011, 98.64886208192145034 ) ) ;
#3450=CARTESIAN_POINT ( 'NONE',  ( -3.662846001189865142, 195.5725841191952838, 34.89886208192143613 ) ) ;
#3452=CARTESIAN_POINT ( 'NONE',  ( -8.118202686958039038, 201.1607312380087080, 48.20113791807857950 ) ) ;
#3454=CARTESIAN_POINT ( 'NONE',  ( 8.015496119326595448, 204.4483345814782638, 16.14886208192143968 ) ) ;
#3458=CARTESIAN_POINT ( 'NONE',  ( -6.444103211790928043, 202.2591342207265939, 98.19886208192144750 ) ) ;
#3459=CARTESIAN_POINT ( 'NONE',  ( 2.426778023690261410, 199.3768101843759837, 35.60113791807857098 ) ) ;
#3464=CARTESIAN_POINT ( 'NONE',  ( -8.062137200540822946, 201.0835637161416400, 62.19886208192143329 ) ) ;
#3465=AXIS2_PLACEMENT_3D ( 'NONE', #8332, #16653, #29615 ) ;
#3468=CARTESIAN_POINT ( 'NONE',  ( 6.444103211791042618, 202.2591342207267644, 101.3011379180785951 ) ) ;
#3472=CARTESIAN_POINT ( 'NONE',  ( -6.444103211790928043, 202.2591342207265939, 71.19886208192144750 ) ) ;
#3477=CARTESIAN_POINT ( 'NONE',  ( -10.00000000000000711, 207.0476921513413515, 12.50113791807856778 ) ) ;
#3482=CARTESIAN_POINT ( 'NONE',  ( -3.753561863808691168, 195.6020594897209435, 80.90113791807858945 ) ) ;
#3483=CARTESIAN_POINT ( 'NONE',  ( -0.05014649552810635652, 196.4853777576173002, 101.7511379180785696 ) ) ;
#3487=CARTESIAN_POINT ( 'NONE',  ( 8.118202686958138514, 201.1607312380088501, 1.298862081921434486 ) ) ;
#3488=CARTESIAN_POINT ( 'NONE',  ( -9.680171189290716072, 199.9079932115567146, 65.19886208192143329 ) ) ;
#3489=CARTESIAN_POINT ( 'NONE',  ( 8.118202686958138514, 201.1607312380088501, 70.29886208192142760 ) ) ;
#3491=CARTESIAN_POINT ( 'NONE',  ( 11.98450388067341876, 210.9467285061363953, 6.848862081921435419 ) ) ;
#3493=CARTESIAN_POINT ( 'NONE',  ( 9.984503880673470277, 203.7031108863295401, 20.15113791807856813 ) ) ;
#3495=CARTESIAN_POINT ( 'NONE',  ( -6.220909254589682469, 215.4770327129946850, 86.94886208192141908 ) ) ;
#3501=CARTESIAN_POINT ( 'NONE',  ( -8.000000000000008882, 206.9523078486584780, 68.49886208192144466 ) ) ;
#3508=CARTESIAN_POINT ( 'NONE',  ( -7.984503880673488041, 209.6470497212046098, 69.65113791807856103 ) ) ;
#3512=CARTESIAN_POINT ( 'NONE',  ( 6.444103211790928043, 211.7408657792734061, 39.69886208192144750 ) ) ;
#3513=CARTESIAN_POINT ( 'NONE',  ( 3.044812012440130555, 197.4746971517856764, 83.60113791807857808 ) ) ;
#3514=CARTESIAN_POINT ( 'NONE',  ( -10.01549611932653860, 203.7984951890123284, 63.35113791807857098 ) ) ;
#3516=CARTESIAN_POINT ( 'NONE',  ( -8.000000000000008882, 207.0476921513413515, 24.50113791807856600 ) ) ;
#3520=CARTESIAN_POINT ( 'NONE',  ( -7.456977232089304408, 196.8216656703010301, 48.05113791807856671 ) ) ;
#3522=CARTESIAN_POINT ( 'NONE',  ( 8.062137200540920645, 201.0835637161417822, 92.30113791807858092 ) ) ;
#3523=CARTESIAN_POINT ( 'NONE',  ( 8.118202686958039038, 212.8392687619912635, 64.70113791807857240 ) ) ;
#3524=CARTESIAN_POINT ( 'NONE',  ( 7.375838497908012492, 217.2372850707501186, 36.54886208192144181 ) ) ;
#3525=CARTESIAN_POINT ( 'NONE',  ( 6.139770520408223575, 215.5359834540460611, 36.54886208192142760 ) ) ;
#3527=CARTESIAN_POINT ( 'NONE',  ( -3.753561863808691168, 195.6020594897209435, 80.90113791807858945 ) ) ;
#3528=CARTESIAN_POINT ( 'NONE',  ( 0.05014649552807626948, 215.4116977939061144, 100.2511379180785696 ) ) ;
#3529=CARTESIAN_POINT ( 'NONE',  ( -10.00000000000000711, 206.9523078486584495, 56.49886208192143755 ) ) ;
#3532=CARTESIAN_POINT ( 'NONE',  ( -12.00000000000000711, 206.9523078486584780, 62.49886208192143044 ) ) ;
#3534=CARTESIAN_POINT ( 'NONE',  ( -6.500168698208244500, 211.6636982574061676, 35.79886208192144181 ) ) ;
#3541=CARTESIAN_POINT ( 'NONE',  ( 6.444103211791042618, 202.2591342207267644, 50.30113791807858092 ) ) ;
#3545=CARTESIAN_POINT ( 'NONE',  ( -8.118202686958138514, 212.8392687619910930, 32.79886208192143471 ) ) ;
#3551=CARTESIAN_POINT ( 'NONE',  ( 4.903702542908435547, 213.8346818373419751, 12.54886208192143826 ) ) ;
#3553=CARTESIAN_POINT ( 'NONE',  ( -6.220909254589537696, 198.5229672870051161, 51.05113791807856671 ) ) ;
#3556=CARTESIAN_POINT ( 'NONE',  ( 0.05014649552810505201, 217.5146222423826714, 37.25113791807855534 ) ) ;
#3559=CARTESIAN_POINT ( 'NONE',  ( 0.05014649552828262524, 198.5883022060938572, 100.7488620819214304 ) ) ;
#3563=CARTESIAN_POINT ( 'NONE',  ( -9.680171189290831535, 214.0920067884431148, 21.80113791807856671 ) ) ;
#3566=CARTESIAN_POINT ( 'NONE',  ( 10.00000000000000711, 206.9523078486586201, 68.00113791807856956 ) ) ;
#3567=CARTESIAN_POINT ( 'NONE',  ( 10.00000000000000711, 206.9523078486586201, 41.00113791807856956 ) ) ;
#3570=CARTESIAN_POINT ( 'NONE',  ( -12.00000000000000711, 207.0476921513413515, 102.5011379180785696 ) ) ;
#3571=CARTESIAN_POINT ( 'NONE',  ( -8.062137200540822946, 201.0835637161416400, 11.19886208192143506 ) ) ;
#3574=CARTESIAN_POINT ( 'NONE',  ( -7.375838497908182134, 217.2372850707499765, 45.95113791807857950 ) ) ;
#3575=CARTESIAN_POINT ( 'NONE',  ( 2.426778023690261410, 199.3768101843759837, 65.60113791807857808 ) ) ;
#3577=CARTESIAN_POINT ( 'NONE',  ( 6.220909254589681581, 198.5229672870052582, 25.44886208192143684 ) ) ;
#3580=CARTESIAN_POINT ( 'NONE',  ( 3.044812012440130555, 197.4746971517856764, 83.60113791807857808 ) ) ;
#3585=CARTESIAN_POINT ( 'NONE',  ( 8.015496119326531499, 209.5516654185219636, 19.85113791807856387 ) ) ;
#3587=CARTESIAN_POINT ( 'NONE',  ( -8.062137200540822946, 201.0835637161416400, 2.198862081921434175 ) ) ;
#3594=CARTESIAN_POINT ( 'NONE',  ( -6.139770520408224463, 198.4640165459539389, 89.04886208192139918 ) ) ;
#3596=CARTESIAN_POINT ( 'NONE',  ( -8.118202686958039038, 201.1607312380087080, 27.20113791807856884 ) ) ;
#3598=CARTESIAN_POINT ( 'NONE',  ( -9.680171189290716072, 199.9079932115567146, 77.19886208192143329 ) ) ;
#3603=CARTESIAN_POINT ( 'NONE',  ( -10.01549611932653860, 203.7984951890123284, 96.35113791807853545 ) ) ;
#3606=CARTESIAN_POINT ( 'NONE',  ( -10.01549611932653860, 203.7984951890123284, 33.35113791807855677 ) ) ;
#3612=CARTESIAN_POINT ( 'NONE',  ( 9.680171189290831535, 199.9079932115568852, 17.30113791807856671 ) ) ;
#3616=CARTESIAN_POINT ( 'NONE',  ( 7.375838497908012492, 217.2372850707501186, 30.54886208192144181 ) ) ;
#3617=CARTESIAN_POINT ( 'NONE',  ( -10.16981089642701974, 207.8187771357854103, 102.5476305063704814 ) ) ;
#3618=CARTESIAN_POINT ( 'NONE',  ( -8.118202686958039038, 201.1607312380087080, 51.20113791807857240 ) ) ;
#3620=CARTESIAN_POINT ( 'NONE',  ( 2.426778023690075337, 214.6231898156240447, 15.39886208192143613 ) ) ;
#3625=CARTESIAN_POINT ( 'NONE',  ( 2.517493886309087436, 199.4062855549015865, 100.5988620819214532 ) ) ;
#3626=CARTESIAN_POINT ( 'NONE',  ( -2.426778023690262742, 214.6231898156240163, 43.10113791807857808 ) ) ;
#3631=CARTESIAN_POINT ( 'NONE',  ( 8.118202686958138514, 201.1607312380088501, 58.29886208192143471 ) ) ;
#3634=CARTESIAN_POINT ( 'NONE',  ( -6.500168698208129925, 202.3363017425936050, 99.20113791807858661 ) ) ;
#3637=CARTESIAN_POINT ( 'NONE',  ( 7.984503880673422316, 209.6470497212048372, 75.84886208192143897 ) ) ;
#3640=CARTESIAN_POINT ( 'NONE',  ( -10.00000000000000178, 206.7692714347156198, 108.3323677711372000 ) ) ;
#3644=CARTESIAN_POINT ( 'NONE',  ( 8.118202686958039038, 212.8392687619912635, 10.70113791807856529 ) ) ;
#3648=CARTESIAN_POINT ( 'NONE',  ( -3.753561863808691168, 195.6020594897209435, 74.90113791807856103 ) ) ;
#3649=CARTESIAN_POINT ( 'NONE',  ( -8.118202686958039038, 201.1607312380087080, 93.20113791807857240 ) ) ;
#3651=AXIS2_PLACEMENT_3D ( 'NONE', #13719, #16614, #32294 ) ;
#3653=CARTESIAN_POINT ( 'NONE',  ( -8.118202686958138514, 212.8392687619910930, 2.798862081921434708 ) ) ;
#3654=CARTESIAN_POINT ( 'NONE',  ( 3.662846001189864698, 218.4274158808046593, 66.39886208192143613 ) ) ;
#3655=CARTESIAN_POINT ( 'NONE',  ( -6.220909254589682469, 215.4770327129947134, 65.94886208192143329 ) ) ;
#3656=CARTESIAN_POINT ( 'NONE',  ( 9.736236675708031640, 199.9851607334238963, 4.298862081921434708 ) ) ;
#3658=CARTESIAN_POINT ( 'NONE',  ( -10.00000000000000711, 207.0476921513413515, 24.50113791807856600 ) ) ;
#3659=CARTESIAN_POINT ( 'NONE',  ( 8.062137200540822946, 212.9164362838583315, 90.69886208192143329 ) ) ;
#3664=CARTESIAN_POINT ( 'NONE',  ( 7.984503880673422316, 209.6470497212048372, 66.84886208192143897 ) ) ;
#3673=CARTESIAN_POINT ( 'NONE',  ( 6.444103211791042618, 202.2591342207267644, 65.30113791807858092 ) ) ;
#3678=CARTESIAN_POINT ( 'NONE',  ( -8.000000000000008882, 206.9523078486584780, 47.49886208192144466 ) ) ;
#3679=CARTESIAN_POINT ( 'NONE',  ( 0.05014649552810505201, 217.5146222423826714, 88.25113791807858377 ) ) ;
#3680=CARTESIAN_POINT ( 'NONE',  ( -10.01549611932653860, 203.7984951890123284, 66.35113791807853545 ) ) ;
#3683=CARTESIAN_POINT ( 'NONE',  ( 7.984503880673485376, 204.3529502787953902, 20.15113791807856458 ) ) ;
#3687=CARTESIAN_POINT ( 'NONE',  ( 3.753561863808689836, 218.3979405102790565, 52.40113791807858235 ) ) ;
#3691=CARTESIAN_POINT ( 'NONE',  ( -9.984503880673473830, 210.2968891136704315, 93.65113791807857524 ) ) ;
#3692=CARTESIAN_POINT ( 'NONE',  ( -10.01549611932653860, 203.7984951890123000, 66.35113791807856387 ) ) ;
#3695=CARTESIAN_POINT ( 'NONE',  ( 12.01549611932659367, 203.1486557965466773, 37.14886208192143613 ) ) ;
#3696=CARTESIAN_POINT ( 'NONE',  ( -10.01549611932659545, 210.2015048109875011, 41.64886208192144323 ) ) ;
#3698=CARTESIAN_POINT ( 'NONE',  ( -12.01549611932652972, 203.1486557965464499, 81.35113791807857808 ) ) ;
#3699=CARTESIAN_POINT ( 'NONE',  ( 2.517493886308900919, 214.5937144450984420, 97.40113791807858945 ) ) ;
#3701=CARTESIAN_POINT ( 'NONE',  ( -8.118202686958138514, 212.8392687619910930, 59.79886208192143471 ) ) ;
#3705=CARTESIAN_POINT ( 'NONE',  ( 7.456977232089471386, 196.8216656703012006, 64.44886208192143329 ) ) ;
#3708=CARTESIAN_POINT ( 'NONE',  ( -4.984841277089891776, 213.7757310962905990, 44.94886208192144039 ) ) ;
#3710=ORIENTED_EDGE ( 'NONE', *, *, #10798, .F. ) ;
#3714=CARTESIAN_POINT ( 'NONE',  ( 6.444103211791042618, 202.2591342207267644, 53.30113791807858092 ) ) ;
#3717=CARTESIAN_POINT ( 'NONE',  ( 6.220909254589681581, 198.5229672870052582, 28.44886208192143684 ) ) ;
#3721=( NAMED_UNIT ( * ) SI_UNIT ( $, .STERADIAN. ) SOLID_ANGLE_UNIT ( ) );
#3724=CARTESIAN_POINT ( 'NONE',  ( -8.015496119326597224, 209.5516654185217362, 17.64886208192143968 ) ) ;
#3725=CARTESIAN_POINT ( 'NONE',  ( 10.00000000000000711, 206.9523078486586201, 62.00113791807856956 ) ) ;
#3726=CARTESIAN_POINT ( 'NONE',  ( -6.220909254589537696, 198.5229672870051161, 33.05113791807857382 ) ) ;
#3729=CARTESIAN_POINT ( 'NONE',  ( 4.903702542908601636, 200.1653181626581102, -0.5488620819214340418 ) ) ;
#3733=CARTESIAN_POINT ( 'NONE',  ( 11.98450388067348271, 203.0532714938637753, 20.15113791807856458 ) ) ;
#3736=CARTESIAN_POINT ( 'NONE',  ( 6.220909254589536808, 215.4770327129947702, 67.55113791807853829 ) ) ;
#3738=CARTESIAN_POINT ( 'NONE',  ( -6.139770520408368348, 215.5359834540460042, 42.95113791807856529 ) ) ;
#3741=CARTESIAN_POINT ( 'NONE',  ( 3.662846001189864698, 218.4274158808046593, 3.398862081921433909 ) ) ;
#3742=CARTESIAN_POINT ( 'NONE',  ( 10.00000000000000711, 207.0476921513415220, 9.998862081921435774 ) ) ;
#3745=CARTESIAN_POINT ( 'NONE',  ( 7.456977232089302632, 217.1783343296989131, 49.55113791807856671 ) ) ;
#3747=CARTESIAN_POINT ( 'NONE',  ( -2.426778023690262742, 214.6231898156240163, 70.10113791807857808 ) ) ;
#3750=CARTESIAN_POINT ( 'NONE',  ( 10.01549611932659545, 203.7984951890123853, 28.14886208192143613 ) ) ;
#3754=CARTESIAN_POINT ( 'NONE',  ( 0.05014649552810505201, 217.5146222423826714, 79.25113791807856956 ) ) ;
#3761=CARTESIAN_POINT ( 'NONE',  ( 8.000000000000008882, 206.9523078486586485, 26.00113791807856600 ) ) ;
#3763=CARTESIAN_POINT ( 'NONE',  ( -6.220909254589682469, 215.4770327129946850, 8.948862081921435063 ) ) ;
#3767=CARTESIAN_POINT ( 'NONE',  ( 8.015496119326531499, 209.5516654185219636, 52.85113791807857098 ) ) ;
#3772=CARTESIAN_POINT ( 'NONE',  ( -3.135527875058982783, 216.4958274776886924, 90.09886208192143897 ) ) ;
#3774=CARTESIAN_POINT ( 'NONE',  ( 9.984503880673470277, 203.7031108863295401, 20.15113791807856813 ) ) ;
#3776=CARTESIAN_POINT ( 'NONE',  ( 7.375838497908012492, 217.2372850707501186, 78.54886208192142760 ) ) ;
#3780=CARTESIAN_POINT ( 'NONE',  ( -10.01549611932653860, 203.7984951890123284, 93.35113791807857808 ) ) ;
#3783=CARTESIAN_POINT ( 'NONE',  ( -9.984503880673473830, 210.2968891136704315, 39.65113791807857524 ) ) ;
#3790=CARTESIAN_POINT ( 'NONE',  ( -7.375838497908182134, 217.2372850707499765, 18.95113791807856529 ) ) ;
#3791=CARTESIAN_POINT ( 'NONE',  ( -11.00000000000000355, 206.9999999999998863, 103.5000000000000142 ) ) ;
#3794=CARTESIAN_POINT ( 'NONE',  ( -3.662846001189865142, 195.5725841191952838, 46.89886208192143613 ) ) ;
#3796=AXIS2_PLACEMENT_3D ( 'NONE', #21965, #24857, #19908 ) ;
#3797=CARTESIAN_POINT ( 'NONE',  ( 0.05014649552810505201, 217.5146222423826714, 49.25113791807857666 ) ) ;
#3798=CARTESIAN_POINT ( 'NONE',  ( -2.426778023690076225, 199.3768101843759553, 13.89886208192143613 ) ) ;
#3801=CARTESIAN_POINT ( 'NONE',  ( -7.984503880673422316, 204.3529502787951628, 104.3488620819214532 ) ) ;
#3803=CARTESIAN_POINT ( 'NONE',  ( -7.984503880673488041, 209.6470497212046098, 36.65113791807856103 ) ) ;
#3807=CARTESIAN_POINT ( 'NONE',  ( -3.135527875058982783, 216.4958274776886924, 57.09886208192143187 ) ) ;
#3810=CARTESIAN_POINT ( 'NONE',  ( 8.015496119326531499, 209.5516654185219636, 97.85113791807857808 ) ) ;
#3812=CARTESIAN_POINT ( 'NONE',  ( 4.984841277089891776, 200.2242689037093726, 73.44886208192143329 ) ) ;
#3816=CARTESIAN_POINT ( 'NONE',  ( 8.118202686958039038, 212.8392687619912635, 22.70113791807856884 ) ) ;
#3818=DIRECTION ( 'NONE',  ( 0.000000000000000000, -0.04769215134144031559, 0.9988620819214357738 ) ) ;
#3820=CARTESIAN_POINT ( 'NONE',  ( -12.01549611932652972, 203.1486557965464499, 84.35113791807857808 ) ) ;
#3821=CARTESIAN_POINT ( 'NONE',  ( -3.135527875058821579, 197.5041725223112223, 92.90113791807857524 ) ) ;
#3824=CARTESIAN_POINT ( 'NONE',  ( -0.05014649552828442242, 219.6175466908591716, 102.2488620819214447 ) ) ;
#3825=CARTESIAN_POINT ( 'NONE',  ( 7.375838497908012492, 217.2372850707501186, 63.54886208192144181 ) ) ;
#3826=CARTESIAN_POINT ( 'NONE',  ( -10.01549611932659545, 210.2015048109875011, 80.64886208192145034 ) ) ;
#3827=CARTESIAN_POINT ( 'NONE',  ( -9.736236675708031640, 214.0148392665760753, 5.798862081921434708 ) ) ;
#3829=CARTESIAN_POINT ( 'NONE',  ( 8.118202686958039038, 212.8392687619912635, 22.70113791807856884 ) ) ;
#3830=CARTESIAN_POINT ( 'NONE',  ( 10.01549611932659545, 203.7984951890123853, 85.14886208192143613 ) ) ;
#3836=CARTESIAN_POINT ( 'NONE',  ( -7.984503880673422316, 204.3529502787951628, 74.34886208192142476 ) ) ;
#3843=CARTESIAN_POINT ( 'NONE',  ( 8.015496119326531499, 209.5516654185219636, 70.85113791807857808 ) ) ;
#3847=CARTESIAN_POINT ( 'NONE',  ( -2.517493886309087880, 214.5937144450984135, 48.09886208192143897 ) ) ;
#3848=CARTESIAN_POINT ( 'NONE',  ( 10.00000000000000711, 206.9523078486586201, 92.00113791807858377 ) ) ;
#3849=CARTESIAN_POINT ( 'NONE',  ( -8.118202686958039038, 201.1607312380087080, 72.20113791807857240 ) ) ;
#3854=CARTESIAN_POINT ( 'NONE',  ( 7.456977232089302632, 217.1783343296989131, 46.55113791807856671 ) ) ;
#3856=CARTESIAN_POINT ( 'NONE',  ( -3.753561863808691168, 195.6020594897209435, -0.09886208192143448870 ) ) ;
#3857=CARTESIAN_POINT ( 'NONE',  ( -8.118202686958039038, 201.1607312380087080, 72.20113791807857240 ) ) ;
#3858=CARTESIAN_POINT ( 'NONE',  ( -3.662846001189865142, 195.5725841191952838, 28.89886208192143613 ) ) ;
#3859=CARTESIAN_POINT ( 'NONE',  ( 3.135527875058981895, 197.5041725223112792, 43.59886208192143897 ) ) ;
#3861=CARTESIAN_POINT ( 'NONE',  ( 0.05014649552807549926, 219.6175466908591716, 79.25113791807856956 ) ) ;
#3862=CARTESIAN_POINT ( 'NONE',  ( -4.984841277089726574, 200.2242689037092305, 102.0511379180785809 ) ) ;
#3863=CARTESIAN_POINT ( 'NONE',  ( 8.118202686958138514, 201.1607312380088501, 64.29886208192144181 ) ) ;
#3867=CARTESIAN_POINT ( 'NONE',  ( -9.736236675708031640, 214.0148392665760753, 62.79886208192144892 ) ) ;
#3871=CARTESIAN_POINT ( 'NONE',  ( 6.444103211790928043, 211.7408657792734061, 45.69886208192144750 ) ) ;
#3876=CARTESIAN_POINT ( 'NONE',  ( -9.000000000000001776, 206.9999999999998863, 103.5000000000000426 ) ) ;
#3877=CARTESIAN_POINT ( 'NONE',  ( 2.517493886308900919, 214.5937144450984420, 55.40113791807858235 ) ) ;
#3878=CARTESIAN_POINT ( 'NONE',  ( -6.139770520408224463, 198.4640165459539389, 29.04886208192143471 ) ) ;
#3884=CARTESIAN_POINT ( 'NONE',  ( -6.500168698208244500, 211.6636982574061676, 14.79886208192143471 ) ) ;
#3885=CARTESIAN_POINT ( 'NONE',  ( -3.044812012440131443, 216.5253028482142952, 61.10113791807857098 ) ) ;
#3886=CARTESIAN_POINT ( 'NONE',  ( 9.984503880673470277, 203.7031108863295401, 35.15113791807856813 ) ) ;
#3888=CARTESIAN_POINT ( 'NONE',  ( -4.903702542908436435, 200.1653181626580249, 98.04886208192144181 ) ) ;
#3892=CARTESIAN_POINT ( 'NONE',  ( 9.680171189290831535, 199.9079932115568852, 20.30113791807857027 ) ) ;
#3895=CARTESIAN_POINT ( 'NONE',  ( -10.00000000000000711, 207.0476921513413515, 63.50113791807856956 ) ) ;
#3896=CARTESIAN_POINT ( 'NONE',  ( -6.220909254589537696, 198.5229672870051445, 42.05113791807857382 ) ) ;
#3899=CARTESIAN_POINT ( 'NONE',  ( 3.753561863808876797, 195.6020594897209719, 4.598862081921434530 ) ) ;
#3900=CARTESIAN_POINT ( 'NONE',  ( 6.139770520408223575, 215.5359834540460611, 12.54886208192143648 ) ) ;
#3904=CARTESIAN_POINT ( 'NONE',  ( 7.456977232089302632, 217.1783343296989131, 46.55113791807856671 ) ) ;
#3905=CARTESIAN_POINT ( 'NONE',  ( -8.000000000000008882, 207.0476921513413515, 72.50113791807856956 ) ) ;
#3906=CARTESIAN_POINT ( 'NONE',  ( 0.05014649552828275708, 196.4853777576173002, 34.74886208192143044 ) ) ;
#3910=CARTESIAN_POINT ( 'NONE',  ( -3.044812012440131443, 216.5253028482142952, 88.10113791807857808 ) ) ;
#3916=CARTESIAN_POINT ( 'NONE',  ( -2.517493886308901807, 199.4062855549015012, 23.90113791807857169 ) ) ;
#3920=CARTESIAN_POINT ( 'NONE',  ( 3.753561863808876797, 195.6020594897209719, 103.5988620819214532 ) ) ;
#3923=CARTESIAN_POINT ( 'NONE',  ( 6.500168698208129925, 211.6636982574063381, 46.70113791807857240 ) ) ;
#3928=CARTESIAN_POINT ( 'NONE',  ( -6.139770520408224463, 198.4640165459539389, 95.04886208192144181 ) ) ;
#3931=CARTESIAN_POINT ( 'NONE',  ( -9.984503880673473830, 210.2968891136704315, 33.65113791807856813 ) ) ;
#3934=CARTESIAN_POINT ( 'NONE',  ( 9.736236675708031640, 199.9851607334238963, 82.29886208192144181 ) ) ;
#3938=CARTESIAN_POINT ( 'NONE',  ( -10.01549611932653860, 203.7984951890123284, 99.35113791807857808 ) ) ;
#3941=CARTESIAN_POINT ( 'NONE',  ( 9.984503880673470277, 203.7031108863295401, 38.15113791807856813 ) ) ;
#3948=CARTESIAN_POINT ( 'NONE',  ( 7.456977232089302632, 217.1783343296989131, 19.55113791807856671 ) ) ;
#3950=CARTESIAN_POINT ( 'NONE',  ( -9.826090958526812358, 208.0352956435529563, 102.7846294209004441 ) ) ;
#3953=CARTESIAN_POINT ( 'NONE',  ( -9.736236675708031640, 214.0148392665760753, 44.79886208192143471 ) ) ;
#3954=CARTESIAN_POINT ( 'NONE',  ( 6.139770520408368348, 198.4640165459539674, 5.451137918078567068 ) ) ;
#3955=CARTESIAN_POINT ( 'NONE',  ( 9.984503880673470277, 203.7031108863295401, 56.15113791807856103 ) ) ;
#3957=CARTESIAN_POINT ( 'NONE',  ( 4.984841277089891776, 200.2242689037093726, 10.44886208192143506 ) ) ;
#3962=CARTESIAN_POINT ( 'NONE',  ( 7.984503880673422316, 209.6470497212048372, 102.8488620819214390 ) ) ;
#3966=CARTESIAN_POINT ( 'NONE',  ( 4.984841277089725686, 213.7757310962907411, 37.55113791807855961 ) ) ;
#3971=CARTESIAN_POINT ( 'NONE',  ( -8.118202686958138514, 212.8392687619910930, 65.79886208192144181 ) ) ;
#3975=CARTESIAN_POINT ( 'NONE',  ( 8.118202686958039038, 212.8392687619912635, 1.701137918078565736 ) ) ;
#3981=CARTESIAN_POINT ( 'NONE',  ( -4.984841277089891776, 213.7757310962905990, 83.94886208192144750 ) ) ;
#3987=CARTESIAN_POINT ( 'NONE',  ( 8.062137200540920645, 201.0835637161417822, 20.30113791807856671 ) ) ;
#3991=CARTESIAN_POINT ( 'NONE',  ( 12.01549611932652972, 210.8513442034534933, 85.85113791807857808 ) ) ;
#3995=CARTESIAN_POINT ( 'NONE',  ( 3.753561863808876797, 195.6020594897209719, 70.59886208192142476 ) ) ;
#3997=CARTESIAN_POINT ( 'NONE',  ( -6.220909254589682469, 215.4770327129947134, 77.94886208192141908 ) ) ;
#3998=CARTESIAN_POINT ( 'NONE',  ( 0.05014649552828288198, 194.3824533091408000, 10.74886208192143577 ) ) ;
#4001=CARTESIAN_POINT ( 'NONE',  ( -3.135527875058821579, 197.5041725223112223, 23.90113791807856813 ) ) ;
#4002=CARTESIAN_POINT ( 'NONE',  ( 6.139770520408223575, 215.5359834540460611, 93.54886208192139918 ) ) ;
#4007=CARTESIAN_POINT ( 'NONE',  ( -4.984841277089891776, 213.7757310962905990, 71.94886208192144750 ) ) ;
#4016=CARTESIAN_POINT ( 'NONE',  ( 0.05014649552807626948, 215.4116977939061144, 70.25113791807856956 ) ) ;
#4021=CARTESIAN_POINT ( 'NONE',  ( 0.05014649552828262524, 198.5883022060938572, 52.74886208192144466 ) ) ;
#4027=CARTESIAN_POINT ( 'NONE',  ( 3.753561863808689836, 218.3979405102790565, 58.40113791807858235 ) ) ;
#4030=CIRCLE ( 'NONE', #24140, 1.000000000000000222 ) ;
#4031=CARTESIAN_POINT ( 'NONE',  ( -6.220909254589537696, 198.5229672870051161, 102.0511379180785383 ) ) ;
#4032=CARTESIAN_POINT ( 'NONE',  ( -10.00000000000000711, 207.0476921513413515, 78.50113791807856956 ) ) ;
#4033=CARTESIAN_POINT ( 'NONE',  ( -9.680171189290716072, 199.9079932115567146, 38.19886208192142618 ) ) ;
#4034=CARTESIAN_POINT ( 'NONE',  ( 0.05014649552828275014, 196.4853777576173002, 49.74886208192142334 ) ) ;
#4036=CARTESIAN_POINT ( 'NONE',  ( -9.736236675707914401, 199.9851607334237542, 90.20113791807857240 ) ) ;
#4037=CARTESIAN_POINT ( 'NONE',  ( 8.000000000000008882, 206.9523078486586485, 95.00113791807856956 ) ) ;
#4038=CARTESIAN_POINT ( 'NONE',  ( -9.984503880673420539, 203.7031108863293980, 62.34886208192143897 ) ) ;
#4041=CARTESIAN_POINT ( 'NONE',  ( 3.753561863808876797, 195.6020594897209719, 64.59886208192142476 ) ) ;
#4044=CARTESIAN_POINT ( 'NONE',  ( -8.000000000000008882, 206.9523078486584780, 38.49886208192143044 ) ) ;
#4050=CARTESIAN_POINT ( 'NONE',  ( -6.444103211791042618, 211.7408657792732356, 57.80113791807857382 ) ) ;
#4051=CARTESIAN_POINT ( 'NONE',  ( -3.044812012439970683, 197.4746971517856196, 46.89886208192143613 ) ) ;
#4056=CARTESIAN_POINT ( 'NONE',  ( 2.517493886309087436, 199.4062855549015865, 25.59886208192143897 ) ) ;
#4057=CARTESIAN_POINT ( 'NONE',  ( -0.05014649552810635652, 196.4853777576173002, 56.75113791807855534 ) ) ;
#4059=CARTESIAN_POINT ( 'NONE',  ( 8.062137200540920645, 201.0835637161417822, 44.30113791807857382 ) ) ;
#4062=CARTESIAN_POINT ( 'NONE',  ( -9.984503880673473830, 210.2968891136704315, 15.65113791807856813 ) ) ;
#4063=CARTESIAN_POINT ( 'NONE',  ( -8.000000000000008882, 206.9523078486584780, 101.4988620819214304 ) ) ;
#4067=CARTESIAN_POINT ( 'NONE',  ( -12.01549611932652972, 203.1486557965464499, 30.35113791807856742 ) ) ;
#4069=CARTESIAN_POINT ( 'NONE',  ( -6.220909254589537696, 198.5229672870051161, 78.05113791807858092 ) ) ;
#4070=CARTESIAN_POINT ( 'NONE',  ( 9.984503880673473830, 203.7031108863295401, 38.15113791807857524 ) ) ;
#4073=CARTESIAN_POINT ( 'NONE',  ( 3.662846001190051659, 195.5725841191953691, 101.6011379180785781 ) ) ;
#4074=CARTESIAN_POINT ( 'NONE',  ( -3.044812012439970683, 197.4746971517856196, 16.89886208192143613 ) ) ;
#4077=CARTESIAN_POINT ( 'NONE',  ( 11.98450388067348271, 203.0532714938637753, 56.15113791807857524 ) ) ;
#4078=CARTESIAN_POINT ( 'NONE',  ( -6.500168698208129925, 202.3363017425936050, 69.20113791807857240 ) ) ;
#4079=CARTESIAN_POINT ( 'NONE',  ( -9.984503880673420539, 203.7031108863293980, 29.34886208192144252 ) ) ;
#4082=CARTESIAN_POINT ( 'NONE',  ( 9.984503880673470277, 203.7031108863295401, 86.15113791807857524 ) ) ;
#4083=ORIENTED_EDGE ( 'NONE', *, *, #9130, .T. ) ;
#4087=CARTESIAN_POINT ( 'NONE',  ( -6.444103211791042618, 211.7408657792732356, 36.80113791807856671 ) ) ;
#4089=CARTESIAN_POINT ( 'NONE',  ( 8.062137200540822946, 212.9164362838583315, 15.69886208192143506 ) ) ;
#4092=CARTESIAN_POINT ( 'NONE',  ( 6.500168698208129925, 211.6636982574063381, 49.70113791807857240 ) ) ;
#4095=CARTESIAN_POINT ( 'NONE',  ( -0.05014649552828403384, 217.5146222423826714, 93.24886208192140202 ) ) ;
#4097=CARTESIAN_POINT ( 'NONE',  ( -10.01549611932653860, 203.7984951890123284, 33.35113791807855677 ) ) ;
#4100=CARTESIAN_POINT ( 'NONE',  ( 6.220909254589536808, 215.4770327129947702, 22.55113791807856671 ) ) ;
#4104=CARTESIAN_POINT ( 'NONE',  ( 10.00000000000000711, 206.9523078486586201, 92.00113791807858377 ) ) ;
#4107=CARTESIAN_POINT ( 'NONE',  ( 10.01549611932653860, 210.2015048109876716, 46.85113791807856387 ) ) ;
#4114=CARTESIAN_POINT ( 'NONE',  ( -12.00000000000000711, 207.0476921513413515, 15.50113791807856600 ) ) ;
#4118=CARTESIAN_POINT ( 'NONE',  ( -0.05014649552828442242, 219.6175466908591716, 42.24886208192143044 ) ) ;
#4120=CARTESIAN_POINT ( 'NONE',  ( -3.135527875058821579, 197.5041725223112223, 59.90113791807856813 ) ) ;
#4123=CARTESIAN_POINT ( 'NONE',  ( -2.426778023690076225, 199.3768101843759553, 25.89886208192143613 ) ) ;
#4126=CARTESIAN_POINT ( 'NONE',  ( 6.500168698208244500, 202.3363017425938324, 103.2988620819214560 ) ) ;
#4130=CARTESIAN_POINT ( 'NONE',  ( 6.500168698208129925, 211.6636982574063381, 40.70113791807857240 ) ) ;
#4135=CARTESIAN_POINT ( 'NONE',  ( -8.118202686958039038, 201.1607312380087080, 0.2011379180785657361 ) ) ;
#4136=CARTESIAN_POINT ( 'NONE',  ( 6.220909254589681581, 198.5229672870052582, 61.44886208192141908 ) ) ;
#4138=CARTESIAN_POINT ( 'NONE',  ( 10.00000000000000711, 207.0000000000000853, 0.000000000000000000 ) ) ;
#4139=CARTESIAN_POINT ( 'NONE',  ( -9.984503880673473830, 210.2968891136704315, 0.6511379180785656917 ) ) ;
#4143=CARTESIAN_POINT ( 'NONE',  ( -2.426778023690076225, 199.3768101843759553, 79.89886208192143613 ) ) ;
#4147=CARTESIAN_POINT ( 'NONE',  ( -6.139770520408368348, 215.5359834540460042, 24.95113791807856174 ) ) ;
#4151=CARTESIAN_POINT ( 'NONE',  ( -11.98450388067348804, 210.9467285061362247, 90.65113791807857524 ) ) ;
#4156=CARTESIAN_POINT ( 'NONE',  ( 12.00000000000000711, 207.0476921513415220, 72.99886208192144466 ) ) ;
#4157=CARTESIAN_POINT ( 'NONE',  ( -9.984503880673420539, 203.7031108863293980, 74.34886208192143897 ) ) ;
#4158=CARTESIAN_POINT ( 'NONE',  ( -9.736236675708031640, 214.0148392665760753, 14.79886208192143471 ) ) ;
#4160=CARTESIAN_POINT ( 'NONE',  ( -6.139770520408369237, 215.5359834540460042, 27.95113791807856174 ) ) ;
#4164=CARTESIAN_POINT ( 'NONE',  ( -3.044812012439970683, 197.4746971517856196, 88.89886208192143613 ) ) ;
#4166=DIRECTION ( 'NONE',  ( -0.5526942671207060176, -0.1536855300543007452, -0.8190908404712106128 ) ) ;
#4169=CARTESIAN_POINT ( 'NONE',  ( 4.984841277089891776, 200.2242689037093726, 70.44886208192144750 ) ) ;
#4177=CARTESIAN_POINT ( 'NONE',  ( 2.426778023690261410, 199.3768101843759837, 80.60113791807857808 ) ) ;
#4182=CARTESIAN_POINT ( 'NONE',  ( -2.517493886309087880, 214.5937144450984135, 51.09886208192143897 ) ) ;
#4189=CARTESIAN_POINT ( 'NONE',  ( 9.680171189290831535, 199.9079932115568852, 56.30113791807857382 ) ) ;
#4191=CARTESIAN_POINT ( 'NONE',  ( 3.753561863808689836, 218.3979405102790565, 1.401137918078565692 ) ) ;
#4193=CARTESIAN_POINT ( 'NONE',  ( -3.135527875058821579, 197.5041725223112223, 80.90113791807858945 ) ) ;
#4194=CARTESIAN_POINT ( 'NONE',  ( -7.375838497908014268, 196.7627149292498530, 41.04886208192144181 ) ) ;
#4195=CARTESIAN_POINT ( 'NONE',  ( 6.220909254589680693, 198.5229672870052582, 49.44886208192144750 ) ) ;
#4197=CARTESIAN_POINT ( 'NONE',  ( 0.05014649552807549926, 219.6175466908591716, 85.25113791807856956 ) ) ;
#4199=CARTESIAN_POINT ( 'NONE',  ( 3.044812012440130555, 197.4746971517856764, 5.601137918078566535 ) ) ;
#4200=CARTESIAN_POINT ( 'NONE',  ( 6.220909254589681581, 198.5229672870052582, 58.44886208192144039 ) ) ;
#4203=CARTESIAN_POINT ( 'NONE',  ( -3.753561863808878130, 218.3979405102790281, 72.09886208192142476 ) ) ;
#4208=CARTESIAN_POINT ( 'NONE',  ( 2.517493886309087436, 199.4062855549015865, 46.59886208192143897 ) ) ;
#4213=CARTESIAN_POINT ( 'NONE',  ( 8.015496119326531499, 209.5516654185219636, 61.85113791807857098 ) ) ;
#4214=CARTESIAN_POINT ( 'NONE',  ( -9.984503880673420539, 203.7031108863293980, 41.34886208192143897 ) ) ;
#4217=SURFACE_STYLE_USAGE ( .BOTH. , #32163 ) ;
#4220=CARTESIAN_POINT ( 'NONE',  ( 6.500168698208244500, 202.3363017425938324, 22.29886208192143826 ) ) ;
#4222=CARTESIAN_POINT ( 'NONE',  ( 8.062137200540920645, 201.0835637161417822, 65.30113791807858092 ) ) ;
#4223=CARTESIAN_POINT ( 'NONE',  ( 10.00000000000000711, 206.9523078486586201, 50.00113791807856956 ) ) ;
#4227=CARTESIAN_POINT ( 'NONE',  ( 10.00000000000000711, 206.9523078486586201, 20.00113791807856600 ) ) ;
#4228=CARTESIAN_POINT ( 'NONE',  ( 2.517493886308900919, 214.5937144450984420, 4.401137918078566358 ) ) ;
#4232=CARTESIAN_POINT ( 'NONE',  ( -11.98450388067348804, 210.9467285061362247, 27.65113791807857169 ) ) ;
#4234=CARTESIAN_POINT ( 'NONE',  ( 9.984503880673470277, 203.7031108863295401, 74.15113791807854682 ) ) ;
#4235=CARTESIAN_POINT ( 'NONE',  ( 3.135527875058820690, 216.4958274776887492, 49.40113791807857524 ) ) ;
#4239=CARTESIAN_POINT ( 'NONE',  ( -12.01549611932659722, 210.8513442034533227, 17.64886208192143968 ) ) ;
#4240=CARTESIAN_POINT ( 'NONE',  ( 6.139770520408223575, 215.5359834540460611, 15.54886208192143471 ) ) ;
#4243=CARTESIAN_POINT ( 'NONE',  ( 3.753561863808689836, 218.3979405102790565, 55.40113791807858235 ) ) ;
#4244=CARTESIAN_POINT ( 'NONE',  ( 6.444103211791042618, 202.2591342207267644, 65.30113791807858092 ) ) ;
#4245=CARTESIAN_POINT ( 'NONE',  ( -3.135527875058982783, 216.4958274776886924, 27.09886208192143542 ) ) ;
#4249=CARTESIAN_POINT ( 'NONE',  ( 6.220909254589536808, 215.4770327129947702, 88.55113791807853829 ) ) ;
#4254=B_SPLINE_CURVE_WITH_KNOTS ( 'NONE', 3,
 ( #17277, #14715, #15056, #15232, #20685, #7579, #22899, #33631, #25620, #18128, #15400, #25956 ),
 .UNSPECIFIED., .F., .F.,
 ( 4, 2, 2, 2, 2, 4 ),
 ( 0.001914709330258871581, 0.002152771118959677116, 0.002390832907660482651, 0.002866956485062089818, 0.003343080062463696552, 0.003819203639865303718 ),
 .UNSPECIFIED. ) ;
#4258=CARTESIAN_POINT ( 'NONE',  ( -2.426778023690262742, 214.6231898156240163, 37.10113791807857098 ) ) ;
#4259=CARTESIAN_POINT ( 'NONE',  ( -0.3755270751584372513, 206.7692714347155629, 108.3323677711371573 ) ) ;
#4260=CARTESIAN_POINT ( 'NONE',  ( 3.044812012439969795, 216.5253028482143520, 12.39886208192143435 ) ) ;
#4264=CARTESIAN_POINT ( 'NONE',  ( -8.000000000000008882, 207.0476921513413515, 45.50113791807857666 ) ) ;
#4266=DIRECTION ( 'NONE',  ( 1.000000000000000000, 0.000000000000000000, 0.000000000000000000 ) ) ;
#4268=CARTESIAN_POINT ( 'NONE',  ( -3.044812012439970683, 197.4746971517856196, 103.8988620819214361 ) ) ;
#4270=CARTESIAN_POINT ( 'NONE',  ( -3.135527875058821579, 197.5041725223112223, 35.90113791807856813 ) ) ;
#4272=CARTESIAN_POINT ( 'NONE',  ( -8.118202686958039038, 201.1607312380087080, 15.20113791807856884 ) ) ;
#4276=DIRECTION ( 'NONE',  ( 0.000000000000000000, 0.9963496021943381020, -0.08536668089591059605 ) ) ;
#4278=CARTESIAN_POINT ( 'NONE',  ( 3.753561863808689836, 218.3979405102790565, 1.401137918078565692 ) ) ;
#4282=CARTESIAN_POINT ( 'NONE',  ( 8.062137200540920645, 201.0835637161417822, 47.30113791807857382 ) ) ;
#4290=CARTESIAN_POINT ( 'NONE',  ( -11.98450388067348804, 210.9467285061362247, 27.65113791807857169 ) ) ;
#4295=CARTESIAN_POINT ( 'NONE',  ( -0.05014649552828442242, 219.6175466908591716, 45.24886208192143755 ) ) ;
#4296=CARTESIAN_POINT ( 'NONE',  ( 6.220909254589536808, 215.4770327129947702, 4.551137918078564937 ) ) ;
#4297=CARTESIAN_POINT ( 'NONE',  ( -8.062137200540920645, 212.9164362838581894, 63.80113791807858092 ) ) ;
#4298=CARTESIAN_POINT ( 'NONE',  ( 4.903702542908435547, 213.8346818373419751, 27.54886208192144181 ) ) ;
#4302=CARTESIAN_POINT ( 'NONE',  ( 8.015496119326531499, 209.5516654185219636, 4.851137918078565647 ) ) ;
#4306=CARTESIAN_POINT ( 'NONE',  ( 7.456977232089471386, 196.8216656703012006, 88.44886208192144750 ) ) ;
#4312=CARTESIAN_POINT ( 'NONE',  ( -9.657736897290682521, 207.8482824000647611, 102.5857182426188388 ) ) ;
#4313=CARTESIAN_POINT ( 'NONE',  ( -10.01549611932659722, 210.2015048109875011, 74.64886208192142192 ) ) ;
#4316=CARTESIAN_POINT ( 'NONE',  ( 9.984503880673470277, 203.7031108863295401, 5.151137918078567246 ) ) ;
#4320=CARTESIAN_POINT ( 'NONE',  ( -8.015496119326597224, 209.5516654185217362, 86.64886208192143613 ) ) ;
#4324=CARTESIAN_POINT ( 'NONE',  ( 3.662846001189864698, 218.4274158808046593, 90.39886208192143613 ) ) ;
#4326=CARTESIAN_POINT ( 'NONE',  ( 0.05014649552810506589, 217.5146222423826714, 22.25113791807856956 ) ) ;
#4328=CARTESIAN_POINT ( 'NONE',  ( -0.3755270751584372513, 206.7692714347155629, 108.3323677711371573 ) ) ;
#4330=CARTESIAN_POINT ( 'NONE',  ( 9.680171189290831535, 199.9079932115568852, 89.30113791807858092 ) ) ;
#4335=CARTESIAN_POINT ( 'NONE',  ( -12.00000000000000711, 206.9523078486584780, 68.49886208192144466 ) ) ;
#4336=CARTESIAN_POINT ( 'NONE',  ( 3.135527875058981895, 197.5041725223112792, 73.59886208192143897 ) ) ;
#4337=CARTESIAN_POINT ( 'NONE',  ( 3.662846001189864698, 218.4274158808046593, 9.398862081921436129 ) ) ;
#4339=CARTESIAN_POINT ( 'NONE',  ( 8.062137200540920645, 201.0835637161417822, 35.30113791807857382 ) ) ;
#4341=CARTESIAN_POINT ( 'NONE',  ( 8.062137200540822946, 212.9164362838583315, 93.69886208192143329 ) ) ;
#4346=CARTESIAN_POINT ( 'NONE',  ( -0.05014649552828365914, 215.4116977939061144, 78.24886208192144466 ) ) ;
#4353=CARTESIAN_POINT ( 'NONE',  ( 6.500168698208129925, 211.6636982574063381, 76.70113791807857240 ) ) ;
#4357=CARTESIAN_POINT ( 'NONE',  ( 2.517493886309087436, 199.4062855549015865, 55.59886208192143897 ) ) ;
#4365=CARTESIAN_POINT ( 'NONE',  ( 9.736236675707914401, 214.0148392665762458, 61.70113791807857240 ) ) ;
#4368=CARTESIAN_POINT ( 'NONE',  ( -8.118202686958039038, 201.1607312380087080, 102.2011379180785866 ) ) ;
#4369=CARTESIAN_POINT ( 'NONE',  ( 6.139770520408367460, 198.4640165459539389, 77.45113791807855819 ) ) ;
#4370=CARTESIAN_POINT ( 'NONE',  ( 3.662846001189864698, 218.4274158808046593, 45.39886208192143613 ) ) ;
#4371=CARTESIAN_POINT ( 'NONE',  ( -6.220909254589682469, 215.4770327129947134, 44.94886208192143329 ) ) ;
#4373=CARTESIAN_POINT ( 'NONE',  ( 3.662846001190051659, 195.5725841191953691, 89.60113791807857808 ) ) ;
#4375=CARTESIAN_POINT ( 'NONE',  ( 8.062137200540920645, 201.0835637161417822, 2.301137918078566269 ) ) ;
#4376=CARTESIAN_POINT ( 'NONE',  ( -3.044812012439970683, 197.4746971517856196, 73.89886208192143613 ) ) ;
#4379=CARTESIAN_POINT ( 'NONE',  ( 3.662846001189864698, 218.4274158808046593, 72.39886208192143613 ) ) ;
#4382=CARTESIAN_POINT ( 'NONE',  ( -4.984841277089891776, 213.7757310962905990, 41.94886208192144750 ) ) ;
#4390=CARTESIAN_POINT ( 'NONE',  ( 10.00000000000000711, 207.0476921513415220, 42.99886208192143044 ) ) ;
#4391=VERTEX_POINT ( 'NONE', #13996 ) ;
#4395=CARTESIAN_POINT ( 'NONE',  ( 6.444103211790928043, 211.7408657792734061, 24.69886208192143684 ) ) ;
#4397=CARTESIAN_POINT ( 'NONE',  ( -6.220909254589537696, 198.5229672870051161, 60.05113791807855961 ) ) ;
#4399=CARTESIAN_POINT ( 'NONE',  ( -3.044812012440131443, 216.5253028482142952, 46.10113791807857098 ) ) ;
#4401=CARTESIAN_POINT ( 'NONE',  ( 6.220909254589536808, 215.4770327129947702, 19.55113791807856671 ) ) ;
#4402=CARTESIAN_POINT ( 'NONE',  ( 4.984841277089725686, 213.7757310962907411, 4.551137918078565825 ) ) ;
#4406=CARTESIAN_POINT ( 'NONE',  ( -0.05014649552807705357, 194.3824533091408000, 32.75113791807856956 ) ) ;
#4407=CARTESIAN_POINT ( 'NONE',  ( -0.3755270751584372513, 206.7692714347155629, 108.3323677711371573 ) ) ;
#4408=CARTESIAN_POINT ( 'NONE',  ( 8.062137200540920645, 201.0835637161417822, 74.30113791807858092 ) ) ;
#4409=CARTESIAN_POINT ( 'NONE',  ( -3.044812012440131443, 216.5253028482142952, 52.10113791807857808 ) ) ;
#4412=CARTESIAN_POINT ( 'NONE',  ( -7.456977232089471386, 217.1783343296987709, 11.94886208192143506 ) ) ;
#4413=CARTESIAN_POINT ( 'NONE',  ( 3.135527875058981895, 197.5041725223112792, 19.59886208192143542 ) ) ;
#4417=CARTESIAN_POINT ( 'NONE',  ( 7.375838497908181246, 196.7627149292499666, 62.45113791807857240 ) ) ;
#4418=CARTESIAN_POINT ( 'NONE',  ( 2.517493886308900919, 214.5937144450984420, 76.40113791807856103 ) ) ;
#4419=CARTESIAN_POINT ( 'NONE',  ( 0.05014649552828275708, 196.4853777576173002, 31.74886208192143044 ) ) ;
#4427=CARTESIAN_POINT ( 'NONE',  ( -8.000000000000008882, 207.0476921513413515, 30.50113791807856600 ) ) ;
#4429=CARTESIAN_POINT ( 'NONE',  ( 6.139770520408223575, 215.5359834540460611, 18.54886208192143826 ) ) ;
#4432=CARTESIAN_POINT ( 'NONE',  ( -6.444103211791042618, 211.7408657792732356, 45.80113791807857382 ) ) ;
#4436=CARTESIAN_POINT ( 'NONE',  ( 9.984503880673420539, 210.2968891136705167, 99.84886208192141055 ) ) ;
#4438=CARTESIAN_POINT ( 'NONE',  ( -6.139770520408369237, 215.5359834540460042, 30.95113791807857240 ) ) ;
#4440=CARTESIAN_POINT ( 'NONE',  ( 8.118202686958039038, 212.8392687619912635, 19.70113791807856884 ) ) ;
#4446=CARTESIAN_POINT ( 'NONE',  ( 12.00000000000000711, 206.9523078486586485, 2.001137918078565114 ) ) ;
#4449=CARTESIAN_POINT ( 'NONE',  ( 6.139770520408368348, 198.4640165459539674, 50.45113791807857240 ) ) ;
#4455=CARTESIAN_POINT ( 'NONE',  ( 3.662846001190051659, 195.5725841191953691, 29.60113791807856742 ) ) ;
#4458=CARTESIAN_POINT ( 'NONE',  ( -10.00000000000000711, 206.9523078486584495, 5.498862081921434886 ) ) ;
#4460=ORIENTED_EDGE ( 'NONE', *, *, #30545, .F. ) ;
#4462=CARTESIAN_POINT ( 'NONE',  ( -8.118202686958039038, 201.1607312380087080, 0.2011379180785657361 ) ) ;
#4463=CARTESIAN_POINT ( 'NONE',  ( -3.135527875058821579, 197.5041725223112223, 65.90113791807857524 ) ) ;
#4465=CARTESIAN_POINT ( 'NONE',  ( 8.000000000000008882, 207.0476921513415220, 27.99886208192144110 ) ) ;
#4469=CARTESIAN_POINT ( 'NONE',  ( -4.903702542908602524, 213.8346818373418898, 0.9511379180785658471 ) ) ;
#4471=CARTESIAN_POINT ( 'NONE',  ( 9.736236675708031640, 199.9851607334238963, 91.29886208192142760 ) ) ;
#4476=CARTESIAN_POINT ( 'NONE',  ( 3.044812012440130555, 197.4746971517856764, -0.3988620819214342972 ) ) ;
#4477=CARTESIAN_POINT ( 'NONE',  ( 10.01549611932659545, 203.7984951890123853, 67.14886208192143613 ) ) ;
#4480=CARTESIAN_POINT ( 'NONE',  ( 9.984503880673470277, 203.7031108863295401, 8.151137918078564581 ) ) ;
#4484=CARTESIAN_POINT ( 'NONE',  ( -6.139770520408369237, 215.5359834540460042, 90.95113791807854398 ) ) ;
#4486=CARTESIAN_POINT ( 'NONE',  ( 9.984503880673470277, 203.7031108863295401, 77.15113791807857524 ) ) ;
#4489=CARTESIAN_POINT ( 'NONE',  ( 9.736236675708031640, 199.9851607334238963, 85.29886208192145602 ) ) ;
#4492=CARTESIAN_POINT ( 'NONE',  ( 8.118202686958039038, 212.8392687619912635, 19.70113791807856884 ) ) ;
#4497=CARTESIAN_POINT ( 'NONE',  ( 9.736236675707914401, 214.0148392665762458, 82.70113791807858661 ) ) ;
#4501=CARTESIAN_POINT ( 'NONE',  ( -7.456977232089471386, 217.1783343296987709, 68.94886208192144750 ) ) ;
#4502=CARTESIAN_POINT ( 'NONE',  ( 10.01549611932659367, 203.7984951890124421, 76.14886208192143613 ) ) ;
#4503=CARTESIAN_POINT ( 'NONE',  ( 9.736236675708031640, 199.9851607334238963, 10.29886208192143471 ) ) ;
#4505=CARTESIAN_POINT ( 'NONE',  ( 3.135527875058820690, 216.4958274776887492, 31.40113791807857524 ) ) ;
#4507=CARTESIAN_POINT ( 'NONE',  ( -0.05014649552828403384, 217.5146222423826714, 102.2488620819214020 ) ) ;
#4512=CARTESIAN_POINT ( 'NONE',  ( -0.05014649552828365914, 215.4116977939061144, 84.24886208192143044 ) ) ;
#4518=EDGE_CURVE ( 'NONE', #11179, #24063, #32218, .T. ) ;
#4523=CARTESIAN_POINT ( 'NONE',  ( -2.426778023690262742, 214.6231898156240163, 79.10113791807857808 ) ) ;
#4527=CARTESIAN_POINT ( 'NONE',  ( 8.000000000000008882, 207.0476921513415220, 54.99886208192145176 ) ) ;
#4530=CARTESIAN_POINT ( 'NONE',  ( -0.3755270751584372513, 206.2625674640609645, 118.9447509161623344 ) ) ;
#4535=CARTESIAN_POINT ( 'NONE',  ( -7.375838497908182134, 217.2372850707499765, 57.95113791807855819 ) ) ;
#4536=DIRECTION ( 'NONE',  ( 0.5526942671207055735, 0.1536855300543024383, 0.8190908404712107238 ) ) ;
#4537=PRODUCT_DEFINITION_SHAPE ( 'NONE', 'NONE',  #1660 ) ;
#4538=CARTESIAN_POINT ( 'NONE',  ( -3.662846001190052991, 218.4274158808045740, 1.101137918078565647 ) ) ;
#4539=CARTESIAN_POINT ( 'NONE',  ( -6.220909254589537696, 198.5229672870051445, 81.05113791807858092 ) ) ;
#4541=CARTESIAN_POINT ( 'NONE',  ( -0.05014649552828442242, 219.6175466908591716, 42.24886208192143044 ) ) ;
#4542=CARTESIAN_POINT ( 'NONE',  ( 8.118202686958138514, 201.1607312380088501, 46.29886208192143471 ) ) ;
#4545=CARTESIAN_POINT ( 'NONE',  ( 0.05014649552807549926, 219.6175466908591716, 88.25113791807856956 ) ) ;
#4547=CARTESIAN_POINT ( 'NONE',  ( 8.118202686958039038, 212.8392687619912635, 4.701137918078565292 ) ) ;
#4549=CARTESIAN_POINT ( 'NONE',  ( -8.062137200540822946, 201.0835637161416400, 65.19886208192143329 ) ) ;
#4553=CARTESIAN_POINT ( 'NONE',  ( -7.375838497908014268, 196.7627149292498530, 68.04886208192144181 ) ) ;
#4556=CARTESIAN_POINT ( 'NONE',  ( -8.015496119326597224, 209.5516654185217362, 53.64886208192143613 ) ) ;
#4557=ORIENTED_EDGE ( 'NONE', *, *, #7388, .F. ) ;
#4565=CARTESIAN_POINT ( 'NONE',  ( -8.062137200540822946, 201.0835637161416400, 44.19886208192143329 ) ) ;
#4571=CARTESIAN_POINT ( 'NONE',  ( -4.903702542908436435, 200.1653181626580249, 29.04886208192143471 ) ) ;
#4573=CARTESIAN_POINT ( 'NONE',  ( -9.984503880673473830, 210.2968891136704315, 66.65113791807857524 ) ) ;
#4575=CARTESIAN_POINT ( 'NONE',  ( 6.139770520408368348, 198.4640165459539674, 50.45113791807857240 ) ) ;
#4576=CARTESIAN_POINT ( 'NONE',  ( -10.00000000000000711, 207.0476921513413515, 21.50113791807856956 ) ) ;
#4577=CARTESIAN_POINT ( 'NONE',  ( -2.517493886308901807, 199.4062855549015012, 2.901137918078565914 ) ) ;
#4580=CARTESIAN_POINT ( 'NONE',  ( 7.375838497908181246, 196.7627149292499666, 26.45113791807857240 ) ) ;
#4582=CARTESIAN_POINT ( 'NONE',  ( -3.135527875058821579, 197.5041725223112223, 74.90113791807857524 ) ) ;
#4583=CARTESIAN_POINT ( 'NONE',  ( -0.05014649552810635652, 196.4853777576173002, 50.75113791807856956 ) ) ;
#4588=CARTESIAN_POINT ( 'NONE',  ( 3.753561863808876797, 195.6020594897209719, 13.59886208192143719 ) ) ;
#4589=CARTESIAN_POINT ( 'NONE',  ( 8.118202686958138514, 201.1607312380088501, 22.29886208192143826 ) ) ;
#4592=CARTESIAN_POINT ( 'NONE',  ( 7.456977232089302632, 217.1783343296989131, 55.55113791807858092 ) ) ;
#4593=CARTESIAN_POINT ( 'NONE',  ( -6.500168698208129925, 202.3363017425936050, 81.20113791807858661 ) ) ;
#4595=CARTESIAN_POINT ( 'NONE',  ( 8.062137200540822946, 212.9164362838583315, 42.69886208192143329 ) ) ;
#4602=EDGE_CURVE ( 'NONE', #33380, #25118, #4982, .T. ) ;
#4606=CARTESIAN_POINT ( 'NONE',  ( 2.426778023690261410, 199.3768101843759837, 35.60113791807857098 ) ) ;
#4609=CARTESIAN_POINT ( 'NONE',  ( 3.135527875058981895, 197.5041725223112792, 10.59886208192143542 ) ) ;
#4612=CARTESIAN_POINT ( 'NONE',  ( 4.903702542908601636, 200.1653181626581102, 56.45113791807857950 ) ) ;
#4616=CARTESIAN_POINT ( 'NONE',  ( -9.984503880673420539, 203.7031108863293980, 104.3488620819214105 ) ) ;
#4618=CARTESIAN_POINT ( 'NONE',  ( -10.01549611932653860, 203.7984951890123284, 30.35113791807856742 ) ) ;
#4620=CARTESIAN_POINT ( 'NONE',  ( -3.044812012440131443, 216.5253028482142952, 19.10113791807856742 ) ) ;
#4624=CARTESIAN_POINT ( 'NONE',  ( -4.945910536743085117, 206.2642604888503968, -6.000000000000014211 ) ) ;
#4625=CARTESIAN_POINT ( 'NONE',  ( 6.220909254589536808, 215.4770327129947702, 100.5511379180785809 ) ) ;
#4628=CARTESIAN_POINT ( 'NONE',  ( -8.118202686958039038, 201.1607312380087080, 48.20113791807857950 ) ) ;
#4634=CARTESIAN_POINT ( 'NONE',  ( -3.753561863808691168, 195.6020594897209435, 32.90113791807856813 ) ) ;
#4636=CARTESIAN_POINT ( 'NONE',  ( -3.135527875058982783, 216.4958274776886924, 15.09886208192143542 ) ) ;
#4639=CARTESIAN_POINT ( 'NONE',  ( -6.139770520408369237, 215.5359834540460042, 3.951137918078566180 ) ) ;
#4640=CARTESIAN_POINT ( 'NONE',  ( 0.05014649552810505201, 217.5146222423826714, 58.25113791807856245 ) ) ;
#4642=CARTESIAN_POINT ( 'NONE',  ( 6.444103211790928043, 211.7408657792734061, 24.69886208192143684 ) ) ;
#4645=CARTESIAN_POINT ( 'NONE',  ( -4.984841277089726574, 200.2242689037092305, 6.051137918078566713 ) ) ;
#4647=CARTESIAN_POINT ( 'NONE',  ( -9.680171189290716072, 199.9079932115567146, 92.19886208192143329 ) ) ;
#4652=CARTESIAN_POINT ( 'NONE',  ( -6.220909254589537696, 198.5229672870051161, 0.05113791807856577637 ) ) ;
#4653=CARTESIAN_POINT ( 'NONE',  ( -8.118202686958138514, 212.8392687619910930, 74.79886208192144181 ) ) ;
#4656=CARTESIAN_POINT ( 'NONE',  ( -10.01549611932653860, 203.7984951890123284, 3.351137918078566091 ) ) ;
#4660=CARTESIAN_POINT ( 'NONE',  ( 9.984503880673470277, 203.7031108863295401, 92.15113791807856103 ) ) ;
#4662=CARTESIAN_POINT ( 'NONE',  ( 3.044812012440130555, 197.4746971517856764, 71.60113791807857808 ) ) ;
#4665=CARTESIAN_POINT ( 'NONE',  ( -12.00000000000000711, 206.9523078486584780, 86.49886208192144466 ) ) ;
#4667=CARTESIAN_POINT ( 'NONE',  ( 3.044812012440130555, 197.4746971517856764, 29.60113791807856742 ) ) ;
#4671=CARTESIAN_POINT ( 'NONE',  ( 7.375838497908181246, 196.7627149292499666, 95.45113791807858661 ) ) ;
#4674=CARTESIAN_POINT ( 'NONE',  ( -6.220909254589682469, 215.4770327129947134, 89.94886208192143329 ) ) ;
#4675=CARTESIAN_POINT ( 'NONE',  ( -9.680171189290716072, 199.9079932115567146, 20.19886208192143684 ) ) ;
#4677=CARTESIAN_POINT ( 'NONE',  ( 0.05014649552810505201, 217.5146222423826714, 37.25113791807855534 ) ) ;
#4679=CARTESIAN_POINT ( 'NONE',  ( -3.044812012439970683, 197.4746971517856196, 94.89886208192143613 ) ) ;
#4683=CARTESIAN_POINT ( 'NONE',  ( 2.517493886309087436, 199.4062855549015865, 79.59886208192143897 ) ) ;
#4691=CARTESIAN_POINT ( 'NONE',  ( 7.984503880673485376, 204.3529502787953902, 83.15113791807856103 ) ) ;
#4693=CARTESIAN_POINT ( 'NONE',  ( 2.517493886309087436, 199.4062855549015865, 58.59886208192145318 ) ) ;
#4695=CARTESIAN_POINT ( 'NONE',  ( 8.062137200540920645, 201.0835637161417822, 2.301137918078566269 ) ) ;
#4700=CARTESIAN_POINT ( 'NONE',  ( 7.375838497908181246, 196.7627149292499666, 62.45113791807857240 ) ) ;
#4702=CARTESIAN_POINT ( 'NONE',  ( 7.456977232089302632, 217.1783343296989131, 10.55113791807856671 ) ) ;
#4703=CARTESIAN_POINT ( 'NONE',  ( 0.05014649552810506589, 217.5146222423826714, 76.25113791807856956 ) ) ;
#4705=CARTESIAN_POINT ( 'NONE',  ( -9.736236675708031640, 214.0148392665760753, 44.79886208192143471 ) ) ;
#4706=CARTESIAN_POINT ( 'NONE',  ( -10.00000000000000711, 206.9523078486584495, 59.49886208192143755 ) ) ;
#4708=CARTESIAN_POINT ( 'NONE',  ( 9.736236675707914401, 214.0148392665762458, 88.70113791807857240 ) ) ;
#4710=CARTESIAN_POINT ( 'NONE',  ( 6.139770520408368348, 198.4640165459539674, 8.451137918078565292 ) ) ;
#4711=CARTESIAN_POINT ( 'NONE',  ( 8.062137200540822946, 212.9164362838583315, 66.69886208192143329 ) ) ;
#4714=CARTESIAN_POINT ( 'NONE',  ( -3.662846001189865142, 195.5725841191952838, 73.89886208192143613 ) ) ;
#4717=CARTESIAN_POINT ( 'NONE',  ( -2.426778023690076225, 199.3768101843759553, 55.89886208192144323 ) ) ;
#4724=DIRECTION ( 'NONE',  ( 0.000000000000000000, 0.04769215134145521340, 0.9988620819214352187 ) ) ;
#4727=CARTESIAN_POINT ( 'NONE',  ( -3.135527875058982783, 216.4958274776886924, 39.09886208192143187 ) ) ;
#4734=CARTESIAN_POINT ( 'NONE',  ( -6.444103211790928043, 202.2591342207265939, 23.19886208192143684 ) ) ;
#4735=CARTESIAN_POINT ( 'NONE',  ( -0.05014649552810635652, 196.4853777576173002, 68.75113791807855534 ) ) ;
#4736=CARTESIAN_POINT ( 'NONE',  ( -10.01549611932653860, 203.7984951890123284, 48.35113791807855677 ) ) ;
#4738=CARTESIAN_POINT ( 'NONE',  ( -3.135527875058821579, 197.5041725223112223, 20.90113791807856813 ) ) ;
#4739=CARTESIAN_POINT ( 'NONE',  ( -7.984503880673488041, 209.6470497212046098, 9.651137918078566358 ) ) ;
#4741=CARTESIAN_POINT ( 'NONE',  ( 3.753561863808689836, 218.3979405102790565, 25.40113791807857169 ) ) ;
#4745=CARTESIAN_POINT ( 'NONE',  ( 6.139770520408368348, 198.4640165459539674, 71.45113791807857240 ) ) ;
#4746=CARTESIAN_POINT ( 'NONE',  ( -3.135527875058821579, 197.5041725223112223, 44.90113791807857524 ) ) ;
#4750=CARTESIAN_POINT ( 'NONE',  ( -9.736236675708031640, 214.0148392665760753, 14.79886208192143471 ) ) ;
#4751=CARTESIAN_POINT ( 'NONE',  ( 8.062137200540822946, 212.9164362838583315, 18.69886208192143329 ) ) ;
#4754=CARTESIAN_POINT ( 'NONE',  ( -7.456977232089304408, 196.8216656703010301, 57.05113791807856671 ) ) ;
#4755=CARTESIAN_POINT ( 'NONE',  ( -7.984503880673488041, 209.6470497212046098, 78.65113791807858945 ) ) ;
#4757=CARTESIAN_POINT ( 'NONE',  ( 3.044812012439969795, 216.5253028482143520, 36.39886208192142902 ) ) ;
#4758=CARTESIAN_POINT ( 'NONE',  ( -9.996365641501871124, 207.8097375604742467, 102.5363179372327096 ) ) ;
#4766=CARTESIAN_POINT ( 'NONE',  ( -8.000000000000008882, 207.0476921513413515, 33.50113791807857666 ) ) ;
#4768=CARTESIAN_POINT ( 'NONE',  ( 0.05014649552828275708, 196.4853777576173002, 10.74886208192143755 ) ) ;
#4771=CARTESIAN_POINT ( 'NONE',  ( -2.426778023690262742, 214.6231898156240163, 58.10113791807857808 ) ) ;
#4774=CARTESIAN_POINT ( 'NONE',  ( 10.01549611932659545, 203.7984951890123853, 100.1488620819214077 ) ) ;
#4776=CARTESIAN_POINT ( 'NONE',  ( 3.135527875058820690, 216.4958274776887492, 40.40113791807857524 ) ) ;
#4778=EDGE_CURVE ( 'NONE', #25118, #33380, #24597, .T. ) ;
#4779=CARTESIAN_POINT ( 'NONE',  ( 6.220909254589536808, 215.4770327129947702, 13.55113791807856849 ) ) ;
#4780=CARTESIAN_POINT ( 'NONE',  ( 3.135527875058981895, 197.5041725223112792, 100.5988620819214390 ) ) ;
#4786=CARTESIAN_POINT ( 'NONE',  ( 7.456977232089302632, 217.1783343296989131, 1.551137918078565603 ) ) ;
#4790=CARTESIAN_POINT ( 'NONE',  ( 0.05014649552810505201, 217.5146222423826714, 43.25113791807856956 ) ) ;
#4796=CARTESIAN_POINT ( 'NONE',  ( -7.456977232089304408, 196.8216656703010301, 27.05113791807857027 ) ) ;
#4800=CARTESIAN_POINT ( 'NONE',  ( 10.00000000000000711, 207.0476921513415220, 15.99886208192143400 ) ) ;
#4803=CARTESIAN_POINT ( 'NONE',  ( 9.984503880673470277, 203.7031108863295401, 8.151137918078564581 ) ) ;
#4804=CARTESIAN_POINT ( 'NONE',  ( -10.01549611932653860, 203.7984951890123284, 72.35113791807859229 ) ) ;
#4806=CARTESIAN_POINT ( 'NONE',  ( -6.444103211790928043, 202.2591342207265939, 23.19886208192143684 ) ) ;
#4810=CARTESIAN_POINT ( 'NONE',  ( 0.05014649552807626948, 215.4116977939061144, 7.251137918078565114 ) ) ;
#4811=CARTESIAN_POINT ( 'NONE',  ( 7.375838497908012492, 217.2372850707501186, 93.54886208192142760 ) ) ;
#4816=CARTESIAN_POINT ( 'NONE',  ( -10.00000000000000711, 207.0476921513413515, 3.501137918078566003 ) ) ;
#4818=CARTESIAN_POINT ( 'NONE',  ( 3.135527875058981895, 197.5041725223112792, 70.59886208192143897 ) ) ;
#4821=CARTESIAN_POINT ( 'NONE',  ( 10.01549611932653860, 210.2015048109876716, 16.85113791807856032 ) ) ;
#4827=CARTESIAN_POINT ( 'NONE',  ( -10.00000000000000711, 207.0476921513413515, 93.50113791807858377 ) ) ;
#4829=CARTESIAN_POINT ( 'NONE',  ( 0.05014649552810505201, 217.5146222423826714, 73.25113791807855534 ) ) ;
#4833=CARTESIAN_POINT ( 'NONE',  ( -9.680171189290716072, 199.9079932115567146, 83.19886208192144750 ) ) ;
#4836=CARTESIAN_POINT ( 'NONE',  ( -6.220909254589537696, 198.5229672870051445, 30.05113791807856671 ) ) ;
#4840=CARTESIAN_POINT ( 'NONE',  ( 3.753561863808689836, 218.3979405102790565, 94.40113791807857524 ) ) ;
#4843=CARTESIAN_POINT ( 'NONE',  ( -8.062137200540822946, 201.0835637161416400, 83.19886208192143329 ) ) ;
#4844=CARTESIAN_POINT ( 'NONE',  ( 12.00000000000000711, 207.0476921513415220, 18.99886208192143400 ) ) ;
#4846=CARTESIAN_POINT ( 'NONE',  ( -9.984503880673473830, 210.2968891136704315, 30.65113791807856813 ) ) ;
#4848=CARTESIAN_POINT ( 'NONE',  ( 8.118202686958138514, 201.1607312380088501, 94.29886208192144181 ) ) ;
#4853=CARTESIAN_POINT ( 'NONE',  ( 7.984503880673422316, 209.6470497212048372, 84.84886208192142476 ) ) ;
#4860=CARTESIAN_POINT ( 'NONE',  ( 8.015496119326531499, 209.5516654185219636, 58.85113791807857098 ) ) ;
#4863=CARTESIAN_POINT ( 'NONE',  ( 7.984503880673485376, 204.3529502787953902, 77.15113791807857524 ) ) ;
#4866=CARTESIAN_POINT ( 'NONE',  ( 8.000000000000008882, 207.0476921513415220, 60.99886208192144466 ) ) ;
#4869=CARTESIAN_POINT ( 'NONE',  ( 6.220909254589536808, 215.4770327129947987, 1.551137918078565825 ) ) ;
#4874=CARTESIAN_POINT ( 'NONE',  ( 11.98450388067348271, 203.0532714938637753, 65.15113791807856103 ) ) ;
#4876=CARTESIAN_POINT ( 'NONE',  ( -0.05014649552807705357, 194.3824533091408000, 11.75113791807856600 ) ) ;
#4878=CARTESIAN_POINT ( 'NONE',  ( 3.135527875058820690, 216.4958274776887492, 88.40113791807857524 ) ) ;
#4879=CARTESIAN_POINT ( 'NONE',  ( -12.00000000000000711, 206.9523078486584780, 47.49886208192144466 ) ) ;
#4880=CARTESIAN_POINT ( 'NONE',  ( -3.135527875058982783, 216.4958274776886924, 54.09886208192143897 ) ) ;
#4883=CARTESIAN_POINT ( 'NONE',  ( 12.01549611932652972, 210.8513442034534933, 97.85113791807857808 ) ) ;
#4885=CARTESIAN_POINT ( 'NONE',  ( 0.05014649552810505201, 217.5146222423826714, 1.251137918078566003 ) ) ;
#4886=CARTESIAN_POINT ( 'NONE',  ( -10.01549611932659722, 210.2015048109875011, 68.64886208192143613 ) ) ;
#4889=CARTESIAN_POINT ( 'NONE',  ( 9.736236675708031640, 199.9851607334238963, 70.29886208192142760 ) ) ;
#4890=CARTESIAN_POINT ( 'NONE',  ( 6.220909254589536808, 215.4770327129947702, 94.55113791807858092 ) ) ;
#4893=CARTESIAN_POINT ( 'NONE',  ( -4.984841277089891776, 213.7757310962905990, 53.94886208192144039 ) ) ;
#4894=CIRCLE ( 'NONE', #3796, 1.000000000000000888 ) ;
#4901=CARTESIAN_POINT ( 'NONE',  ( -10.01549611932659722, 210.2015048109875011, 56.64886208192142902 ) ) ;
#4906=CARTESIAN_POINT ( 'NONE',  ( -8.015496119326597224, 209.5516654185217362, 38.64886208192143613 ) ) ;
#4907=CARTESIAN_POINT ( 'NONE',  ( 3.135527875058820690, 216.4958274776887492, 73.40113791807857524 ) ) ;
#4909=CARTESIAN_POINT ( 'NONE',  ( -9.984503880673473830, 210.2968891136704315, 60.65113791807856103 ) ) ;
#4911=CARTESIAN_POINT ( 'NONE',  ( -6.139770520408369237, 215.5359834540460042, 30.95113791807857240 ) ) ;
#4912=CARTESIAN_POINT ( 'NONE',  ( 8.015496119326531499, 209.5516654185219636, 7.851137918078565647 ) ) ;
#4916=CARTESIAN_POINT ( 'NONE',  ( -7.456977232089304408, 196.8216656703010301, 42.05113791807857382 ) ) ;
#4918=CARTESIAN_POINT ( 'NONE',  ( -8.118202686958039038, 201.1607312380087080, 81.20113791807857240 ) ) ;
#4920=CARTESIAN_POINT ( 'NONE',  ( -3.135527875058821579, 197.5041725223112223, 56.90113791807857524 ) ) ;
#4922=CARTESIAN_POINT ( 'NONE',  ( 9.680171189290716072, 214.0920067884432854, 9.698862081921433287 ) ) ;
#4923=CARTESIAN_POINT ( 'NONE',  ( 8.118202686958138514, 201.1607312380088501, 31.29886208192143826 ) ) ;
#4926=CARTESIAN_POINT ( 'NONE',  ( 3.753561863808689836, 218.3979405102790565, 67.40113791807856103 ) ) ;
#4927=CARTESIAN_POINT ( 'NONE',  ( 4.984841277089725686, 213.7757310962907411, 76.55113791807858092 ) ) ;
#4928=CARTESIAN_POINT ( 'NONE',  ( 6.139770520408223575, 215.5359834540460611, 36.54886208192142050 ) ) ;
#4932=CARTESIAN_POINT ( 'NONE',  ( -7.375838497908014268, 196.7627149292498530, 41.04886208192144181 ) ) ;
#4940=CARTESIAN_POINT ( 'NONE',  ( 4.984841277089725686, 213.7757310962907411, 43.55113791807857382 ) ) ;
#4941=CARTESIAN_POINT ( 'NONE',  ( -10.01549611932659722, 210.2015048109875011, 26.64886208192142902 ) ) ;
#4944=CARTESIAN_POINT ( 'NONE',  ( -4.903702542908602524, 213.8346818373418898, 54.95113791807857240 ) ) ;
#4945=CARTESIAN_POINT ( 'NONE',  ( -10.00000000000000178, 206.7692714347156198, 108.3323677711372000 ) ) ;
#4947=CARTESIAN_POINT ( 'NONE',  ( 0.05014649552828275708, 196.4853777576173002, 100.7488620819214304 ) ) ;
#4950=CARTESIAN_POINT ( 'NONE',  ( -3.135527875058821579, 197.5041725223112223, 38.90113791807857524 ) ) ;
#4952=CARTESIAN_POINT ( 'NONE',  ( 8.062137200540920645, 201.0835637161417822, 23.30113791807856671 ) ) ;
#4953=CARTESIAN_POINT ( 'NONE',  ( 8.118202686958138514, 201.1607312380088501, 100.2988620819214418 ) ) ;
#4956=CARTESIAN_POINT ( 'NONE',  ( 4.903702542908435547, 213.8346818373419751, 78.54886208192142760 ) ) ;
#4960=CARTESIAN_POINT ( 'NONE',  ( 12.01549611932652972, 210.8513442034534933, 4.851137918078565647 ) ) ;
#4963=CARTESIAN_POINT ( 'NONE',  ( -10.00000000000000711, 207.0476921513413515, 60.50113791807857666 ) ) ;
#4970=CARTESIAN_POINT ( 'NONE',  ( 0.05014649552807549926, 219.6175466908591716, 28.25113791807856245 ) ) ;
#4972=CARTESIAN_POINT ( 'NONE',  ( -9.984503880673420539, 203.7031108863293980, 14.34886208192143542 ) ) ;
#4977=CARTESIAN_POINT ( 'NONE',  ( -10.01549611932653860, 203.7984951890123284, 12.35113791807856387 ) ) ;
#4978=CARTESIAN_POINT ( 'NONE',  ( -8.062137200540920645, 212.9164362838581894, 66.80113791807858092 ) ) ;
#4980=CARTESIAN_POINT ( 'NONE',  ( -2.517493886309087880, 214.5937144450984135, 30.09886208192144252 ) ) ;
#4982=CIRCLE ( 'NONE', #24008, 0.9999999999999915623 ) ;
#4984=CARTESIAN_POINT ( 'NONE',  ( -2.426778023690262742, 214.6231898156240163, 1.101137918078566091 ) ) ;
#4986=CARTESIAN_POINT ( 'NONE',  ( 9.680171189290716072, 214.0920067884432854, 84.69886208192144750 ) ) ;
#4991=CARTESIAN_POINT ( 'NONE',  ( 10.00000000000000711, 206.9523078486586201, 5.001137918078565114 ) ) ;
#4992=CARTESIAN_POINT ( 'NONE',  ( -8.118202686958138514, 212.8392687619910930, 71.79886208192142760 ) ) ;
#4995=CARTESIAN_POINT ( 'NONE',  ( -8.062137200540920645, 212.9164362838581894, 15.80113791807856849 ) ) ;
#4998=CARTESIAN_POINT ( 'NONE',  ( 10.01549611932653860, 210.2015048109876716, 100.8511379180785497 ) ) ;
#5000=CARTESIAN_POINT ( 'NONE',  ( 8.118202686958039038, 212.8392687619912635, 79.70113791807857240 ) ) ;
#5003=CARTESIAN_POINT ( 'NONE',  ( -9.736236675708031640, 214.0148392665760753, 86.79886208192142760 ) ) ;
#5008=CARTESIAN_POINT ( 'NONE',  ( -11.98450388067348804, 210.9467285061362247, 99.65113791807858945 ) ) ;
#5011=CARTESIAN_POINT ( 'NONE',  ( 0.05014649552828275014, 196.4853777576173002, 82.74886208192143044 ) ) ;
#5013=CARTESIAN_POINT ( 'NONE',  ( 12.01549611932659367, 203.1486557965466773, 22.14886208192143613 ) ) ;
#5015=CARTESIAN_POINT ( 'NONE',  ( 8.062137200540920645, 201.0835637161417822, 44.30113791807857382 ) ) ;
#5017=CARTESIAN_POINT ( 'NONE',  ( 0.05014649552828275708, 196.4853777576173002, 100.7488620819214304 ) ) ;
#5022=CARTESIAN_POINT ( 'NONE',  ( -7.984503880673422316, 204.3529502787951628, 80.34886208192143897 ) ) ;
#5027=ORIENTED_EDGE ( 'NONE', *, *, #10798, .T. ) ;
#5029=CARTESIAN_POINT ( 'NONE',  ( -0.05014649552807731031, 198.5883022060938572, 59.75113791807857666 ) ) ;
#5032=CARTESIAN_POINT ( 'NONE',  ( -6.500168698208129925, 202.3363017425936050, 84.20113791807858661 ) ) ;
#5036=CARTESIAN_POINT ( 'NONE',  ( 6.444103211790928043, 211.7408657792734061, 63.69886208192144039 ) ) ;
#5044=CARTESIAN_POINT ( 'NONE',  ( -11.98450388067348804, 210.9467285061362247, 63.65113791807855392 ) ) ;
#5046=CARTESIAN_POINT ( 'NONE',  ( 7.375838497908181246, 196.7627149292499666, 14.45113791807856707 ) ) ;
#5047=CARTESIAN_POINT ( 'NONE',  ( -3.135527875058821579, 197.5041725223112223, 86.90113791807857524 ) ) ;
#5048=CARTESIAN_POINT ( 'NONE',  ( 7.375838497908012492, 217.2372850707501186, 48.54886208192142050 ) ) ;
#5050=CARTESIAN_POINT ( 'NONE',  ( -8.062137200540822946, 201.0835637161416400, 56.19886208192144039 ) ) ;
#5052=CARTESIAN_POINT ( 'NONE',  ( -12.01549611932652972, 203.1486557965464499, 99.35113791807857808 ) ) ;
#5054=CARTESIAN_POINT ( 'NONE',  ( -6.139770520408369237, 215.5359834540460042, 15.95113791807856884 ) ) ;
#5055=CARTESIAN_POINT ( 'NONE',  ( -10.01549611932659722, 210.2015048109875011, 71.64886208192143613 ) ) ;
#5057=CARTESIAN_POINT ( 'NONE',  ( -11.98450388067341876, 203.0532714938636047, 77.34886208192143897 ) ) ;
#5058=CARTESIAN_POINT ( 'NONE',  ( -0.05014649552810635652, 196.4853777576173002, 89.75113791807854113 ) ) ;
#5062=CARTESIAN_POINT ( 'NONE',  ( 2.426778023690075337, 214.6231898156240447, 48.39886208192144323 ) ) ;
#5069=CARTESIAN_POINT ( 'NONE',  ( -10.00000000000000711, 206.9523078486584495, 47.49886208192143755 ) ) ;
#5073=CARTESIAN_POINT ( 'NONE',  ( -4.984841277089891776, 213.7757310962905990, 29.94886208192143684 ) ) ;
#5074=CARTESIAN_POINT ( 'NONE',  ( -0.05014649552810635652, 196.4853777576173002, 71.75113791807858377 ) ) ;
#5076=CARTESIAN_POINT ( 'NONE',  ( -6.220909254589537696, 198.5229672870051161, 60.05113791807855961 ) ) ;
#5077=CARTESIAN_POINT ( 'NONE',  ( 8.062137200540920645, 201.0835637161417822, 29.30113791807857027 ) ) ;
#5078=CARTESIAN_POINT ( 'NONE',  ( -8.015496119326531499, 204.4483345814780364, 15.35113791807856387 ) ) ;
#5083=CARTESIAN_POINT ( 'NONE',  ( -9.680171189290831535, 214.0920067884431148, 36.80113791807856671 ) ) ;
#5086=CARTESIAN_POINT ( 'NONE',  ( -6.220909254589537696, 198.5229672870051161, 84.05113791807855250 ) ) ;
#5087=CARTESIAN_POINT ( 'NONE',  ( -10.00000000000000711, 207.0476921513413515, 63.50113791807856956 ) ) ;
#5090=CARTESIAN_POINT ( 'NONE',  ( -3.753561863808878130, 218.3979405102790281, 21.09886208192143897 ) ) ;
#5091=CARTESIAN_POINT ( 'NONE',  ( -3.044812012439970683, 197.4746971517856196, 31.89886208192143613 ) ) ;
#5093=CARTESIAN_POINT ( 'NONE',  ( -12.01549611932652972, 203.1486557965464499, 66.35113791807857808 ) ) ;
#5094=CARTESIAN_POINT ( 'NONE',  ( -4.984841277089726574, 200.2242689037092305, 81.05113791807856671 ) ) ;
#5095=CARTESIAN_POINT ( 'NONE',  ( -3.044812012439970683, 197.4746971517856196, 40.89886208192143613 ) ) ;
#5098=CARTESIAN_POINT ( 'NONE',  ( -9.736236675708031640, 214.0148392665760753, 53.79886208192143471 ) ) ;
#5108=CARTESIAN_POINT ( 'NONE',  ( -0.05014649552807731031, 198.5883022060938572, 44.75113791807857666 ) ) ;
#5111=CARTESIAN_POINT ( 'NONE',  ( -6.139770520408224463, 198.4640165459539389, 23.04886208192143116 ) ) ;
#5116=CARTESIAN_POINT ( 'NONE',  ( 8.015496119326595448, 204.4483345814782638, 4.148862081921435241 ) ) ;
#5117=CARTESIAN_POINT ( 'NONE',  ( 6.220909254589536808, 215.4770327129947702, 40.55113791807855250 ) ) ;
#5119=CARTESIAN_POINT ( 'NONE',  ( -3.044812012440131443, 216.5253028482142952, 25.10113791807856742 ) ) ;
#5120=CARTESIAN_POINT ( 'NONE',  ( 8.062137200540822946, 212.9164362838583315, 102.6988620819214475 ) ) ;
#5123=CARTESIAN_POINT ( 'NONE',  ( 0.05014649552828262524, 198.5883022060938572, 94.74886208192144466 ) ) ;
#5127=CARTESIAN_POINT ( 'NONE',  ( -12.01549611932652972, 203.1486557965464499, 9.351137918078563871 ) ) ;
#5130=CARTESIAN_POINT ( 'NONE',  ( -6.220909254589537696, 198.5229672870051161, 57.05113791807857382 ) ) ;
#5133=CARTESIAN_POINT ( 'NONE',  ( 6.220909254589680693, 198.5229672870052582, 4.448862081921433287 ) ) ;
#5137=CARTESIAN_POINT ( 'NONE',  ( 3.753561863808689836, 218.3979405102790565, 40.40113791807857524 ) ) ;
#5139=CARTESIAN_POINT ( 'NONE',  ( 3.135527875058981895, 197.5041725223112792, 16.59886208192143542 ) ) ;
#5142=CARTESIAN_POINT ( 'NONE',  ( -6.139770520408369237, 215.5359834540460042, 12.95113791807856352 ) ) ;
#5143=CARTESIAN_POINT ( 'NONE',  ( 6.220909254589536808, 215.4770327129947702, 73.55113791807858092 ) ) ;
#5145=CARTESIAN_POINT ( 'NONE',  ( -8.000000000000008882, 206.9523078486584780, 32.49886208192143044 ) ) ;
#5146=( GEOMETRIC_REPRESENTATION_CONTEXT ( 3 ) GLOBAL_UNCERTAINTY_ASSIGNED_CONTEXT ( ( #505 ) ) GLOBAL_UNIT_ASSIGNED_CONTEXT ( ( #16997, #12058, #9172 ) ) REPRESENTATION_CONTEXT ( 'NONE', 'WORKASPACE' ) );
#5148=CARTESIAN_POINT ( 'NONE',  ( -8.000000000000008882, 207.0476921513413515, 12.50113791807856600 ) ) ;
#5150=CARTESIAN_POINT ( 'NONE',  ( -9.736236675708031640, 214.0148392665760753, 98.79886208192142760 ) ) ;
#5155=CARTESIAN_POINT ( 'NONE',  ( -8.118202686958039038, 201.1607312380087080, 9.201137918078565292 ) ) ;
#5156=CARTESIAN_POINT ( 'NONE',  ( -6.139770520408224463, 198.4640165459539389, 77.04886208192144181 ) ) ;
#5159=CARTESIAN_POINT ( 'NONE',  ( -10.00000000000000711, 207.0476921513413515, 15.50113791807856600 ) ) ;
#5163=CARTESIAN_POINT ( 'NONE',  ( 6.139770520408368348, 198.4640165459539674, 95.45113791807855819 ) ) ;
#5165=CARTESIAN_POINT ( 'NONE',  ( 10.01549611932653860, 210.2015048109876716, 82.85113791807854966 ) ) ;
#5168=CARTESIAN_POINT ( 'NONE',  ( 12.01549611932659367, 203.1486557965466773, 94.14886208192145034 ) ) ;
#5173=CARTESIAN_POINT ( 'NONE',  ( 12.01549611932652972, 210.8513442034534933, 100.8511379180785781 ) ) ;
#5177=ORIENTED_EDGE ( 'NONE', *, *, #9983, .F. ) ;
#5178=CARTESIAN_POINT ( 'NONE',  ( 6.139770520408223575, 215.5359834540460611, 90.54886208192144181 ) ) ;
#5179=CARTESIAN_POINT ( 'NONE',  ( 9.680171189290716072, 214.0920067884432854, 24.69886208192143684 ) ) ;
#5181=CARTESIAN_POINT ( 'NONE',  ( -10.01549611932653860, 203.7984951890123284, 45.35113791807857808 ) ) ;
#5184=CARTESIAN_POINT ( 'NONE',  ( 6.500168698208244500, 202.3363017425938324, 7.298862081921435596 ) ) ;
#5187=CARTESIAN_POINT ( 'NONE',  ( 4.903702542908435547, 213.8346818373419751, 87.54886208192142760 ) ) ;
#5189=CARTESIAN_POINT ( 'NONE',  ( 8.015496119326531499, 209.5516654185219636, 34.85113791807857098 ) ) ;
#5195=CARTESIAN_POINT ( 'NONE',  ( 2.517493886308900919, 214.5937144450984420, 88.40113791807857524 ) ) ;
#5199=CARTESIAN_POINT ( 'NONE',  ( -0.05014649552828365914, 215.4116977939061144, 63.24886208192142334 ) ) ;
#5208=CARTESIAN_POINT ( 'NONE',  ( 9.680171189290831535, 199.9079932115568852, 65.30113791807858092 ) ) ;
#5210=CARTESIAN_POINT ( 'NONE',  ( 7.375838497908181246, 196.7627149292499666, 5.451137918078566180 ) ) ;
#5212=CARTESIAN_POINT ( 'NONE',  ( 6.139770520408367460, 198.4640165459539389, 86.45113791807857240 ) ) ;
#5213=CARTESIAN_POINT ( 'NONE',  ( 0.05014649552828288198, 194.3824533091408000, 52.74886208192143755 ) ) ;
#5214=CARTESIAN_POINT ( 'NONE',  ( -3.135527875058982783, 216.4958274776886924, 57.09886208192143187 ) ) ;
#5215=CARTESIAN_POINT ( 'NONE',  ( 7.456977232089302632, 217.1783343296989131, 100.5511379180785809 ) ) ;
#5217=CARTESIAN_POINT ( 'NONE',  ( 3.044812012440130555, 197.4746971517856764, 14.60113791807856565 ) ) ;
#5219=CARTESIAN_POINT ( 'NONE',  ( -6.220909254589682469, 215.4770327129946850, 83.94886208192143329 ) ) ;
#5221=CARTESIAN_POINT ( 'NONE',  ( -7.375838497908014268, 196.7627149292498530, 80.04886208192144181 ) ) ;
#5222=CARTESIAN_POINT ( 'NONE',  ( 8.118202686958039038, 212.8392687619912635, 97.70113791807857240 ) ) ;
#5224=CARTESIAN_POINT ( 'NONE',  ( 3.273409709747122864, 207.3577873115561943, -8.276342481318904376 ) ) ;
#5225=CARTESIAN_POINT ( 'NONE',  ( 8.015496119326595448, 204.4483345814782638, 52.14886208192145034 ) ) ;
#5233=CARTESIAN_POINT ( 'NONE',  ( -8.118202686958138514, 212.8392687619910930, 53.79886208192143471 ) ) ;
#5236=ORIENTED_EDGE ( 'NONE', *, *, #20639, .F. ) ;
#5239=CARTESIAN_POINT ( 'NONE',  ( 2.426778023690075337, 214.6231898156240447, 33.39886208192144323 ) ) ;
#5240=CARTESIAN_POINT ( 'NONE',  ( -0.05014649552810635652, 196.4853777576173002, 74.75113791807858377 ) ) ;
#5242=CARTESIAN_POINT ( 'NONE',  ( 6.220909254589536808, 215.4770327129947702, 58.55113791807858092 ) ) ;
#5243=CARTESIAN_POINT ( 'NONE',  ( 9.984503880673470277, 203.7031108863295401, 32.15113791807857524 ) ) ;
#5244=CARTESIAN_POINT ( 'NONE',  ( -0.05014649552807731031, 198.5883022060938572, 11.75113791807856600 ) ) ;
#5248=CARTESIAN_POINT ( 'NONE',  ( 3.753561863808689836, 218.3979405102790565, 37.40113791807856813 ) ) ;
#5250=CARTESIAN_POINT ( 'NONE',  ( 6.139770520408368348, 198.4640165459539674, 89.45113791807857240 ) ) ;
#5251=CARTESIAN_POINT ( 'NONE',  ( 10.01549611932653860, 210.2015048109876716, 58.85113791807857098 ) ) ;
#5253=CARTESIAN_POINT ( 'NONE',  ( 7.375838497908012492, 217.2372850707501186, 27.54886208192144181 ) ) ;
#5254=CARTESIAN_POINT ( 'NONE',  ( 3.044812012439969795, 216.5253028482143520, 27.39886208192143613 ) ) ;
#5256=CARTESIAN_POINT ( 'NONE',  ( -7.375838497908182134, 217.2372850707499765, 66.95113791807857240 ) ) ;
#5257=CARTESIAN_POINT ( 'NONE',  ( 6.444103211791042618, 202.2591342207267644, 89.30113791807858092 ) ) ;
#5258=CARTESIAN_POINT ( 'NONE',  ( -0.05014649552828403384, 217.5146222423826714, 39.24886208192142334 ) ) ;
#5262=CARTESIAN_POINT ( 'NONE',  ( 12.00000000000000711, 207.0476921513415220, 48.99886208192143044 ) ) ;
#5269=CARTESIAN_POINT ( 'NONE',  ( -6.444103211791042618, 211.7408657792732356, 45.80113791807857382 ) ) ;
#5271=CARTESIAN_POINT ( 'NONE',  ( -9.984503880673420539, 203.7031108863293980, 20.34886208192143187 ) ) ;
#5276=CARTESIAN_POINT ( 'NONE',  ( 0.05014649552828262524, 198.5883022060938572, 7.748862081921434886 ) ) ;
#5278=CARTESIAN_POINT ( 'NONE',  ( 6.220909254589536808, 215.4770327129947702, 43.55113791807857382 ) ) ;
#5280=CARTESIAN_POINT ( 'NONE',  ( 9.984503880673470277, 203.7031108863295401, 26.15113791807856813 ) ) ;
#5285=CARTESIAN_POINT ( 'NONE',  ( 6.500168698208244500, 202.3363017425938324, 88.29886208192142760 ) ) ;
#5289=CARTESIAN_POINT ( 'NONE',  ( 11.98450388067348271, 203.0532714938637753, 14.15113791807856991 ) ) ;
#5292=CARTESIAN_POINT ( 'NONE',  ( 9.984503880673470277, 203.7031108863295401, 53.15113791807857524 ) ) ;
#5298=ORIENTED_EDGE ( 'NONE', *, *, #29583, .T. ) ;
#5299=CARTESIAN_POINT ( 'NONE',  ( -0.05014649552807705357, 194.3824533091408000, 35.75113791807857666 ) ) ;
#5302=CARTESIAN_POINT ( 'NONE',  ( 3.135527875058981895, 197.5041725223112792, 7.598862081921435419 ) ) ;
#5305=CARTESIAN_POINT ( 'NONE',  ( -10.01549611932653860, 203.7984951890123284, 69.35113791807857808 ) ) ;
#5307=ORIENTED_EDGE ( 'NONE', *, *, #29774, .T. ) ;
#5308=CARTESIAN_POINT ( 'NONE',  ( 6.444103211790928043, 211.7408657792734061, 36.69886208192144039 ) ) ;
#5314=CARTESIAN_POINT ( 'NONE',  ( 8.000000000000008882, 206.9523078486586485, 17.00113791807856956 ) ) ;
#5315=CARTESIAN_POINT ( 'NONE',  ( 11.98450388067341876, 210.9467285061363953, 99.84886208192143897 ) ) ;
#5320=CARTESIAN_POINT ( 'NONE',  ( 6.220909254589536808, 215.4770327129947702, 10.55113791807856138 ) ) ;
#5321=CARTESIAN_POINT ( 'NONE',  ( -8.118202686958138514, 212.8392687619910930, 83.79886208192144181 ) ) ;
#5324=CARTESIAN_POINT ( 'NONE',  ( -6.220909254589537696, 198.5229672870051161, 9.051137918078561384 ) ) ;
#5327=CARTESIAN_POINT ( 'NONE',  ( -9.984503880673473830, 210.2968891136704315, 96.65113791807857524 ) ) ;
#5329=CARTESIAN_POINT ( 'NONE',  ( 0.05014649552810505201, 217.5146222423826714, 82.25113791807858377 ) ) ;
#5333=CARTESIAN_POINT ( 'NONE',  ( -9.680171189290716072, 199.9079932115567146, 101.1988620819214475 ) ) ;
#5336=MECHANICAL_DESIGN_GEOMETRIC_PRESENTATION_REPRESENTATION('',(#21089),#32508);
#5340=CARTESIAN_POINT ( 'NONE',  ( 7.456977232089302632, 217.1783343296989131, 94.55113791807855250 ) ) ;
#5342=EDGE_CURVE ( 'NONE', #33380, #29176, #13632, .T. ) ;
#5345=CARTESIAN_POINT ( 'NONE',  ( -9.984503880673420539, 203.7031108863293980, 86.34886208192143897 ) ) ;
#5346=CARTESIAN_POINT ( 'NONE',  ( -3.662846001189865142, 195.5725841191952838, 22.89886208192143613 ) ) ;
#5348=CARTESIAN_POINT ( 'NONE',  ( 3.135527875058820690, 216.4958274776887492, 46.40113791807857524 ) ) ;
#5350=CARTESIAN_POINT ( 'NONE',  ( -7.984503880673422316, 204.3529502787951628, 5.348862081921435419 ) ) ;
#5354=CARTESIAN_POINT ( 'NONE',  ( -8.000000000000008882, 206.9523078486584780, 92.49886208192144466 ) ) ;
#5358=CARTESIAN_POINT ( 'NONE',  ( 2.426778023690261410, 199.3768101843759837, 29.60113791807856742 ) ) ;
#5365=CARTESIAN_POINT ( 'NONE',  ( -0.05014649552807731031, 198.5883022060938572, 89.75113791807858377 ) ) ;
#5368=CARTESIAN_POINT ( 'NONE',  ( 7.984503880673422316, 209.6470497212048372, 66.84886208192143897 ) ) ;
#5372=CARTESIAN_POINT ( 'NONE',  ( 8.062137200540920645, 201.0835637161417822, 5.301137918078566713 ) ) ;
#5376=CARTESIAN_POINT ( 'NONE',  ( 3.662846001190051659, 195.5725841191953691, 68.60113791807857808 ) ) ;
#5379=CARTESIAN_POINT ( 'NONE',  ( -10.01549611932653860, 203.7984951890123000, 87.35113791807856387 ) ) ;
#5383=CARTESIAN_POINT ( 'NONE',  ( 3.662846001189864698, 218.4274158808046593, 54.39886208192143613 ) ) ;
#5384=CARTESIAN_POINT ( 'NONE',  ( 0.05014649552828275708, 196.4853777576173002, 43.74886208192141623 ) ) ;
#5385=CARTESIAN_POINT ( 'NONE',  ( -6.139770520408224463, 198.4640165459539105, 53.04886208192142760 ) ) ;
#5386=CARTESIAN_POINT ( 'NONE',  ( 3.753561863808689836, 218.3979405102790565, 94.40113791807857524 ) ) ;
#5388=CARTESIAN_POINT ( 'NONE',  ( -8.118202686958039038, 201.1607312380087080, 9.201137918078565292 ) ) ;
#5389=CARTESIAN_POINT ( 'NONE',  ( 0.05014649552828275708, 196.4853777576173002, 76.74886208192140202 ) ) ;
#5392=CARTESIAN_POINT ( 'NONE',  ( 3.662846001189864698, 218.4274158808046593, 78.39886208192143613 ) ) ;
#5393=CARTESIAN_POINT ( 'NONE',  ( 8.062137200540920645, 201.0835637161417822, 95.30113791807858092 ) ) ;
#5396=CARTESIAN_POINT ( 'NONE',  ( 6.500168698208244500, 202.3363017425938324, 64.29886208192144181 ) ) ;
#5398=EDGE_CURVE ( 'NONE', #19921, #18219, #2644, .T. ) ;
#5406=CARTESIAN_POINT ( 'NONE',  ( 6.139770520408223575, 215.5359834540460611, 51.54886208192142050 ) ) ;
#5410=CARTESIAN_POINT ( 'NONE',  ( 2.517493886309087436, 199.4062855549015865, 31.59886208192144252 ) ) ;
#5411=CARTESIAN_POINT ( 'NONE',  ( 3.044812012440130555, 197.4746971517856764, 80.60113791807857808 ) ) ;
#5413=CARTESIAN_POINT ( 'NONE',  ( 6.220909254589536808, 215.4770327129947702, 52.55113791807858092 ) ) ;
#5414=CARTESIAN_POINT ( 'NONE',  ( 3.044812012440130555, 197.4746971517856764, 23.60113791807857098 ) ) ;
#5415=CARTESIAN_POINT ( 'NONE',  ( -2.426778023690262742, 214.6231898156240163, 13.10113791807856742 ) ) ;
#5419=CARTESIAN_POINT ( 'NONE',  ( 3.662846001190051659, 195.5725841191953691, 38.60113791807855677 ) ) ;
#5421=CARTESIAN_POINT ( 'NONE',  ( 10.00000000000000711, 206.9523078486586201, 83.00113791807856956 ) ) ;
#5422=CARTESIAN_POINT ( 'NONE',  ( -3.044812012440131443, 216.5253028482142952, 55.10113791807857098 ) ) ;
#5423=CARTESIAN_POINT ( 'NONE',  ( 9.736236675708031640, 199.9851607334238963, 19.29886208192143471 ) ) ;
#5424=CARTESIAN_POINT ( 'NONE',  ( 3.044812012439969795, 216.5253028482143520, 33.39886208192143613 ) ) ;
#5426=CARTESIAN_POINT ( 'NONE',  ( -0.05014649552807705357, 194.3824533091408000, 65.75113791807856956 ) ) ;
#5428=CARTESIAN_POINT ( 'NONE',  ( 6.500168698208129925, 211.6636982574063381, 91.70113791807857240 ) ) ;
#5430=CARTESIAN_POINT ( 'NONE',  ( 6.139770520408223575, 215.5359834540460611, 51.54886208192142050 ) ) ;
#5433=CARTESIAN_POINT ( 'NONE',  ( -11.98450388067341876, 203.0532714938636047, 56.34886208192143187 ) ) ;
#5434=EDGE_LOOP ( 'NONE', ( #26715, #23542, #17197, #8727, #19054 ) ) ;
#5440=CARTESIAN_POINT ( 'NONE',  ( 8.015496119326531499, 209.5516654185219636, 46.85113791807857098 ) ) ;
#5444=CARTESIAN_POINT ( 'NONE',  ( -10.00000000000000711, 206.9523078486584495, 20.49886208192143755 ) ) ;
#5448=CARTESIAN_POINT ( 'NONE',  ( -4.903702542908436435, 200.1653181626580249, 8.048862081921434708 ) ) ;
#5449=CARTESIAN_POINT ( 'NONE',  ( -6.139770520408369237, 215.5359834540460042, 39.95113791807857240 ) ) ;
#5452=CARTESIAN_POINT ( 'NONE',  ( 10.01549611932653860, 210.2015048109876716, 31.85113791807857453 ) ) ;
#5453=CARTESIAN_POINT ( 'NONE',  ( 0.05014649552828275014, 196.4853777576173002, 103.7488620819214589 ) ) ;
#5455=CARTESIAN_POINT ( 'NONE',  ( 8.015496119326595448, 204.4483345814782638, 94.14886208192145034 ) ) ;
#5460=CARTESIAN_POINT ( 'NONE',  ( -3.753561863808691168, 195.6020594897209435, 5.901137918078566358 ) ) ;
#5463=CARTESIAN_POINT ( 'NONE',  ( -3.044812012440131443, 216.5253028482142952, 55.10113791807857098 ) ) ;
#5464=CARTESIAN_POINT ( 'NONE',  ( 6.220909254589536808, 215.4770327129947987, 31.55113791807856671 ) ) ;
#5470=CARTESIAN_POINT ( 'NONE',  ( -3.753561863808691168, 195.6020594897209435, 35.90113791807856813 ) ) ;
#5472=CARTESIAN_POINT ( 'NONE',  ( 0.05014649552828275708, 196.4853777576173002, 22.74886208192142689 ) ) ;
#5475=CARTESIAN_POINT ( 'NONE',  ( 3.044812012440130555, 197.4746971517856764, 74.60113791807856387 ) ) ;
#5480=CARTESIAN_POINT ( 'NONE',  ( 6.500168698208129925, 211.6636982574063381, 10.70113791807856529 ) ) ;
#5481=CARTESIAN_POINT ( 'NONE',  ( 0.05014649552828288198, 194.3824533091408000, 94.74886208192144466 ) ) ;
#5487=CARTESIAN_POINT ( 'NONE',  ( -8.062137200540920645, 212.9164362838581894, 9.801137918078566713 ) ) ;
#5488=CARTESIAN_POINT ( 'NONE',  ( -6.220909254589682469, 215.4770327129946850, 77.94886208192140487 ) ) ;
#5491=CARTESIAN_POINT ( 'NONE',  ( -8.118202686958039038, 201.1607312380087080, 15.20113791807856884 ) ) ;
#5494=CARTESIAN_POINT ( 'NONE',  ( 9.984503880673470277, 203.7031108863295401, 101.1511379180785752 ) ) ;
#5496=CARTESIAN_POINT ( 'NONE',  ( 10.00000000000000711, 206.9523078486586201, 89.00113791807858377 ) ) ;
#5499=CARTESIAN_POINT ( 'NONE',  ( -3.662846001189865142, 195.5725841191952838, 97.89886208192146455 ) ) ;
#5504=CARTESIAN_POINT ( 'NONE',  ( -9.680171189290716072, 199.9079932115567146, 2.198862081921433731 ) ) ;
#5507=CARTESIAN_POINT ( 'NONE',  ( 9.984503880673420539, 210.2968891136705736, 93.84886208192143897 ) ) ;
#5509=CARTESIAN_POINT ( 'NONE',  ( -9.680171189290716072, 199.9079932115567146, 35.19886208192142618 ) ) ;
#5511=CARTESIAN_POINT ( 'NONE',  ( 0.05014649552810505201, 217.5146222423826714, 40.25113791807856956 ) ) ;
#5513=CARTESIAN_POINT ( 'NONE',  ( 6.444103211790928043, 211.7408657792734061, 3.698862081921435063 ) ) ;
#5516=CARTESIAN_POINT ( 'NONE',  ( 8.015496119326595448, 204.4483345814782638, 94.14886208192145034 ) ) ;
#5517=CARTESIAN_POINT ( 'NONE',  ( 2.426778023690261410, 199.3768101843759837, 32.60113791807857098 ) ) ;
#5523=CARTESIAN_POINT ( 'NONE',  ( 8.000000000000008882, 206.9523078486586485, 89.00113791807858377 ) ) ;
#5528=CARTESIAN_POINT ( 'NONE',  ( -8.015496119326597224, 209.5516654185217362, 65.64886208192142192 ) ) ;
#5531=CARTESIAN_POINT ( 'NONE',  ( 8.062137200540920645, 201.0835637161417822, 14.30113791807856671 ) ) ;
#5537=CARTESIAN_POINT ( 'NONE',  ( 9.736236675707914401, 214.0148392665762458, 64.70113791807857240 ) ) ;
#5539=CARTESIAN_POINT ( 'NONE',  ( 0.05014649552810506589, 217.5146222423826714, 91.25113791807858377 ) ) ;
#5542=CARTESIAN_POINT ( 'NONE',  ( -9.736236675708031640, 214.0148392665760753, 56.79886208192143471 ) ) ;
#5543=CARTESIAN_POINT ( 'NONE',  ( -6.139770520408224463, 198.4640165459539105, 65.04886208192144181 ) ) ;
#5544=CARTESIAN_POINT ( 'NONE',  ( -3.662846001190052991, 218.4274158808045740, 97.10113791807857808 ) ) ;
#5546=CARTESIAN_POINT ( 'NONE',  ( 3.135527875058820690, 216.4958274776887492, 16.40113791807856813 ) ) ;
#5547=CARTESIAN_POINT ( 'NONE',  ( 3.135527875058981895, 197.5041725223112792, 79.59886208192143897 ) ) ;
#5549=CARTESIAN_POINT ( 'NONE',  ( 6.220909254589536808, 215.4770327129947702, 100.5511379180785809 ) ) ;
#5553=CARTESIAN_POINT ( 'NONE',  ( -4.903702542908436435, 200.1653181626580249, 62.04886208192144181 ) ) ;
#5560=AXIS2_PLACEMENT_3D ( 'NONE', #21634, #10924, #23695 ) ;
#5562=CARTESIAN_POINT ( 'NONE',  ( -8.015496119326531499, 204.4483345814780364, 63.35113791807857098 ) ) ;
#5568=CARTESIAN_POINT ( 'NONE',  ( 8.015496119326595448, 204.4483345814782638, 37.14886208192143613 ) ) ;
#5569=CARTESIAN_POINT ( 'NONE',  ( -8.118202686958039038, 201.1607312380087080, 84.20113791807858661 ) ) ;
#5571=CARTESIAN_POINT ( 'NONE',  ( -9.984503880673473830, 210.2968891136704315, 63.65113791807857524 ) ) ;
#5574=CARTESIAN_POINT ( 'NONE',  ( 0.05014649552810505201, 217.5146222423826714, 25.25113791807856245 ) ) ;
#5575=CARTESIAN_POINT ( 'NONE',  ( 4.903702542908601636, 200.1653181626581102, 14.45113791807856707 ) ) ;
#5579=CARTESIAN_POINT ( 'NONE',  ( -9.736236675707914401, 199.9851607334237542, 36.20113791807856529 ) ) ;
#5581=CARTESIAN_POINT ( 'NONE',  ( 0.05014649552810505201, 217.5146222423826714, 85.25113791807854113 ) ) ;
#5582=CARTESIAN_POINT ( 'NONE',  ( -8.118202686958039038, 201.1607312380087080, 60.20113791807857240 ) ) ;
#5583=CARTESIAN_POINT ( 'NONE',  ( -9.680171189290716072, 199.9079932115567146, 20.19886208192143684 ) ) ;
#5584=CARTESIAN_POINT ( 'NONE',  ( -9.984503880673420539, 203.7031108863293980, 26.34886208192143187 ) ) ;
#5587=CARTESIAN_POINT ( 'NONE',  ( -3.662846001190052991, 218.4274158808045740, 64.10113791807857808 ) ) ;
#5588=CARTESIAN_POINT ( 'NONE',  ( -6.500168698208129925, 202.3363017425936050, 93.20113791807858661 ) ) ;
#5591=CARTESIAN_POINT ( 'NONE',  ( 6.139770520408223575, 215.5359834540460611, 54.54886208192144181 ) ) ;
#5593=ORIENTED_EDGE ( 'NONE', *, *, #5342, .F. ) ;
#5594=CARTESIAN_POINT ( 'NONE',  ( -7.456977232089471386, 217.1783343296987709, 56.94886208192144039 ) ) ;
#5602=CARTESIAN_POINT ( 'NONE',  ( -4.903702542908602524, 213.8346818373418898, 42.95113791807857240 ) ) ;
#5603=CARTESIAN_POINT ( 'NONE',  ( -6.220909254589682469, 215.4770327129946850, 20.94886208192143684 ) ) ;
#5610=CARTESIAN_POINT ( 'NONE',  ( 2.426778023690075337, 214.6231898156240447, 3.398862081921434797 ) ) ;
#5612=CARTESIAN_POINT ( 'NONE',  ( -8.118202686958039038, 201.1607312380087080, 51.20113791807857240 ) ) ;
#5614=CARTESIAN_POINT ( 'NONE',  ( 8.062137200540920645, 201.0835637161417822, 29.30113791807857027 ) ) ;
#5616=CARTESIAN_POINT ( 'NONE',  ( -0.05014649552828365914, 215.4116977939061144, 93.24886208192143044 ) ) ;
#5620=CARTESIAN_POINT ( 'NONE',  ( 9.680171189290831535, 199.9079932115568852, 14.30113791807856849 ) ) ;
#5624=CARTESIAN_POINT ( 'NONE',  ( 3.044812012440130555, 197.4746971517856764, 56.60113791807857098 ) ) ;
#5626=CARTESIAN_POINT ( 'NONE',  ( 8.118202686958039038, 212.8392687619912635, 28.70113791807856884 ) ) ;
#5630=CARTESIAN_POINT ( 'NONE',  ( 3.135527875058981895, 197.5041725223112792, 4.598862081921434530 ) ) ;
#5633=CARTESIAN_POINT ( 'NONE',  ( -12.00000000000000711, 207.0476921513413515, 36.50113791807857666 ) ) ;
#5636=CARTESIAN_POINT ( 'NONE',  ( -10.00000000000000711, 206.9523078486584495, 17.49886208192143400 ) ) ;
#5640=CARTESIAN_POINT ( 'NONE',  ( -0.05014649552810635652, 196.4853777576173002, 80.75113791807854113 ) ) ;
#5647=CARTESIAN_POINT ( 'NONE',  ( -4.984841277089726574, 200.2242689037092305, 9.051137918078564937 ) ) ;
#5648=CARTESIAN_POINT ( 'NONE',  ( -9.736236675708031640, 214.0148392665760753, 101.7988620819214560 ) ) ;
#5653=CARTESIAN_POINT ( 'NONE',  ( -3.044812012440131443, 216.5253028482142952, 7.101137918078566535 ) ) ;
#5655=CARTESIAN_POINT ( 'NONE',  ( 3.044812012439969795, 216.5253028482143520, 78.39886208192143613 ) ) ;
#5657=CARTESIAN_POINT ( 'NONE',  ( -8.062137200540920645, 212.9164362838581894, 21.80113791807856671 ) ) ;
#5661=CARTESIAN_POINT ( 'NONE',  ( 8.118202686958039038, 212.8392687619912635, 97.70113791807857240 ) ) ;
#5663=( BOUNDED_CURVE ( )  B_SPLINE_CURVE ( 2, ( #18418, #2758, #28479, #23528, #16020, #8200, #7535, #13298, #20643, #13461, #12800, #20971, #7699, #17922, #15355, #28970, #31366, #25744, #23691, #18082, #18585, #353, #33586, #5133, #5630, #32186, #29135, #16682, #9020, #24021, #11577, #6470, #32022, #21967, #21794, #8846, #19077, #18909, #29466, #16853, #32355, #5955, #29641, #16344, #19409, #16514, #19246, #6118, #21629, #13623, #6288, #684, #26738, #3400, #27246, #27079, #13796, #18750, #26568, #24190, #3742, #14131, #24525, #11087, #26913, #8686, #852, #8516, #3571, #11244, #1022, #13960, #21467, #3237, #1181, #24355, #29811, #3900, #8360, #14296, #24698, #11417, #1355, #21296, #16179, #31690, #5783, #31851, #29303, #9869, #17020, #32684, #12249, #1860, #27750, #19583, #9352, #4240, #22470, #19748, #30145, #32861, #27414, #9523, #25034, #17189, #4074, #25535, #22637, #1686, #19910, #7324, #12079, #30310, #6977, #6802, #9695, #17364, #4751, #11918, #27574, #30657, #22304, #11743, #4413, #14462, #14799, #7144, #15142, #17700, #25192, #33025, #9193, #17529, #14637, #20087, #22815, #30482, #22130, #20252, #32520, #27917, #4589, #14975, #28088, #25362, #2034, #12421, #33206, #29976, #6634, #24859, #1522, #31325, #7824, #311, #28924, #18212, #2203, #10386, #28769, #15309, #28268, #2374, #23652, #10710, #13094, #33378, #21091, #5584, #25701, #31493, #8160, #10052, #15809, #15648, #5254, #26047, #7991, #31156, #23484, #9740, #33541, #20758, #18542, #26202, #12585, #10554, #12763, #15979, #7489, #15486, #23153, #22978, #20429, #30822, #20599, #17873, #28434, #10217, #13256, #7657, #4923, #31001, #18040, #150, #5091, #18377, #25877, #2543, #2870, #12927, #23322, #28603, #2717, #20933, #5424, #31974, #24144, #24303, #3357, #8803, #13587, #16636, #29424, #6426, #18862, #26868, #29599, #21255, #32141, #29260, #13416, #19035, #24480, #31648, #23980, #3525, #16468, #8644, #483, #8315, #21579, #5911, #26528, #1142, #13748, #18709, #810, #16306, #31808, #29095, #26371, #13918, #26695, #11200, #21917, #6073, #974, #11373, #641, #21752, #29760, #11039, #19200, #6249, #11535, #3199, #3031, #27032, #5743, #3696, #14086, #23811, #32313, #8979, #19366, #10880, #16135, #21422, #8473, #1811, #1986, #17147, #3859, #32982, #12207, #22423, #14932, #9829, #32813, #7102, #17320, #4371, #14595, #14423, #24992, #12376, #17482, #27203, #25146, #11875, #4542, #12035, #27710, #1643, #27533, #9144, #14753, #29934, #22260, #32647, #22773, #22594, #9309, #14252, #22090, #1479, #9646, #24651, #20043, #6588, #9479, #4195, #19702, #4034, #19869, #30095, #30265, #6927, #19541, #32475, #30442, #27868, #25320, #33165, #1317, #20209, #30610, #16807, #11705, #16971, #27367, #24816, #6762, #28044, #33672, #5385, #12545, #28223, #7781, #31118, #23276, #15095, #4880, #33498, #18001, #15268, #25660, #13215, #15770, #28392, #20550, #12716, #22936, #21051, #18171, #30957, #5050, #2830, #7617, #15441, #25837, #2329, #5214, #2499, #277, #7441, #23110, #26163, #7950, #7274, #10347, #33332, #12883, #2675, #10672, #23612, #20718, #28566, #4706, #13055, #10170, #15600, #18333, #26003, #17657, #25491, #2162, #20387, #10003, #23445, #30780, #20891, #110, #10512, #31289, #28726, #17821, #31934, #18503, #16599, #24264, #11332, #8604, #10999, #32107, #19160, #31452, #13704, #26826, #29557, #2997, #18665, #19001, #21544, #24104, #5543, #29055, #23941, #8439, #5708, #16096, #3655, #6210, #771, #18826, #16429, #15934, #26994, #8770, #21379, #29220, #14049, #31772, #5872, #16271, #26491, #29391, #26657, #24445, #31610, #3159, #1109, #11502, #6038, #13376, #440, #11168, #3320, #8121, #28888, #3489, #13881, #26331, #934, #13549, #21717, #23774, #603, #10843, #21216, #8278, #1277, #14218, #22054, #9610, #20006, #32775, #19331, #30406, #7067, #22221, #8941, #4336, #17281, #27500, #17449, #14893, #4157, #12173, #22386, #9447, #19668, #19501, #30060, #27832, #22564, #32275, #30233, #11671, #4502, #17116, #19837, #6726, #32611, #24616, #6890, #32438, #16936, #27332, #25285, #27668, #3997, #29722, #27171, #6553, #14719, #6384, #25111, #1951, #32949, #21880, #9274, #14554, #16772, #1441, #24952, #1610, #12000, #1772, #3826, #9105, #29900, #11836, #14393, #24785, #12340, #28357, #7744, #26132, #17621, #33294, #12845, #2464, #5011, #20172, #9961, #4843, #23070, #20348, #30745, #18294, #20851, #15402, #33462, #31085, #30570, #10474, #13019, #7404, #10133, #7914, #25622, #2290, #20515, #17787, #10311, #12675, #5345, #12512, #28186, #31250, #23411, #33633, #28008, #15059, #25800, #17967, #28686, #30918, #7581, #23238, #9790, #18130, #15234, #20687, #74, #28529, #15734, #22736, #33123, #25454, #4674, #22901, #7233, #2128, #5178, #15563, #25960, #2635, #18627, #23578, #13667, #26619, #23903, #8569, #26782, #568, #11136, #8407, #18793, #16065, #2965, #26454, #29354, #21511, #13180, #5835, #5507, #16390, #13509, #31735, #3120, #29018, #18466, #29182, #28852, #400, #10803, #6002, #16230, #21177, #246, #31413, #23734, #3283, #10637, #24064, #31897, #15896, #5675, #31574, #26293, #10963, #8239, #21338, #735, #13343, #8082, #18961, #3449, #13845, #2799, #21014, #18404, #26077, #17906, #7352, #25733, #23010, #7855, #4953, #30689, #4780, #28300, #10414, #17732, #28628, #20958, #2232, #23513, #28797, #10252, #25901, #15839, #12790, #20627, #5120, #31029, #31186, #28464, #2747, #18, #20283, #5453, #13120, #181, #20787, #23180, #10580 ),
 .UNSPECIFIED., .F., .T. ) 
 B_SPLINE_CURVE_WITH_KNOTS ( ( 3, 2, 2, 2, 2, 2, 2, 2, 2, 2, 2, 2, 2, 2, 2, 2, 2, 2, 2, 2, 2, 2, 2, 2, 2, 2, 2, 2, 2, 2, 2, 2, 2, 2, 2, 2, 2, 2, 2, 2, 2, 2, 2, 2, 2, 2, 2, 2, 2, 2, 2, 2, 2, 2, 2, 2, 2, 2, 2, 2, 2, 2, 2, 2, 2, 2, 2, 2, 2, 2, 2, 2, 2, 2, 2, 2, 2, 2, 2, 2, 2, 2, 2, 2, 2, 2, 2, 2, 2, 2, 2, 2, 2, 2, 2, 2, 2, 2, 2, 2, 2, 2, 2, 2, 2, 2, 2, 2, 2, 2, 2, 2, 2, 2, 2, 2, 2, 2, 2, 2, 2, 2, 2, 2, 2, 2, 2, 2, 2, 2, 2, 2, 2, 2, 2, 2, 2, 2, 2, 2, 2, 2, 2, 2, 2, 2, 2, 2, 2, 2, 2, 2, 2, 2, 2, 2, 2, 2, 2, 2, 2, 2, 2, 2, 2, 2, 2, 2, 2, 2, 2, 2, 2, 2, 2, 2, 2, 2, 2, 2, 2, 2, 2, 2, 2, 2, 2, 2, 2, 2, 2, 2, 2, 2, 2, 2, 2, 2, 2, 2, 2, 2, 2, 2, 2, 2, 2, 2, 2, 2, 2, 2, 2, 2, 2, 2, 2, 2, 2, 2, 2, 2, 2, 2, 2, 2, 2, 2, 2, 2, 2, 2, 2, 2, 2, 2, 2, 2, 2, 2, 2, 2, 2, 2, 2, 2, 2, 2, 2, 2, 2, 2, 2, 2, 2, 2, 2, 2, 2, 2, 2, 2, 2, 2, 2, 2, 2, 2, 2, 2, 2, 2, 2, 2, 2, 2, 2, 2, 2, 2, 2, 2, 2, 2, 2, 2, 2, 2, 2, 2, 2, 2, 2, 2, 2, 2, 2, 2, 2, 2, 2, 2, 2, 2, 2, 2, 2, 2, 2, 2, 2, 2, 2, 2, 2, 2, 2, 2, 2, 2, 2, 2, 2, 2, 2, 2, 2, 2, 2, 2, 2, 2, 2, 2, 2, 2, 2, 2, 2, 2, 2, 2, 2, 2, 2, 3 ),
 ( 0.000000000000000000, 0.002857142857142857140, 0.005714285714285714281, 0.008571428571428571855, 0.01142857142857142856, 0.01428571428571428527, 0.01714285714285714371, 0.02000000000000000042, 0.02285714285714285712, 0.02571428571428571383, 0.02857142857142857054, 0.03142857142857143071, 0.03428571428571428742, 0.03714285714285714413, 0.04000000000000000083, 0.04285714285714285754, 0.04571428571428571425, 0.04857142857142857095, 0.05142857142857142766, 0.05428571428571428437, 0.05714285714285714107, 0.05999999999999999778, 0.06285714285714286143, 0.06571428571428571119, 0.06857142857142857484, 0.07142857142857142461, 0.07428571428571428825, 0.07714285714285713802, 0.08000000000000000167, 0.08285714285714285143, 0.08571428571428571508, 0.08857142857142855097, 0.09142857142857142849, 0.09428571428571429214, 0.09714285714285714191, 0.1000000000000000056, 0.1028571428571428553, 0.1057142857142857190, 0.1085714285714285687, 0.1114285714285714324, 0.1142857142857142821, 0.1171428571428571458, 0.1199999999999999956, 0.1228571428571428592, 0.1257142857142857229, 0.1285714285714285587, 0.1314285714285714224, 0.1342857142857142860, 0.1371428571428571497, 0.1400000000000000133, 0.1428571428571428492, 0.1457142857142857129, 0.1485714285714285765, 0.1514285714285714401, 0.1542857142857142760, 0.1571428571428571397, 0.1600000000000000033, 0.1628571428571428670, 0.1657142857142857029, 0.1685714285714285665, 0.1714285714285714302, 0.1742857142857142938, 0.1771428571428571019, 0.1799999999999999933, 0.1828571428571428570, 0.1857142857142857206, 0.1885714285714285843, 0.1914285714285714202, 0.1942857142857142838, 0.1971428571428571475, 0.2000000000000000111, 0.2028571428571428470, 0.2057142857142857106, 0.2085714285714285743, 0.2114285714285714379, 0.2142857142857142738, 0.2171428571428571375, 0.2200000000000000011, 0.2228571428571428648, 0.2257142857142857006, 0.2285714285714285643, 0.2314285714285714279, 0.2342857142857142916, 0.2371428571428571552, 0.2399999999999999911, 0.2428571428571428548, 0.2457142857142857184, 0.2485714285714285821, 0.2514285714285714457, 0.2542857142857142816, 0.2571428571428571175, 0.2600000000000000089, 0.2628571428571428448, 0.2657142857142857362, 0.2685714285714285721, 0.2714285714285714080, 0.2742857142857142994, 0.2771428571428571352, 0.2800000000000000266, 0.2828571428571428625, 0.2857142857142856984, 0.2885714285714285898, 0.2914285714285714257, 0.2942857142857142616, 0.2971428571428571530, 0.2999999999999999889, 0.3028571428571428803, 0.3057142857142857162, 0.3085714285714285521, 0.3114285714285714435, 0.3142857142857142794, 0.3171428571428571153, 0.3200000000000000067, 0.3228571428571428426, 0.3257142857142857340, 0.3285714285714285698, 0.3314285714285714057, 0.3342857142857142971, 0.3371428571428571330, 0.3400000000000000244, 0.3428571428571428603, 0.3457142857142856962, 0.3485714285714285876, 0.3514285714285714235, 0.3542857142857142039, 0.3571428571428571508, 0.3599999999999999867, 0.3628571428571428781, 0.3657142857142857140, 0.3685714285714285499, 0.3714285714285714413, 0.3742857142857142771, 0.3771428571428571686, 0.3800000000000000044, 0.3828571428571428403, 0.3857142857142857317, 0.3885714285714285676, 0.3914285714285714035, 0.3942857142857142949, 0.3971428571428571308, 0.4000000000000000222, 0.4028571428571428581, 0.4057142857142856940, 0.4085714285714285854, 0.4114285714285714213, 0.4142857142857143127, 0.4171428571428571486, 0.4199999999999999845, 0.4228571428571428759, 0.4257142857142857117, 0.4285714285714285476, 0.4314285714285714390, 0.4342857142857142749, 0.4371428571428571663, 0.4400000000000000022, 0.4428571428571428381, 0.4457142857142857295, 0.4485714285714285654, 0.4514285714285714013, 0.4542857142857142927, 0.4571428571428571286, 0.4600000000000000200, 0.4628571428571428559, 0.4657142857142856918, 0.4685714285714285832, 0.4714285714285714191, 0.4742857142857143105, 0.4771428571428571463, 0.4799999999999999822, 0.4828571428571428736, 0.4857142857142857095, 0.4885714285714285454, 0.4914285714285714368, 0.4942857142857142727, 0.4971428571428571641, 0.5000000000000000000, 0.5028571428571428914, 0.5057142857142856718, 0.5085714285714285632, 0.5114285714285714546, 0.5142857142857142350, 0.5171428571428571264, 0.5200000000000000178, 0.5228571428571429092, 0.5257142857142856895, 0.5285714285714285809, 0.5314285714285714723, 0.5342857142857142527, 0.5371428571428571441, 0.5400000000000000355, 0.5428571428571428159, 0.5457142857142857073, 0.5485714285714285987, 0.5514285714285713791, 0.5542857142857142705, 0.5571428571428571619, 0.5600000000000000533, 0.5628571428571428337, 0.5657142857142857251, 0.5685714285714286165, 0.5714285714285713969, 0.5742857142857142883, 0.5771428571428571797, 0.5799999999999999600, 0.5828571428571428514, 0.5857142857142857428, 0.5885714285714285232, 0.5914285714285714146, 0.5942857142857143060, 0.5971428571428571974, 0.5999999999999999778, 0.6028571428571428692, 0.6057142857142857606, 0.6085714285714285410, 0.6114285714285714324, 0.6142857142857143238, 0.6171428571428571042, 0.6199999999999999956, 0.6228571428571428870, 0.6257142857142856673, 0.6285714285714285587, 0.6314285714285714501, 0.6342857142857142305, 0.6371428571428571219, 0.6400000000000000133, 0.6428571428571429047, 0.6457142857142856851, 0.6485714285714285765, 0.6514285714285714679, 0.6542857142857142483, 0.6571428571428571397, 0.6600000000000000311, 0.6628571428571428115, 0.6657142857142857029, 0.6685714285714285943, 0.6714285714285713746, 0.6742857142857142660, 0.6771428571428571574, 0.6800000000000000488, 0.6828571428571428292, 0.6857142857142857206, 0.6885714285714286120, 0.6914285714285713924, 0.6942857142857142838, 0.6971428571428571752, 0.7000000000000000666, 0.7028571428571428470, 0.7057142857142857384, 0.7085714285714284077, 0.7114285714285714102, 0.7142857142857143016, 0.7171428571428571930, 0.7199999999999999734, 0.7228571428571428648, 0.7257142857142857562, 0.7285714285714285365, 0.7314285714285714279, 0.7342857142857143193, 0.7371428571428570997, 0.7399999999999999911, 0.7428571428571428825, 0.7457142857142856629, 0.7485714285714285543, 0.7514285714285714457, 0.7542857142857143371, 0.7571428571428571175, 0.7600000000000000089, 0.7628571428571429003, 0.7657142857142856807, 0.7685714285714285721, 0.7714285714285714635, 0.7742857142857142438, 0.7771428571428571352, 0.7800000000000000266, 0.7828571428571428070, 0.7857142857142856984, 0.7885714285714285898, 0.7914285714285714812, 0.7942857142857142616, 0.7971428571428571530, 0.8000000000000000444, 0.8028571428571428248, 0.8057142857142857162, 0.8085714285714286076, 0.8114285714285713880, 0.8142857142857142794, 0.8171428571428571708, 0.8199999999999999512, 0.8228571428571428426, 0.8257142857142857340, 0.8285714285714286254, 0.8314285714285714057, 0.8342857142857142971, 0.8371428571428571885, 0.8399999999999999689, 0.8428571428571428603, 0.8457142857142857517, 0.8485714285714285321, 0.8514285714285714235, 0.8542857142857143149, 0.8571428571428570953, 0.8599999999999999867, 0.8628571428571428781, 0.8657142857142857695, 0.8685714285714285499, 0.8714285714285714413, 0.8742857142857143327, 0.8771428571428571130, 0.8800000000000000044, 0.8828571428571428958, 0.8857142857142856762, 0.8885714285714285676, 0.8914285714285714590, 0.8942857142857142394, 0.8971428571428571308, 0.8999999999999999112, 0.9028571428571428026, 0.9057142857142856940, 0.9085714285714285854, 0.9114285714285714768, 0.9142857142857142572, 0.9171428571428571486, 0.9200000000000000400, 0.9228571428571428203, 0.9257142857142857117, 0.9285714285714286031, 0.9314285714285713835, 0.9342857142857142749, 0.9371428571428571663, 0.9399999999999999467, 0.9428571428571428381, 0.9457142857142857295, 0.9485714285714286209, 0.9514285714285714013, 0.9542857142857142927, 0.9571428571428571841, 0.9599999999999999645, 0.9628571428571428559, 0.9657142857142857473, 0.9685714285714285277, 0.9714285714285714191, 0.9742857142857143105, 0.9771428571428570908, 0.9799999999999999822, 0.9828571428571428736, 0.9852555582871577178 ),
 .UNSPECIFIED. ) 
 CURVE ( )  GEOMETRIC_REPRESENTATION_ITEM ( )  RATIONAL_B_SPLINE_CURVE ( ( 1.000000000000000000, 0.9510565162951535312, 1.000000000000000000, 0.9510565162951535312, 1.000000000000000000, 0.9510565162951535312, 1.000000000000000000, 0.9510565162951535312, 1.000000000000000000, 0.9510565162951535312, 1.000000000000000000, 0.9510565162951535312, 1.000000000000000000, 0.9510565162951535312, 1.000000000000000000, 0.9510565162951535312, 1.000000000000000000, 0.9510565162951535312, 1.000000000000000000, 0.9510565162951535312, 1.000000000000000000, 0.9510565162951535312, 1.000000000000000000, 0.9510565162951535312, 1.000000000000000000, 0.9510565162951535312, 1.000000000000000000, 0.9510565162951535312, 1.000000000000000000, 0.9510565162951535312, 1.000000000000000000, 0.9510565162951535312, 1.000000000000000000, 0.9510565162951535312, 1.000000000000000000, 0.9510565162951535312, 1.000000000000000000, 0.9510565162951535312, 1.000000000000000000, 0.9510565162951535312, 1.000000000000000000, 0.9510565162951535312, 1.000000000000000000, 0.9510565162951535312, 1.000000000000000000, 0.9510565162951535312, 1.000000000000000000, 0.9510565162951535312, 1.000000000000000000, 0.9510565162951535312, 1.000000000000000000, 0.9510565162951535312, 1.000000000000000000, 0.9510565162951535312, 1.000000000000000000, 0.9510565162951535312, 1.000000000000000000, 0.9510565162951535312, 1.000000000000000000, 0.9510565162951535312, 1.000000000000000000, 0.9510565162951535312, 1.000000000000000000, 0.9510565162951535312, 1.000000000000000000, 0.9510565162951535312, 1.000000000000000000, 0.9510565162951535312, 1.000000000000000000, 0.9510565162951535312, 1.000000000000000000, 0.9510565162951535312, 1.000000000000000000, 0.9510565162951535312, 1.000000000000000000, 0.9510565162951535312, 1.000000000000000000, 0.9510565162951535312, 1.000000000000000000, 0.9510565162951535312, 1.000000000000000000, 0.9510565162951535312, 1.000000000000000000, 0.9510565162951535312, 1.000000000000000000, 0.9510565162951535312, 1.000000000000000000, 0.9510565162951535312, 1.000000000000000000, 0.9510565162951535312, 1.000000000000000000, 0.9510565162951535312, 1.000000000000000000, 0.9510565162951535312, 1.000000000000000000, 0.9510565162951535312, 1.000000000000000000, 0.9510565162951535312, 1.000000000000000000, 0.9510565162951535312, 1.000000000000000000, 0.9510565162951535312, 1.000000000000000000, 0.9510565162951535312, 1.000000000000000000, 0.9510565162951535312, 1.000000000000000000, 0.9510565162951535312, 1.000000000000000000, 0.9510565162951535312, 1.000000000000000000, 0.9510565162951535312, 1.000000000000000000, 0.9510565162951535312, 1.000000000000000000, 0.9510565162951535312, 1.000000000000000000, 0.9510565162951535312, 1.000000000000000000, 0.9510565162951535312, 1.000000000000000000, 0.9510565162951535312, 1.000000000000000000, 0.9510565162951535312, 1.000000000000000000, 0.9510565162951535312, 1.000000000000000000, 0.9510565162951535312, 1.000000000000000000, 0.9510565162951535312, 1.000000000000000000, 0.9510565162951535312, 1.000000000000000000, 0.9510565162951535312, 1.000000000000000000, 0.9510565162951535312, 1.000000000000000000, 0.9510565162951535312, 1.000000000000000000, 0.9510565162951535312, 1.000000000000000000, 0.9510565162951535312, 1.000000000000000000, 0.9510565162951535312, 1.000000000000000000, 0.9510565162951535312, 1.000000000000000000, 0.9510565162951535312, 1.000000000000000000, 0.9510565162951535312, 1.000000000000000000, 0.9510565162951535312, 1.000000000000000000, 0.9510565162951535312, 1.000000000000000000, 0.9510565162951535312, 1.000000000000000000, 0.9510565162951535312, 1.000000000000000000, 0.9510565162951535312, 1.000000000000000000, 0.9510565162951535312, 1.000000000000000000, 0.9510565162951535312, 1.000000000000000000, 0.9510565162951535312, 1.000000000000000000, 0.9510565162951535312, 1.000000000000000000, 0.9510565162951535312, 1.000000000000000000, 0.9510565162951535312, 1.000000000000000000, 0.9510565162951535312, 1.000000000000000000, 0.9510565162951535312, 1.000000000000000000, 0.9510565162951535312, 1.000000000000000000, 0.9510565162951535312, 1.000000000000000000, 0.9510565162951535312, 1.000000000000000000, 0.9510565162951535312, 1.000000000000000000, 0.9510565162951535312, 1.000000000000000000, 0.9510565162951535312, 1.000000000000000000, 0.9510565162951535312, 1.000000000000000000, 0.9510565162951535312, 1.000000000000000000, 0.9510565162951535312, 1.000000000000000000, 0.9510565162951535312, 1.000000000000000000, 0.9510565162951535312, 1.000000000000000000, 0.9510565162951535312, 1.000000000000000000, 0.9510565162951535312, 1.000000000000000000, 0.9510565162951535312, 1.000000000000000000, 0.9510565162951535312, 1.000000000000000000, 0.9510565162951535312, 1.000000000000000000, 0.9510565162951535312, 1.000000000000000000, 0.9510565162951535312, 1.000000000000000000, 0.9510565162951535312, 1.000000000000000000, 0.9510565162951535312, 1.000000000000000000, 0.9510565162951535312, 1.000000000000000000, 0.9510565162951535312, 1.000000000000000000, 0.9510565162951535312, 1.000000000000000000, 0.9510565162951535312, 1.000000000000000000, 0.9510565162951535312, 1.000000000000000000, 0.9510565162951535312, 1.000000000000000000, 0.9510565162951535312, 1.000000000000000000, 0.9510565162951535312, 1.000000000000000000, 0.9510565162951535312, 1.000000000000000000, 0.9510565162951535312, 1.000000000000000000, 0.9510565162951535312, 1.000000000000000000, 0.9510565162951535312, 1.000000000000000000, 0.9510565162951535312, 1.000000000000000000, 0.9510565162951535312, 1.000000000000000000, 0.9510565162951535312, 1.000000000000000000, 0.9510565162951535312, 1.000000000000000000, 0.9510565162951535312, 1.000000000000000000, 0.9510565162951535312, 1.000000000000000000, 0.9510565162951535312, 1.000000000000000000, 0.9510565162951535312, 1.000000000000000000, 0.9510565162951535312, 1.000000000000000000, 0.9510565162951535312, 1.000000000000000000, 0.9510565162951535312, 1.000000000000000000, 0.9510565162951535312, 1.000000000000000000, 0.9510565162951535312, 1.000000000000000000, 0.9510565162951535312, 1.000000000000000000, 0.9510565162951535312, 1.000000000000000000, 0.9510565162951535312, 1.000000000000000000, 0.9510565162951535312, 1.000000000000000000, 0.9510565162951535312, 1.000000000000000000, 0.9510565162951535312, 1.000000000000000000, 0.9510565162951535312, 1.000000000000000000, 0.9510565162951535312, 1.000000000000000000, 0.9510565162951535312, 1.000000000000000000, 0.9510565162951535312, 1.000000000000000000, 0.9510565162951535312, 1.000000000000000000, 0.9510565162951535312, 1.000000000000000000, 0.9510565162951535312, 1.000000000000000000, 0.9510565162951535312, 1.000000000000000000, 0.9510565162951535312, 1.000000000000000000, 0.9510565162951535312, 1.000000000000000000, 0.9510565162951535312, 1.000000000000000000, 0.9510565162951535312, 1.000000000000000000, 0.9510565162951535312, 1.000000000000000000, 0.9510565162951535312, 1.000000000000000000, 0.9510565162951535312, 1.000000000000000000, 0.9510565162951535312, 1.000000000000000000, 0.9510565162951535312, 1.000000000000000000, 0.9510565162951535312, 1.000000000000000000, 0.9510565162951535312, 1.000000000000000000, 0.9510565162951535312, 1.000000000000000000, 0.9510565162951535312, 1.000000000000000000, 0.9510565162951535312, 1.000000000000000000, 0.9510565162951535312, 1.000000000000000000, 0.9510565162951535312, 1.000000000000000000, 0.9510565162951535312, 1.000000000000000000, 0.9510565162951535312, 1.000000000000000000, 0.9510565162951535312, 1.000000000000000000, 0.9510565162951535312, 1.000000000000000000, 0.9510565162951535312, 1.000000000000000000, 0.9510565162951535312, 1.000000000000000000, 0.9510565162951535312, 1.000000000000000000, 0.9510565162951535312, 1.000000000000000000, 0.9510565162951535312, 1.000000000000000000, 0.9510565162951535312, 1.000000000000000000, 0.9510565162951535312, 1.000000000000000000, 0.9510565162951535312, 1.000000000000000000, 0.9510565162951535312, 1.000000000000000000, 0.9510565162951535312, 1.000000000000000000, 0.9510565162951535312, 1.000000000000000000, 0.9510565162951535312, 1.000000000000000000, 0.9510565162951535312, 1.000000000000000000, 0.9510565162951535312, 1.000000000000000000, 0.9510565162951535312, 1.000000000000000000, 0.9510565162951535312, 1.000000000000000000, 0.9510565162951535312, 1.000000000000000000, 0.9510565162951535312, 1.000000000000000000, 0.9510565162951535312, 1.000000000000000000, 0.9510565162951535312, 1.000000000000000000, 0.9510565162951535312, 1.000000000000000000, 0.9510565162951535312, 1.000000000000000000, 0.9510565162951535312, 1.000000000000000000, 0.9510565162951535312, 1.000000000000000000, 0.9510565162951535312, 1.000000000000000000, 0.9510565162951535312, 1.000000000000000000, 0.9510565162951535312, 1.000000000000000000, 0.9510565162951535312, 1.000000000000000000, 0.9510565162951535312, 1.000000000000000000, 0.9510565162951535312, 1.000000000000000000, 0.9510565162951535312, 1.000000000000000000, 0.9510565162951535312, 1.000000000000000000, 0.9510565162951535312, 1.000000000000000000, 0.9510565162951535312, 1.000000000000000000, 0.9510565162951535312, 1.000000000000000000, 0.9510565162951535312, 1.000000000000000000, 0.9510565162951535312, 1.000000000000000000, 0.9510565162951535312, 1.000000000000000000, 0.9510565162951535312, 1.000000000000000000, 0.9510565162951535312, 1.000000000000000000, 0.9510565162951535312, 1.000000000000000000, 0.9510565162951535312, 1.000000000000000000, 0.9510565162951535312, 1.000000000000000000, 0.9510565162951535312, 1.000000000000000000, 0.9510565162951535312, 1.000000000000000000, 0.9510565162951535312, 1.000000000000000000, 0.9510565162951535312, 1.000000000000000000, 0.9510565162951535312, 1.000000000000000000, 0.9510565162951535312, 1.000000000000000000, 0.9510565162951535312, 1.000000000000000000, 0.9510565162951535312, 1.000000000000000000, 0.9510565162951535312, 1.000000000000000000, 0.9510565162951535312, 1.000000000000000000, 0.9510565162951535312, 1.000000000000000000, 0.9510565162951535312, 1.000000000000000000, 0.9510565162951535312, 1.000000000000000000, 0.9510565162951535312, 1.000000000000000000, 0.9510565162951535312, 1.000000000000000000, 0.9510565162951535312, 1.000000000000000000, 0.9510565162951535312, 1.000000000000000000, 0.9510565162951535312, 1.000000000000000000, 0.9510565162951535312, 1.000000000000000000, 0.9510565162951535312, 1.000000000000000000, 0.9510565162951535312, 1.000000000000000000, 0.9510565162951535312, 1.000000000000000000, 0.9510565162951535312, 1.000000000000000000, 0.9510565162951535312, 1.000000000000000000, 0.9510565162951535312, 1.000000000000000000, 0.9510565162951535312, 1.000000000000000000, 0.9510565162951535312, 1.000000000000000000, 0.9510565162951535312, 1.000000000000000000, 0.9510565162951535312, 1.000000000000000000, 0.9510565162951535312, 1.000000000000000000, 0.9510565162951535312, 1.000000000000000000, 0.9510565162951535312, 1.000000000000000000, 0.9510565162951535312, 1.000000000000000000, 0.9510565162951535312, 1.000000000000000000, 0.9510565162951535312, 1.000000000000000000, 0.9510565162951535312, 1.000000000000000000, 0.9510565162951535312, 1.000000000000000000, 0.9510565162951535312, 1.000000000000000000, 0.9510565162951535312, 1.000000000000000000, 0.9510565162951535312, 1.000000000000000000, 0.9510565162951535312, 1.000000000000000000, 0.9510565162951535312, 1.000000000000000000, 0.9510565162951535312, 1.000000000000000000, 0.9510565162951535312, 1.000000000000000000, 0.9510565162951535312, 1.000000000000000000, 0.9510565162951535312, 1.000000000000000000, 0.9510565162951535312, 1.000000000000000000, 0.9510565162951535312, 1.000000000000000000, 0.9510565162951535312, 1.000000000000000000, 0.9510565162951535312, 1.000000000000000000, 0.9510565162951535312, 1.000000000000000000, 0.9510565162951535312, 1.000000000000000000, 0.9510565162951535312, 1.000000000000000000, 0.9510565162951535312, 1.000000000000000000, 0.9510565162951535312, 1.000000000000000000, 0.9510565162951535312, 1.000000000000000000, 0.9510565162951535312, 1.000000000000000000, 0.9510565162951535312, 1.000000000000000000, 0.9510565162951535312, 1.000000000000000000, 0.9510565162951535312, 1.000000000000000000, 0.9510565162951535312, 1.000000000000000000, 0.9510565162951535312, 1.000000000000000000, 0.9510565162951535312, 1.000000000000000000, 0.9510565162951535312, 1.000000000000000000, 0.9510565162951535312, 1.000000000000000000, 0.9510565162951535312, 1.000000000000000000, 0.9510565162951535312, 1.000000000000000000, 0.9510565162951535312, 1.000000000000000000, 0.9510565162951535312, 1.000000000000000000, 0.9510565162951535312, 1.000000000000000000, 0.9510565162951535312, 1.000000000000000000, 0.9510565162951535312, 1.000000000000000000, 0.9510565162951535312, 1.000000000000000000, 0.9510565162951535312, 1.000000000000000000, 0.9510565162951535312, 1.000000000000000000, 0.9510565162951535312, 1.000000000000000000, 0.9510565162951535312, 1.000000000000000000, 0.9510565162951535312, 1.000000000000000000, 0.9510565162951535312, 1.000000000000000000, 0.9510565162951535312, 1.000000000000000000, 0.9510565162951535312, 1.000000000000000000, 0.9510565162951535312, 1.000000000000000000, 0.9510565162951535312, 1.000000000000000000, 0.9510565162951535312, 1.000000000000000000, 0.9510565162951535312, 1.000000000000000000, 0.9510565162951535312, 1.000000000000000000, 0.9510565162951535312, 1.000000000000000000, 0.9510565162951535312, 1.000000000000000000, 0.9510565162951535312, 1.000000000000000000, 0.9510565162951535312, 1.000000000000000000, 0.9510565162951535312, 1.000000000000000000, 0.9510565162951535312, 1.000000000000000000, 0.9510565162951535312, 1.000000000000000000, 0.9510565162951535312, 1.000000000000000000, 0.9510565162951535312, 1.000000000000000000, 0.9510565162951535312, 1.000000000000000000, 0.9510565162951535312, 1.000000000000000000, 0.9510565162951535312, 1.000000000000000000, 0.9510565162951535312, 1.000000000000000000, 0.9510565162951535312, 1.000000000000000000, 0.9510565162951535312, 1.000000000000000000, 0.9510565162951535312, 1.000000000000000000, 0.9510565162951535312, 1.000000000000000000, 0.9510565162951535312, 1.000000000000000000, 0.9510565162951535312, 1.000000000000000000, 0.9510565162951535312, 1.000000000000000000, 0.9510565162951535312, 1.000000000000000000, 0.9510565162951535312, 1.000000000000000000, 0.9510565162951535312, 1.000000000000000000, 0.9510565162951535312, 1.000000000000000000, 0.9510565162951535312, 1.000000000000000000, 0.9510565162951535312, 1.000000000000000000, 0.9510565162951535312, 1.000000000000000000, 0.9510565162951535312, 1.000000000000000000, 0.9510565162951535312, 1.000000000000000000, 0.9510565162951535312, 1.000000000000000000, 0.9510565162951535312, 1.000000000000000000, 0.9510565162951535312, 1.000000000000000000, 0.9510565162951535312, 1.000000000000000000, 0.9510565162951535312, 1.000000000000000000, 0.9510565162951535312, 1.000000000000000000, 0.9510565162951535312, 1.000000000000000000, 0.9510565162951535312, 1.000000000000000000, 0.9510565162951535312, 1.000000000000000000, 0.9510565162951535312, 1.000000000000000000, 0.9510565162951535312, 1.000000000000000000, 0.9510565162951535312, 1.000000000000000000, 0.9510565162951535312, 1.000000000000000000, 0.9510565162951535312, 1.000000000000000000, 0.9510565162951535312, 1.000000000000000000, 0.9510565162951535312, 1.000000000000000000, 0.9510565162951535312, 1.000000000000000000, 0.9510565162951535312, 1.000000000000000000, 0.9510565162951535312, 1.000000000000000000, 0.9589146177192661158, 0.9868071058056508971 ) ) 
 REPRESENTATION_ITEM ( '' )  );
#5664=CARTESIAN_POINT ( 'NONE',  ( 8.062137200540920645, 201.0835637161417822, 86.30113791807856671 ) ) ;
#5667=CARTESIAN_POINT ( 'NONE',  ( -11.98450388067341876, 203.0532714938636047, 92.34886208192143897 ) ) ;
#5675=CARTESIAN_POINT ( 'NONE',  ( 10.01549611932659367, 203.7984951890124421, 97.14886208192145034 ) ) ;
#5676=CARTESIAN_POINT ( 'NONE',  ( 9.736236675708031640, 199.9851607334238963, 34.29886208192143471 ) ) ;
#5678=CARTESIAN_POINT ( 'NONE',  ( 0.05014649552810505201, 217.5146222423826714, 43.25113791807856956 ) ) ;
#5680=CARTESIAN_POINT ( 'NONE',  ( 4.903702542908435547, 213.8346818373419751, 6.548862081921434708 ) ) ;
#5684=CARTESIAN_POINT ( 'NONE',  ( 0.05014649552828262524, 198.5883022060938572, 94.74886208192144466 ) ) ;
#5685=CARTESIAN_POINT ( 'NONE',  ( -6.444103211791042618, 211.7408657792732356, 33.80113791807857382 ) ) ;
#5691=CARTESIAN_POINT ( 'NONE',  ( 4.903702542908601636, 200.1653181626581102, 86.45113791807858661 ) ) ;
#5694=CARTESIAN_POINT ( 'NONE',  ( 2.426778023690075337, 214.6231898156240447, 69.39886208192143613 ) ) ;
#5697=CARTESIAN_POINT ( 'NONE',  ( -8.118202686958039038, 201.1607312380087080, 6.201137918078566180 ) ) ;
#5702=CARTESIAN_POINT ( 'NONE',  ( 7.375838497908181246, 196.7627149292499666, 77.45113791807855819 ) ) ;
#5704=CARTESIAN_POINT ( 'NONE',  ( 6.220909254589536808, 215.4770327129947987, 97.55113791807856671 ) ) ;
#5707=CARTESIAN_POINT ( 'NONE',  ( 3.753561863808876797, 195.6020594897209719, 61.59886208192143897 ) ) ;
#5708=CARTESIAN_POINT ( 'NONE',  ( -10.01549611932659545, 210.2015048109875011, 65.64886208192143613 ) ) ;
#5709=CARTESIAN_POINT ( 'NONE',  ( -3.662846001189865142, 195.5725841191952838, 7.898862081921435241 ) ) ;
#5711=CARTESIAN_POINT ( 'NONE',  ( 6.139770520408368348, 198.4640165459539674, 17.45113791807855819 ) ) ;
#5712=CARTESIAN_POINT ( 'NONE',  ( 0.05014649552828275708, 196.4853777576173002, 82.74886208192143044 ) ) ;
#5713=EDGE_CURVE ( 'NONE', #4391, #22743, #16746, .T. ) ;
#5715=CARTESIAN_POINT ( 'NONE',  ( 6.139770520408368348, 198.4640165459539674, 101.4511379180785866 ) ) ;
#5718=CARTESIAN_POINT ( 'NONE',  ( 4.984841277089891776, 200.2242689037093726, 64.44886208192143329 ) ) ;
#5724=CARTESIAN_POINT ( 'NONE',  ( -6.444103211791042618, 211.7408657792732356, 63.80113791807858092 ) ) ;
#5729=CARTESIAN_POINT ( 'NONE',  ( 6.500168698208244500, 202.3363017425938324, 40.29886208192144181 ) ) ;
#5730=CARTESIAN_POINT ( 'NONE',  ( 8.062137200540920645, 201.0835637161417822, 77.30113791807858092 ) ) ;
#5732=CARTESIAN_POINT ( 'NONE',  ( 6.139770520408368348, 198.4640165459539674, 62.45113791807857950 ) ) ;
#5734=CARTESIAN_POINT ( 'NONE',  ( 4.903702542908601636, 200.1653181626581102, 17.45113791807856174 ) ) ;
#5738=CARTESIAN_POINT ( 'NONE',  ( 3.753561863808689836, 218.3979405102790565, 46.40113791807856813 ) ) ;
#5739=DIRECTION ( 'NONE',  ( -0.1461455375466716444, 0.9854922318508084755, -0.08629335326029916042 ) ) ;
#5740=CARTESIAN_POINT ( 'NONE',  ( 10.01549611932653860, 210.2015048109876716, 91.85113791807853545 ) ) ;
#5741=CARTESIAN_POINT ( 'NONE',  ( 8.062137200540920645, 201.0835637161417822, 68.30113791807856671 ) ) ;
#5742=CARTESIAN_POINT ( 'NONE',  ( -7.456977232089471386, 217.1783343296987709, 26.94886208192142973 ) ) ;
#5743=CARTESIAN_POINT ( 'NONE',  ( -10.00000000000000711, 206.9523078486584495, 41.49886208192143044 ) ) ;
#5745=CARTESIAN_POINT ( 'NONE',  ( -3.662846001190052991, 218.4274158808045740, 73.10113791807857808 ) ) ;
#5746=CARTESIAN_POINT ( 'NONE',  ( 8.015496119326531499, 209.5516654185219636, 91.85113791807857808 ) ) ;
#5747=CARTESIAN_POINT ( 'NONE',  ( -8.062137200540822946, 201.0835637161416400, 50.19886208192144039 ) ) ;
#5751=CARTESIAN_POINT ( 'NONE',  ( 3.662846001189864698, 218.4274158808046593, 48.39886208192143613 ) ) ;
#5758=CARTESIAN_POINT ( 'NONE',  ( 6.500168698208129925, 211.6636982574063381, 55.70113791807857240 ) ) ;
#5760=CARTESIAN_POINT ( 'NONE',  ( 3.135527875058981895, 197.5041725223112792, 31.59886208192143187 ) ) ;
#5765=CARTESIAN_POINT ( 'NONE',  ( 6.444103211790928043, 211.7408657792734061, 9.698862081921433287 ) ) ;
#5766=CARTESIAN_POINT ( 'NONE',  ( -0.05014649552810635652, 196.4853777576173002, 53.75113791807857666 ) ) ;
#5769=CARTESIAN_POINT ( 'NONE',  ( -10.01549611932653860, 203.7984951890123284, 39.35113791807857098 ) ) ;
#5771=CARTESIAN_POINT ( 'NONE',  ( -2.426778023690076225, 199.3768101843759553, 88.89886208192143613 ) ) ;
#5775=CARTESIAN_POINT ( 'NONE',  ( 11.98450388067348271, 203.0532714938637753, 8.151137918078566358 ) ) ;
#5779=CARTESIAN_POINT ( 'NONE',  ( 6.220909254589536808, 215.4770327129947702, 64.55113791807858092 ) ) ;
#5780=CARTESIAN_POINT ( 'NONE',  ( 3.135527875058820690, 216.4958274776887492, 31.40113791807857524 ) ) ;
#5783=CARTESIAN_POINT ( 'NONE',  ( -3.044812012439970683, 197.4746971517856196, 13.89886208192143613 ) ) ;
#5786=CARTESIAN_POINT ( 'NONE',  ( -11.98450388067348804, 210.9467285061362247, 39.65113791807857524 ) ) ;
#5788=CARTESIAN_POINT ( 'NONE',  ( 9.984503880673420539, 210.2968891136705167, 21.84886208192143542 ) ) ;
#5792=CARTESIAN_POINT ( 'NONE',  ( -3.044812012440131443, 216.5253028482142952, 82.10113791807857808 ) ) ;
#5797=CARTESIAN_POINT ( 'NONE',  ( 4.903702542908601636, 200.1653181626581102, 14.45113791807856707 ) ) ;
#5802=CARTESIAN_POINT ( 'NONE',  ( 11.98450388067341876, 210.9467285061363953, 96.84886208192143897 ) ) ;
#5810=CARTESIAN_POINT ( 'NONE',  ( -10.01549611932659722, 210.2015048109875011, 83.64886208192143613 ) ) ;
#5812=CARTESIAN_POINT ( 'NONE',  ( -9.984503880673473830, 210.2968891136704315, 24.65113791807856103 ) ) ;
#5815=CARTESIAN_POINT ( 'NONE',  ( 3.753561863808876797, 195.6020594897209719, 79.59886208192143897 ) ) ;
#5820=CARTESIAN_POINT ( 'NONE',  ( 10.01549611932653860, 210.2015048109876716, 85.85113791807857808 ) ) ;
#5824=CARTESIAN_POINT ( 'NONE',  ( -7.375838497908014268, 196.7627149292498530, 98.04886208192144181 ) ) ;
#5829=CARTESIAN_POINT ( 'NONE',  ( -7.375838497908182134, 217.2372850707499765, 12.95113791807856707 ) ) ;
#5835=CARTESIAN_POINT ( 'NONE',  ( 8.062137200540822946, 212.9164362838583315, 93.69886208192143329 ) ) ;
#5836=CARTESIAN_POINT ( 'NONE',  ( -9.736236675708031640, 214.0148392665760753, 35.79886208192143471 ) ) ;
#5837=CARTESIAN_POINT ( 'NONE',  ( -10.47863426674271814, 207.9189531262114770, 102.6635298682156758 ) ) ;
#5838=CARTESIAN_POINT ( 'NONE',  ( -6.220909254589537696, 198.5229672870051161, 51.05113791807856671 ) ) ;
#5840=CARTESIAN_POINT ( 'NONE',  ( -7.984503880673422316, 204.3529502787951628, 2.348862081921434974 ) ) ;
#5844=CARTESIAN_POINT ( 'NONE',  ( -2.426778023690076225, 199.3768101843759553, 88.89886208192143613 ) ) ;
#5846=CARTESIAN_POINT ( 'NONE',  ( -8.015496119326531499, 204.4483345814780364, 30.35113791807856742 ) ) ;
#5853=CARTESIAN_POINT ( 'NONE',  ( -8.000000000000008882, 207.0476921513413515, 102.5011379180785696 ) ) ;
#5856=CARTESIAN_POINT ( 'NONE',  ( -0.05014649552828365914, 215.4116977939061144, 75.24886208192143044 ) ) ;
#5860=CARTESIAN_POINT ( 'NONE',  ( 8.062137200540920645, 201.0835637161417822, 11.30113791807856671 ) ) ;
#5865=CARTESIAN_POINT ( 'NONE',  ( 11.98450388067348271, 203.0532714938637753, 80.15113791807857524 ) ) ;
#5867=CARTESIAN_POINT ( 'NONE',  ( 9.984503880673473830, 203.7031108863295401, 95.15113791807857524 ) ) ;
#5870=CARTESIAN_POINT ( 'NONE',  ( -3.753561863808878130, 218.3979405102790281, 102.0988620819214532 ) ) ;
#5871=CARTESIAN_POINT ( 'NONE',  ( -9.736236675708031640, 214.0148392665760753, 59.79886208192143471 ) ) ;
#5872=CARTESIAN_POINT ( 'NONE',  ( 0.05014649552828275014, 196.4853777576173002, 67.74886208192141623 ) ) ;
#5873=CARTESIAN_POINT ( 'NONE',  ( 0.05014649552828288198, 194.3824533091408000, 1.748862081921433775 ) ) ;
#5876=CARTESIAN_POINT ( 'NONE',  ( 3.135527875058820690, 216.4958274776887492, 25.40113791807856813 ) ) ;
#5877=CARTESIAN_POINT ( 'NONE',  ( -9.984503880673420539, 203.7031108863293980, 80.34886208192143897 ) ) ;
#5880=CIRCLE ( 'NONE', #24423, 1.000000000000000888 ) ;
#5881=CARTESIAN_POINT ( 'NONE',  ( 3.135527875058820690, 216.4958274776887492, 97.40113791807858945 ) ) ;
#5883=CARTESIAN_POINT ( 'NONE',  ( 6.444103211790928043, 211.7408657792734061, 57.69886208192144039 ) ) ;
#5887=FACE_OUTER_BOUND ( 'NONE', #9103, .T. ) ;
#5890=CARTESIAN_POINT ( 'NONE',  ( -4.984841277089726574, 200.2242689037092305, 72.05113791807858092 ) ) ;
#5895=CARTESIAN_POINT ( 'NONE',  ( 7.984503880673422316, 209.6470497212048372, 39.84886208192144608 ) ) ;
#5897=CARTESIAN_POINT ( 'NONE',  ( -9.984503880673473830, 210.2968891136704315, 81.65113791807857524 ) ) ;
#5898=CARTESIAN_POINT ( 'NONE',  ( 6.139770520408368348, 198.4640165459539674, 68.45113791807858661 ) ) ;
#5901=CARTESIAN_POINT ( 'NONE',  ( -7.984503880673488041, 209.6470497212046098, 24.65113791807857169 ) ) ;
#5905=CARTESIAN_POINT ( 'NONE',  ( 12.00000000000000711, 206.9523078486586485, 50.00113791807856956 ) ) ;
#5907=CARTESIAN_POINT ( 'NONE',  ( -9.984503880673473830, 210.2968891136704315, 99.65113791807853261 ) ) ;
#5908=CARTESIAN_POINT ( 'NONE',  ( 10.00000000000000711, 206.9523078486586201, 71.00113791807858377 ) ) ;
#5910=CARTESIAN_POINT ( 'NONE',  ( 11.98450388067341876, 210.9467285061363953, 30.84886208192143542 ) ) ;
#5911=CARTESIAN_POINT ( 'NONE',  ( 6.220909254589680693, 198.5229672870052582, 37.44886208192143329 ) ) ;
#5913=CARTESIAN_POINT ( 'NONE',  ( -7.375838497908182134, 217.2372850707499765, 75.95113791807857240 ) ) ;
#5914=CARTESIAN_POINT ( 'NONE',  ( -6.444103211791042618, 211.7408657792732356, 90.80113791807858092 ) ) ;
#5915=CARTESIAN_POINT ( 'NONE',  ( -3.135527875058982783, 216.4958274776886924, 48.09886208192143187 ) ) ;
#5918=CARTESIAN_POINT ( 'NONE',  ( -3.662846001189865142, 195.5725841191952838, 58.89886208192143613 ) ) ;
#5919=ORIENTED_EDGE ( 'NONE', *, *, #24563, .F. ) ;
#5920=CARTESIAN_POINT ( 'NONE',  ( 2.517493886309087436, 199.4062855549015865, 28.59886208192143897 ) ) ;
#5922=ORIENTED_EDGE ( 'NONE', *, *, #19778, .F. ) ;
#5927=CARTESIAN_POINT ( 'NONE',  ( -2.426778023690262742, 214.6231898156240163, 52.10113791807857808 ) ) ;
#5930=CARTESIAN_POINT ( 'NONE',  ( -6.220909254589682469, 215.4770327129946850, 29.94886208192142973 ) ) ;
#5935=CARTESIAN_POINT ( 'NONE',  ( 0.05014649552828262524, 198.5883022060938572, 10.74886208192143577 ) ) ;
#5936=CARTESIAN_POINT ( 'NONE',  ( -0.05014649552810635652, 196.4853777576173002, 47.75113791807855534 ) ) ;
#5939=CARTESIAN_POINT ( 'NONE',  ( -3.135527875058821579, 197.5041725223112223, 35.90113791807856813 ) ) ;
#5942=CARTESIAN_POINT ( 'NONE',  ( 6.500168698208244500, 202.3363017425938324, 103.2988620819214560 ) ) ;
#5946=CARTESIAN_POINT ( 'NONE',  ( 11.98450388067348271, 203.0532714938637753, 17.15113791807856458 ) ) ;
#5950=CARTESIAN_POINT ( 'NONE',  ( -8.062137200540920645, 212.9164362838581894, 66.80113791807858092 ) ) ;
#5951=CARTESIAN_POINT ( 'NONE',  ( -6.220909254589537696, 198.5229672870051445, 36.05113791807857382 ) ) ;
#5954=DIRECTION ( 'NONE',  ( 0.000000000000000000, -0.04769215134144032253, 0.9988620819214358848 ) ) ;
#5955=CARTESIAN_POINT ( 'NONE',  ( 10.01549611932659367, 203.7984951890124421, 7.148862081921434353 ) ) ;
#5958=CARTESIAN_POINT ( 'NONE',  ( 9.680171189290831535, 199.9079932115568852, 53.30113791807857382 ) ) ;
#5960=CARTESIAN_POINT ( 'NONE',  ( -0.05014649552828403384, 217.5146222423826714, 24.24886208192143044 ) ) ;
#5964=CARTESIAN_POINT ( 'NONE',  ( 8.118202686958039038, 212.8392687619912635, 82.70113791807857240 ) ) ;
#5969=CARTESIAN_POINT ( 'NONE',  ( 2.517493886308900919, 214.5937144450984420, 22.40113791807856813 ) ) ;
#5972=CARTESIAN_POINT ( 'NONE',  ( 0.05014649552828288198, 194.3824533091408000, 103.7488620819214304 ) ) ;
#5974=EDGE_LOOP ( 'NONE', ( #14432, #4083, #28401, #9374, #13970, #33637, #21138 ) ) ;
#5979=CARTESIAN_POINT ( 'NONE',  ( 10.00000000000000711, 207.0476921513415220, 93.99886208192144466 ) ) ;
#5981=CARTESIAN_POINT ( 'NONE',  ( -3.044812012440131443, 216.5253028482142952, 25.10113791807856742 ) ) ;
#5984=CARTESIAN_POINT ( 'NONE',  ( 3.662846001189864698, 218.4274158808046593, 78.39886208192143613 ) ) ;
#5989=CARTESIAN_POINT ( 'NONE',  ( -9.984503880673473830, 210.2968891136704315, 90.65113791807854682 ) ) ;
#5992=CARTESIAN_POINT ( 'NONE',  ( -3.135527875058821579, 197.5041725223112223, 38.90113791807857524 ) ) ;
#5995=ORIENTED_EDGE ( 'NONE', *, *, #5713, .T. ) ;
#5998=CARTESIAN_POINT ( 'NONE',  ( -3.753561863808691168, 195.6020594897209435, 23.90113791807857169 ) ) ;
#6002=CARTESIAN_POINT ( 'NONE',  ( -10.00000000000000711, 206.9523078486584495, 95.49886208192144466 ) ) ;
#6003=CARTESIAN_POINT ( 'NONE',  ( 3.753561863808876797, 195.6020594897209719, 31.59886208192143187 ) ) ;
#6005=CARTESIAN_POINT ( 'NONE',  ( 3.044812012440130555, 197.4746971517856764, 47.60113791807857098 ) ) ;
#6008=CARTESIAN_POINT ( 'NONE',  ( -4.903702542908436435, 200.1653181626580249, 14.04886208192143471 ) ) ;
#6010=ORIENTED_EDGE ( 'NONE', *, *, #9130, .F. ) ;
#6011=CARTESIAN_POINT ( 'NONE',  ( 6.444103211790928043, 211.7408657792734061, 102.6988620819214475 ) ) ;
#6012=CARTESIAN_POINT ( 'NONE',  ( -8.015496119326531499, 204.4483345814780364, 42.35113791807857098 ) ) ;
#6016=CARTESIAN_POINT ( 'NONE',  ( -6.220909254589682469, 215.4770327129946850, 50.94886208192141908 ) ) ;
#6019=CARTESIAN_POINT ( 'NONE',  ( 8.000000000000008882, 206.9523078486586485, 101.0011379180785696 ) ) ;
#6022=CARTESIAN_POINT ( 'NONE',  ( -2.517493886309087880, 214.5937144450984135, 72.09886208192142476 ) ) ;
#6023=DIRECTION ( 'NONE',  ( -0.08583835255247916629, -0.09953364313786493278, -0.9913247858874408847 ) ) ;
#6025=CARTESIAN_POINT ( 'NONE',  ( -0.05014649552810635652, 196.4853777576173002, 11.75113791807856600 ) ) ;
#6030=CARTESIAN_POINT ( 'NONE',  ( 12.00000000000000711, 206.9523078486586485, 80.00113791807856956 ) ) ;
#6033=CARTESIAN_POINT ( 'NONE',  ( 3.135527875058820690, 216.4958274776887492, 97.40113791807858945 ) ) ;
#6034=CARTESIAN_POINT ( 'NONE',  ( -10.34113947703223424, 207.9902438215976872, 102.7420191180251692 ) ) ;
#6036=CARTESIAN_POINT ( 'NONE',  ( 7.375838497908012492, 217.2372850707501186, 102.5488620819214560 ) ) ;
#6037=CARTESIAN_POINT ( 'NONE',  ( -12.00000000000000711, 206.9523078486584780, 59.49886208192143044 ) ) ;
#6038=CARTESIAN_POINT ( 'NONE',  ( -0.05014649552828402690, 217.5146222423826714, 69.24886208192143044 ) ) ;
#6039=CARTESIAN_POINT ( 'NONE',  ( -9.736236675708031640, 214.0148392665760753, 2.798862081921433820 ) ) ;
#6041=CARTESIAN_POINT ( 'NONE',  ( 3.044812012440130555, 197.4746971517856764, 26.60113791807856742 ) ) ;
#6042=EDGE_CURVE ( 'NONE', #17930, #11179, #13495, .T. ) ;
#6043=CARTESIAN_POINT ( 'NONE',  ( 10.00000000000000711, 207.0476921513415220, 90.99886208192144466 ) ) ;
#6048=CARTESIAN_POINT ( 'NONE',  ( 6.500168698208244500, 202.3363017425938324, 58.29886208192143471 ) ) ;
#6056=CARTESIAN_POINT ( 'NONE',  ( -0.05014649552807731031, 198.5883022060938572, 68.75113791807856956 ) ) ;
#6057=FILL_AREA_STYLE ('',( #29407 ) ) ;
#6060=CARTESIAN_POINT ( 'NONE',  ( 4.903702542908435547, 213.8346818373419751, 45.54886208192144181 ) ) ;
#6061=CARTESIAN_POINT ( 'NONE',  ( 3.135527875058820690, 216.4958274776887492, 82.40113791807857524 ) ) ;
#6062=CARTESIAN_POINT ( 'NONE',  ( -3.044812012440131443, 216.5253028482142952, 70.10113791807857808 ) ) ;
#6064=CARTESIAN_POINT ( 'NONE',  ( -6.444103211791042618, 211.7408657792732356, 21.80113791807856671 ) ) ;
#6068=CARTESIAN_POINT ( 'NONE',  ( -7.375838497908182134, 217.2372850707499765, 45.95113791807857950 ) ) ;
#6070=CARTESIAN_POINT ( 'NONE',  ( -6.220909254589537696, 198.5229672870051161, 93.05113791807853829 ) ) ;
#6071=CARTESIAN_POINT ( 'NONE',  ( -8.062137200540920645, 212.9164362838581894, 69.80113791807856671 ) ) ;
#6072=CARTESIAN_POINT ( 'NONE',  ( -9.680171189290716072, 199.9079932115567146, 35.19886208192142618 ) ) ;
#6073=CARTESIAN_POINT ( 'NONE',  ( 6.139770520408223575, 215.5359834540460611, 39.54886208192143471 ) ) ;
#6075=CARTESIAN_POINT ( 'NONE',  ( 11.98450388067348271, 203.0532714938637753, 80.15113791807857524 ) ) ;
#6076=CARTESIAN_POINT ( 'NONE',  ( -4.903702542908602524, 213.8346818373418898, 96.95113791807857240 ) ) ;
#6077=CARTESIAN_POINT ( 'NONE',  ( -10.01549611932659722, 210.2015048109875011, 56.64886208192142902 ) ) ;
#6080=CARTESIAN_POINT ( 'NONE',  ( 12.01549611932659367, 203.1486557965466773, 58.14886208192143613 ) ) ;
#6083=CARTESIAN_POINT ( 'NONE',  ( -4.903702542908436435, 200.1653181626580249, 35.04886208192144181 ) ) ;
#6088=CARTESIAN_POINT ( 'NONE',  ( 8.000000000000008882, 206.9523078486586485, 47.00113791807856956 ) ) ;
#6090=CARTESIAN_POINT ( 'NONE',  ( -10.01549611932659722, 210.2015048109875011, 35.64886208192143613 ) ) ;
#6098=CARTESIAN_POINT ( 'NONE',  ( 4.984841277089891776, 200.2242689037093726, 13.44886208192143684 ) ) ;
#6099=CARTESIAN_POINT ( 'NONE',  ( 3.044812012440130555, 197.4746971517856764, 53.60113791807857098 ) ) ;
#6101=CARTESIAN_POINT ( 'NONE',  ( 8.062137200540920645, 201.0835637161417822, 41.30113791807857382 ) ) ;
#6104=CARTESIAN_POINT ( 'NONE',  ( 4.984841277089891776, 200.2242689037093726, 97.44886208192143329 ) ) ;
#6108=DIRECTION ( 'NONE',  ( -0.9891821073486152249, -0.1466927349985428231, 0.000000000000000000 ) ) ;
#6109=CARTESIAN_POINT ( 'NONE',  ( 7.456977232089302632, 217.1783343296989131, 16.55113791807857027 ) ) ;
#6113=CARTESIAN_POINT ( 'NONE',  ( 9.984503880673470277, 203.7031108863295401, 62.15113791807856813 ) ) ;
#6114=CARTESIAN_POINT ( 'NONE',  ( 3.044812012440130555, 197.4746971517856764, 38.60113791807857098 ) ) ;
#6117=CARTESIAN_POINT ( 'NONE',  ( -0.05014649552828442242, 219.6175466908591716, 3.248862081921433997 ) ) ;
#6118=CARTESIAN_POINT ( 'NONE',  ( -6.139770520408224463, 198.4640165459539105, 8.048862081921434708 ) ) ;
#6121=CARTESIAN_POINT ( 'NONE',  ( -0.05014649552807705357, 194.3824533091408000, 47.75113791807856245 ) ) ;
#6122=CARTESIAN_POINT ( 'NONE',  ( -6.500168698208129925, 202.3363017425936050, 72.20113791807857240 ) ) ;
#6124=CARTESIAN_POINT ( 'NONE',  ( -6.220909254589682469, 215.4770327129946850, 20.94886208192143684 ) ) ;
#6127=CARTESIAN_POINT ( 'NONE',  ( 8.062137200540920645, 201.0835637161417822, 80.30113791807858092 ) ) ;
#6135=CARTESIAN_POINT ( 'NONE',  ( -4.984841277089726574, 200.2242689037092305, 21.05113791807857027 ) ) ;
#6138=CARTESIAN_POINT ( 'NONE',  ( 10.00000000000000711, 207.0476921513415220, 6.998862081921434886 ) ) ;
#6146=CARTESIAN_POINT ( 'NONE',  ( 10.01549611932659545, 203.7984951890123853, 91.14886208192140771 ) ) ;
#6148=CARTESIAN_POINT ( 'NONE',  ( 3.135527875058820690, 216.4958274776887492, 19.40113791807856813 ) ) ;
#6150=CARTESIAN_POINT ( 'NONE',  ( -3.753561863808878130, 218.3979405102790281, 75.09886208192142476 ) ) ;
#6155=CARTESIAN_POINT ( 'NONE',  ( 8.118202686958039038, 212.8392687619912635, 91.70113791807857240 ) ) ;
#6158=CARTESIAN_POINT ( 'NONE',  ( 3.044812012440130555, 197.4746971517856764, 35.60113791807857098 ) ) ;
#6165=CARTESIAN_POINT ( 'NONE',  ( 12.00000000000000711, 206.9523078486586485, 23.00113791807856600 ) ) ;
#6172=CARTESIAN_POINT ( 'NONE',  ( -3.753561863808878130, 218.3979405102790281, 30.09886208192144252 ) ) ;
#6174=CARTESIAN_POINT ( 'NONE',  ( 6.139770520408368348, 198.4640165459539674, 53.45113791807855108 ) ) ;
#6176=CARTESIAN_POINT ( 'NONE',  ( -6.500168698208244500, 211.6636982574061676, 14.79886208192143471 ) ) ;
#6182=CARTESIAN_POINT ( 'NONE',  ( -4.903702542908436435, 200.1653181626580249, 98.04886208192144181 ) ) ;
#6183=CARTESIAN_POINT ( 'NONE',  ( 2.517493886308900919, 214.5937144450984420, 40.40113791807857524 ) ) ;
#6189=CARTESIAN_POINT ( 'NONE',  ( -10.00000000000000711, 206.9523078486584495, 62.49886208192143755 ) ) ;
#6193=CARTESIAN_POINT ( 'NONE',  ( -4.903702542908602524, 213.8346818373418898, 99.95113791807860082 ) ) ;
#6195=CARTESIAN_POINT ( 'NONE',  ( -4.984841277089891776, 213.7757310962905990, 74.94886208192143329 ) ) ;
#6199=CARTESIAN_POINT ( 'NONE',  ( 3.044812012440130555, 197.4746971517856764, 8.601137918078565647 ) ) ;
#6203=CARTESIAN_POINT ( 'NONE',  ( 9.680171189290831535, 199.9079932115568852, 74.30113791807858092 ) ) ;
#6205=CARTESIAN_POINT ( 'NONE',  ( 8.118202686958039038, 212.8392687619912635, 94.70113791807857240 ) ) ;
#6208=CARTESIAN_POINT ( 'NONE',  ( -6.139770520408224463, 198.4640165459539389, 5.048862081921435596 ) ) ;
#6209=CARTESIAN_POINT ( 'NONE',  ( -7.456977232089471386, 217.1783343296987709, 59.94886208192143329 ) ) ;
#6210=CARTESIAN_POINT ( 'NONE',  ( -3.135527875058982783, 216.4958274776886924, 66.09886208192143897 ) ) ;
#6212=CARTESIAN_POINT ( 'NONE',  ( 11.98450388067341876, 210.9467285061363953, 3.848862081921433642 ) ) ;
#6214=CARTESIAN_POINT ( 'NONE',  ( -10.00000000000000711, 207.0476921513413515, 27.50113791807856600 ) ) ;
#6216=CARTESIAN_POINT ( 'NONE',  ( -3.044812012439970683, 197.4746971517856196, 85.89886208192143613 ) ) ;
#6221=CARTESIAN_POINT ( 'NONE',  ( -6.444103211790928043, 202.2591342207265939, 71.19886208192144750 ) ) ;
#6228=CARTESIAN_POINT ( 'NONE',  ( 6.500168698208129925, 211.6636982574063381, 64.70113791807857240 ) ) ;
#6230=EDGE_CURVE ( 'NONE', #4391, #17930, #19504, .T. ) ;
#6231=CYLINDRICAL_SURFACE ( 'NONE', #12692, 3.000000000000002665 ) ;
#6233=CARTESIAN_POINT ( 'NONE',  ( -6.444103211790928043, 202.2591342207265939, 47.19886208192144750 ) ) ;
#6234=CARTESIAN_POINT ( 'NONE',  ( 3.135527875058820690, 216.4958274776887492, 85.40113791807857524 ) ) ;
#6237=CARTESIAN_POINT ( 'NONE',  ( 10.01549611932653860, 210.2015048109876716, 67.85113791807857808 ) ) ;
#6239=CARTESIAN_POINT ( 'NONE',  ( 4.984841277089725686, 213.7757310962907411, 22.55113791807857027 ) ) ;
#6243=CARTESIAN_POINT ( 'NONE',  ( -0.05014649552807705357, 194.3824533091408000, 47.75113791807856245 ) ) ;
#6246=CARTESIAN_POINT ( 'NONE',  ( -8.062137200540920645, 212.9164362838581894, 90.80113791807858092 ) ) ;
#6247=CARTESIAN_POINT ( 'NONE',  ( -8.062137200540920645, 212.9164362838581894, 72.80113791807856671 ) ) ;
#6248=CARTESIAN_POINT ( 'NONE',  ( 9.680171189290716072, 214.0920067884432854, 36.69886208192142618 ) ) ;
#6249=CARTESIAN_POINT ( 'NONE',  ( 0.05014649552828275014, 196.4853777576173002, 40.74886208192143044 ) ) ;
#6251=CARTESIAN_POINT ( 'NONE',  ( -9.736236675707914401, 199.9851607334237542, 78.20113791807857240 ) ) ;
#6252=CARTESIAN_POINT ( 'NONE',  ( -7.898309971686851227, 224.1054302408387287, 103.4854814124441447 ) ) ;
#6253=CARTESIAN_POINT ( 'NONE',  ( -6.139770520408224463, 198.4640165459539389, 59.04886208192143471 ) ) ;
#6256=CARTESIAN_POINT ( 'NONE',  ( -7.375838497908014268, 196.7627149292498530, 65.04886208192144181 ) ) ;
#6259=CARTESIAN_POINT ( 'NONE',  ( -6.500168698208244500, 211.6636982574061676, 41.79886208192144181 ) ) ;
#6264=CARTESIAN_POINT ( 'NONE',  ( 7.984503880673485376, 204.3529502787953902, 50.15113791807857524 ) ) ;
#6266=CARTESIAN_POINT ( 'NONE',  ( 10.01549611932659545, 203.7984951890123853, 31.14886208192142902 ) ) ;
#6272=CARTESIAN_POINT ( 'NONE',  ( -8.015496119326597224, 209.5516654185217362, 11.64886208192143613 ) ) ;
#6273=CARTESIAN_POINT ( 'NONE',  ( 10.00000000000000711, 206.9523078486586201, 50.00113791807856956 ) ) ;
#6275=CARTESIAN_POINT ( 'NONE',  ( -8.118202686958039038, 201.1607312380087080, 36.20113791807857240 ) ) ;
#6277=CARTESIAN_POINT ( 'NONE',  ( -2.426778023690076225, 199.3768101843759553, 100.8988620819214361 ) ) ;
#6281=CARTESIAN_POINT ( 'NONE',  ( 12.01549611932652972, 210.8513442034534933, 22.85113791807856742 ) ) ;
#6283=CARTESIAN_POINT ( 'NONE',  ( -9.984503880673473830, 210.2968891136704315, 69.65113791807854682 ) ) ;
#6284=CARTESIAN_POINT ( 'NONE',  ( 8.118202686958039038, 212.8392687619912635, 43.70113791807857240 ) ) ;
#6287=CARTESIAN_POINT ( 'NONE',  ( 0.05014649552828288198, 194.3824533091408000, 4.748862081921433109 ) ) ;
#6288=CARTESIAN_POINT ( 'NONE',  ( -10.00000000000000711, 206.9523078486584495, 8.498862081921433997 ) ) ;
#6291=CARTESIAN_POINT ( 'NONE',  ( -11.98450388067348804, 210.9467285061362247, 45.65113791807856813 ) ) ;
#6292=CARTESIAN_POINT ( 'NONE',  ( 6.444103211791042618, 202.2591342207267644, 71.30113791807856671 ) ) ;
#6294=CARTESIAN_POINT ( 'NONE',  ( 10.01549611932659545, 203.7984951890123853, 31.14886208192142902 ) ) ;
#6297=CARTESIAN_POINT ( 'NONE',  ( -8.062137200540920645, 212.9164362838581894, 78.80113791807858092 ) ) ;
#6299=B_SPLINE_CURVE_WITH_KNOTS ( 'NONE', 3,
 ( #1910, #22345, #6683, #32397, #14179, #9566 ),
 .UNSPECIFIED., .F., .F.,
 ( 4, 2, 4 ),
 ( -6.634491363447954936E-06, 0.0006892677013496626174, 0.001385169894062773148 ),
 .UNSPECIFIED. ) ;
#6303=CARTESIAN_POINT ( 'NONE',  ( 6.500168698208129925, 211.6636982574063381, 25.70113791807857240 ) ) ;
#6306=CARTESIAN_POINT ( 'NONE',  ( -8.062137200540822946, 201.0835637161416400, 8.198862081921435063 ) ) ;
#6310=CARTESIAN_POINT ( 'NONE',  ( -6.500168698208129925, 202.3363017425936050, 51.20113791807857240 ) ) ;
#6314=CARTESIAN_POINT ( 'NONE',  ( -10.01549611932659722, 210.2015048109875011, 86.64886208192139350 ) ) ;
#6316=CARTESIAN_POINT ( 'NONE',  ( -3.044812012440131443, 216.5253028482142952, 22.10113791807856742 ) ) ;
#6318=CARTESIAN_POINT ( 'NONE',  ( 7.456977232089471386, 196.8216656703012006, 82.44886208192144750 ) ) ;
#6324=CARTESIAN_POINT ( 'NONE',  ( -0.05014649552810635652, 196.4853777576173002, 92.75113791807858377 ) ) ;
#6327=CARTESIAN_POINT ( 'NONE',  ( 3.135527875058820690, 216.4958274776887492, 37.40113791807857524 ) ) ;
#6331=ORIENTED_EDGE ( 'NONE', *, *, #15102, .T. ) ;
#6335=CARTESIAN_POINT ( 'NONE',  ( 7.456977232089302632, 217.1783343296989131, 22.55113791807857027 ) ) ;
#6339=CARTESIAN_POINT ( 'NONE',  ( -3.662846001189865142, 195.5725841191952838, 37.89886208192143613 ) ) ;
#6341=CARTESIAN_POINT ( 'NONE',  ( -10.00000000000000711, 207.0476921513413515, 54.50113791807857666 ) ) ;
#6343=CARTESIAN_POINT ( 'NONE',  ( -2.517493886309087880, 214.5937144450984135, 18.09886208192143187 ) ) ;
#6349=CARTESIAN_POINT ( 'NONE',  ( 8.015496119326595448, 204.4483345814782638, 103.1488620819214361 ) ) ;
#6351=CARTESIAN_POINT ( 'NONE',  ( 8.015496119326531499, 209.5516654185219636, 43.85113791807856387 ) ) ;
#6356=CARTESIAN_POINT ( 'NONE',  ( 3.044812012439969795, 216.5253028482143520, 57.39886208192143613 ) ) ;
#6359=CARTESIAN_POINT ( 'NONE',  ( -8.015496119326531499, 204.4483345814780364, 96.35113791807857808 ) ) ;
#6362=CARTESIAN_POINT ( 'NONE',  ( 2.517493886309087436, 199.4062855549015865, 70.59886208192142476 ) ) ;
#6371=CARTESIAN_POINT ( 'NONE',  ( 10.00000000000000711, 206.9523078486586201, 17.00113791807856600 ) ) ;
#6375=CARTESIAN_POINT ( 'NONE',  ( -11.98450388067348804, 210.9467285061362247, 81.65113791807856103 ) ) ;
#6377=CARTESIAN_POINT ( 'NONE',  ( -8.118202686958039038, 201.1607312380087080, 96.20113791807857240 ) ) ;
#6382=CARTESIAN_POINT ( 'NONE',  ( -3.135527875058982783, 216.4958274776886924, 3.098862081921434974 ) ) ;
#6383=CARTESIAN_POINT ( 'NONE',  ( 11.98450388067341876, 210.9467285061363953, 60.84886208192143187 ) ) ;
#6384=CARTESIAN_POINT ( 'NONE',  ( 8.062137200540822946, 212.9164362838583315, 78.69886208192143329 ) ) ;
#6385=CARTESIAN_POINT ( 'NONE',  ( -7.375838497908014268, 196.7627149292498530, 2.048862081921434264 ) ) ;
#6387=CARTESIAN_POINT ( 'NONE',  ( 3.044812012440130555, 197.4746971517856764, 20.60113791807856742 ) ) ;
#6388=CARTESIAN_POINT ( 'NONE',  ( -8.118202686958138514, 212.8392687619910930, 92.79886208192144181 ) ) ;
#6394=CARTESIAN_POINT ( 'NONE',  ( -2.426778023690076225, 199.3768101843759553, 67.89886208192143613 ) ) ;
#6405=CARTESIAN_POINT ( 'NONE',  ( 4.903702542908601636, 200.1653181626581102, 71.45113791807854398 ) ) ;
#6410=CARTESIAN_POINT ( 'NONE',  ( -6.500168698208244500, 211.6636982574061676, 47.79886208192144181 ) ) ;
#6411=CARTESIAN_POINT ( 'NONE',  ( 3.044812012440130555, 197.4746971517856764, 89.60113791807857808 ) ) ;
#6412=CARTESIAN_POINT ( 'NONE',  ( -6.220909254589537696, 198.5229672870051161, 78.05113791807858092 ) ) ;
#6418=CARTESIAN_POINT ( 'NONE',  ( 12.00000000000000711, 206.9523078486586485, 47.00113791807856956 ) ) ;
#6422=CARTESIAN_POINT ( 'NONE',  ( 6.139770520408368348, 198.4640165459539674, 95.45113791807855819 ) ) ;
#6423=CARTESIAN_POINT ( 'NONE',  ( -6.139770520408368348, 215.5359834540460042, 72.95113791807855819 ) ) ;
#6425=CARTESIAN_POINT ( 'NONE',  ( 9.680171189290716072, 214.0920067884432854, 30.69886208192143684 ) ) ;
#6426=CARTESIAN_POINT ( 'NONE',  ( 0.05014649552828275014, 196.4853777576173002, 34.74886208192143044 ) ) ;
#6428=CARTESIAN_POINT ( 'NONE',  ( -12.00000000000000711, 207.0476921513413515, 75.50113791807856956 ) ) ;
#6429=CARTESIAN_POINT ( 'NONE',  ( 8.015496119326531499, 209.5516654185219636, 97.85113791807857808 ) ) ;
#6431=CARTESIAN_POINT ( 'NONE',  ( -0.05014649552828403384, 217.5146222423826714, 63.24886208192143755 ) ) ;
#6435=CARTESIAN_POINT ( 'NONE',  ( -3.753561863808878130, 218.3979405102790281, 63.09886208192143187 ) ) ;
#6436=VERTEX_POINT ( 'NONE', #10376 ) ;
#6438=CARTESIAN_POINT ( 'NONE',  ( 2.517493886309087436, 199.4062855549015865, 40.59886208192143897 ) ) ;
#6443=CARTESIAN_POINT ( 'NONE',  ( 10.00000000000000888, 207.0476921513417494, 0.9988620819214907298 ) ) ;
#6444=CARTESIAN_POINT ( 'NONE',  ( 8.000000000000008882, 206.9523078486586485, 53.00113791807857666 ) ) ;
#6448=CARTESIAN_POINT ( 'NONE',  ( 8.062137200540822946, 212.9164362838583315, 30.69886208192144039 ) ) ;
#6452=( NAMED_UNIT ( * ) PLANE_ANGLE_UNIT ( ) SI_UNIT ( $, .RADIAN. ) );
#6455=CARTESIAN_POINT ( 'NONE',  ( -6.444103211790928043, 202.2591342207265939, 14.19886208192143684 ) ) ;
#6456=CARTESIAN_POINT ( 'NONE',  ( -0.05014649552810635652, 196.4853777576173002, 59.75113791807857666 ) ) ;
#6457=CARTESIAN_POINT ( 'NONE',  ( -8.062137200540920645, 212.9164362838581894, 36.80113791807856671 ) ) ;
#6459=CARTESIAN_POINT ( 'NONE',  ( 8.000000000000008882, 207.0476921513415220, 99.99886208192143044 ) ) ;
#6463=CARTESIAN_POINT ( 'NONE',  ( -9.680171189290831535, 214.0920067884431148, 18.80113791807856671 ) ) ;
#6465=CARTESIAN_POINT ( 'NONE',  ( 3.135527875058820690, 216.4958274776887492, 70.40113791807857524 ) ) ;
#6466=CARTESIAN_POINT ( 'NONE',  ( -9.984503880673475606, 210.2968891136704315, 39.65113791807857524 ) ) ;
#6469=CARTESIAN_POINT ( 'NONE',  ( -11.89830997168683702, 232.6342992855866783, 103.4854814124441447 ) ) ;
#6470=CARTESIAN_POINT ( 'NONE',  ( -10.01549611932659545, 210.2015048109875011, 5.648862081921436129 ) ) ;
#6473=CARTESIAN_POINT ( 'NONE',  ( -7.456977232089304408, 196.8216656703010301, 51.05113791807856671 ) ) ;
#6474=CIRCLE ( 'NONE', #25509, 1.000000000000000000 ) ;
#6475=CARTESIAN_POINT ( 'NONE',  ( 4.984841277089725686, 213.7757310962907411, 70.55113791807856671 ) ) ;
#6478=CARTESIAN_POINT ( 'NONE',  ( 6.220909254589681581, 198.5229672870052582, 34.44886208192143329 ) ) ;
#6481=CARTESIAN_POINT ( 'NONE',  ( 3.044812012440130555, 197.4746971517856764, 86.60113791807857808 ) ) ;
#6489=CARTESIAN_POINT ( 'NONE',  ( 0.05014649552807626948, 215.4116977939061144, 25.25113791807856956 ) ) ;
#6491=CARTESIAN_POINT ( 'NONE',  ( -6.139770520408224463, 198.4640165459539389, 5.048862081921435596 ) ) ;
#6494=CARTESIAN_POINT ( 'NONE',  ( 7.984503880673485376, 204.3529502787953902, 50.15113791807857524 ) ) ;
#6495=CARTESIAN_POINT ( 'NONE',  ( -9.521242624480144912, 207.9188892840786878, 102.6634595774070533 ) ) ;
#6498=CARTESIAN_POINT ( 'NONE',  ( 0.05014649552828275708, 196.4853777576173002, 94.74886208192141623 ) ) ;
#6500=CARTESIAN_POINT ( 'NONE',  ( 9.984503880673470277, 203.7031108863295401, 32.15113791807857524 ) ) ;
#6502=CARTESIAN_POINT ( 'NONE',  ( -9.736236675708031640, 214.0148392665760753, 80.79886208192144181 ) ) ;
#6506=CARTESIAN_POINT ( 'NONE',  ( -3.135527875058821579, 197.5041725223112223, 98.90113791807857524 ) ) ;
#6509=CARTESIAN_POINT ( 'NONE',  ( -8.062137200540920645, 212.9164362838581894, 36.80113791807856671 ) ) ;
#6515=CARTESIAN_POINT ( 'NONE',  ( 0.05014649552807549926, 219.6175466908591716, 22.25113791807856956 ) ) ;
#6519=CARTESIAN_POINT ( 'NONE',  ( 3.662846001189864698, 218.4274158808046593, 42.39886208192144323 ) ) ;
#6520=CARTESIAN_POINT ( 'NONE',  ( 3.044812012440130555, 197.4746971517856764, 2.601137918078566091 ) ) ;
#6522=CARTESIAN_POINT ( 'NONE',  ( 6.220909254589536808, 215.4770327129947702, 49.55113791807855250 ) ) ;
#6524=CARTESIAN_POINT ( 'NONE',  ( 8.015496119326595448, 204.4483345814782638, 10.14886208192143435 ) ) ;
#6527=CARTESIAN_POINT ( 'NONE',  ( 6.500168698208244500, 202.3363017425938324, 100.2988620819214276 ) ) ;
#6529=CARTESIAN_POINT ( 'NONE',  ( -4.903702542908602524, 213.8346818373418898, 39.95113791807856529 ) ) ;
#6534=CARTESIAN_POINT ( 'NONE',  ( -8.062137200540822946, 201.0835637161416400, 65.19886208192143329 ) ) ;
#6537=CARTESIAN_POINT ( 'NONE',  ( -3.135527875058821579, 197.5041725223112223, 2.901137918078565914 ) ) ;
#6540=CARTESIAN_POINT ( 'NONE',  ( -0.05014649552828365914, 215.4116977939061144, 84.24886208192143044 ) ) ;
#6544=CARTESIAN_POINT ( 'NONE',  ( -6.139770520408368348, 215.5359834540460042, 15.95113791807856884 ) ) ;
#6548=CARTESIAN_POINT ( 'NONE',  ( -3.662846001190052991, 218.4274158808045740, 85.10113791807857808 ) ) ;
#6552=CARTESIAN_POINT ( 'NONE',  ( 9.680171189290716072, 214.0920067884432854, 66.69886208192143329 ) ) ;
#6553=CARTESIAN_POINT ( 'NONE',  ( 3.044812012439969795, 216.5253028482143520, 78.39886208192143613 ) ) ;
#6554=CARTESIAN_POINT ( 'NONE',  ( -9.680171189290716072, 199.9079932115567146, 17.19886208192143684 ) ) ;
#6556=CARTESIAN_POINT ( 'NONE',  ( -0.05014649552810635652, 196.4853777576173002, 23.75113791807855890 ) ) ;
#6557=CARTESIAN_POINT ( 'NONE',  ( -0.05014649552828403384, 217.5146222423826714, 93.24886208192140202 ) ) ;
#6562=CARTESIAN_POINT ( 'NONE',  ( 6.444103211790928043, 211.7408657792734061, 69.69886208192143329 ) ) ;
#6571=CARTESIAN_POINT ( 'NONE',  ( -4.903702542908602524, 213.8346818373418898, 72.95113791807857240 ) ) ;
#6576=CARTESIAN_POINT ( 'NONE',  ( 6.500168698208244500, 202.3363017425938324, 55.29886208192144892 ) ) ;
#6577=CARTESIAN_POINT ( 'NONE',  ( 6.220909254589536808, 215.4770327129947702, 73.55113791807858092 ) ) ;
#6582=CARTESIAN_POINT ( 'NONE',  ( 0.05014649552807549926, 219.6175466908591716, 55.25113791807857666 ) ) ;
#6584=CARTESIAN_POINT ( 'NONE',  ( 12.01549611932652972, 210.8513442034534933, 4.851137918078565647 ) ) ;
#6585=APPLICATION_CONTEXT ( 'automotive_design' ) ;
#6586=CARTESIAN_POINT ( 'NONE',  ( -9.984503880673475606, 210.2968891136704315, 78.65113791807856103 ) ) ;
#6587=CARTESIAN_POINT ( 'NONE',  ( -0.05014649552828442242, 219.6175466908591716, 36.24886208192142334 ) ) ;
#6588=CARTESIAN_POINT ( 'NONE',  ( 10.01549611932659367, 203.7984951890124421, 49.14886208192143613 ) ) ;
#6590=CARTESIAN_POINT ( 'NONE',  ( 7.456977232089302632, 217.1783343296989131, 88.55113791807858092 ) ) ;
#6591=CARTESIAN_POINT ( 'NONE',  ( 8.015496119326531499, 209.5516654185219636, 100.8511379180785781 ) ) ;
#6593=CARTESIAN_POINT ( 'NONE',  ( 10.00000000000000711, 207.0476921513415220, 57.99886208192143044 ) ) ;
#6596=CARTESIAN_POINT ( 'NONE',  ( -0.05014649552828442242, 219.6175466908591716, 57.24886208192144466 ) ) ;
#6600=CARTESIAN_POINT ( 'NONE',  ( -8.015496119326597224, 209.5516654185217362, 38.64886208192143613 ) ) ;
#6604=DIRECTION ( 'NONE',  ( 0.5526942671207055735, 0.1536855300543024383, 0.8190908404712107238 ) ) ;
#6605=CARTESIAN_POINT ( 'NONE',  ( 3.281878800801977025, 207.2857746820136526, -8.268545444955467616 ) ) ;
#6606=CARTESIAN_POINT ( 'NONE',  ( 6.444103211791042618, 202.2591342207267644, 59.30113791807857382 ) ) ;
#6608=CARTESIAN_POINT ( 'NONE',  ( 3.044812012439969795, 216.5253028482143520, 42.39886208192143613 ) ) ;
#6615=CARTESIAN_POINT ( 'NONE',  ( -4.903702542908436435, 200.1653181626580249, 11.04886208192143648 ) ) ;
#6616=CARTESIAN_POINT ( 'NONE',  ( 6.220909254589536808, 215.4770327129947702, 64.55113791807858092 ) ) ;
#6617=CARTESIAN_POINT ( 'NONE',  ( -8.062137200540920645, 212.9164362838581894, 42.80113791807857382 ) ) ;
#6620=CARTESIAN_POINT ( 'NONE',  ( -0.05014649552810635652, 196.4853777576173002, 20.75113791807855890 ) ) ;
#6622=CARTESIAN_POINT ( 'NONE',  ( -4.903702542908436435, 200.1653181626580249, 101.0488620819214276 ) ) ;
#6626=CARTESIAN_POINT ( 'NONE',  ( -9.680171189290831535, 214.0920067884431148, 27.80113791807857027 ) ) ;
#6629=CARTESIAN_POINT ( 'NONE',  ( 8.062137200540920645, 201.0835637161417822, 71.30113791807856671 ) ) ;
#6630=CARTESIAN_POINT ( 'NONE',  ( 8.062137200540920645, 201.0835637161417822, 35.30113791807857382 ) ) ;
#6633=CARTESIAN_POINT ( 'NONE',  ( 12.00000000000000711, 207.0476921513415220, 0.9988620819214339974 ) ) ;
#6634=CARTESIAN_POINT ( 'NONE',  ( -10.00000000000000711, 206.9523078486584495, 23.49886208192143755 ) ) ;
#6638=CARTESIAN_POINT ( 'NONE',  ( -7.375838497908182134, 217.2372850707499765, 48.95113791807855108 ) ) ;
#6639=CARTESIAN_POINT ( 'NONE',  ( 7.984503880673485376, 204.3529502787953902, 74.15113791807857524 ) ) ;
#6641=CARTESIAN_POINT ( 'NONE',  ( -10.01549611932659722, 210.2015048109875011, 32.64886208192143613 ) ) ;
#6644=CARTESIAN_POINT ( 'NONE',  ( -3.044812012440131443, 216.5253028482142952, 91.10113791807857808 ) ) ;
#6649=CARTESIAN_POINT ( 'NONE',  ( 7.984503880673485376, 204.3529502787953902, 26.15113791807857169 ) ) ;
#6651=CARTESIAN_POINT ( 'NONE',  ( -6.139770520408224463, 198.4640165459539389, 8.048862081921434708 ) ) ;
#6654=CARTESIAN_POINT ( 'NONE',  ( 4.903702542908601636, 200.1653181626581102, 53.45113791807857950 ) ) ;
#6658=CARTESIAN_POINT ( 'NONE',  ( 10.00000000000000711, 207.0476921513415220, 90.99886208192144466 ) ) ;
#6661=CARTESIAN_POINT ( 'NONE',  ( -3.044812012440131443, 216.5253028482142952, 31.10113791807856742 ) ) ;
#6665=CARTESIAN_POINT ( 'NONE',  ( 6.220909254589536808, 215.4770327129947702, 19.55113791807856671 ) ) ;
#6670=CARTESIAN_POINT ( 'NONE',  ( -6.139770520408369237, 215.5359834540460042, 96.95113791807857240 ) ) ;
#6674=CARTESIAN_POINT ( 'NONE',  ( -0.05014649552810635652, 196.4853777576173002, 38.75113791807856956 ) ) ;
#6681=CARTESIAN_POINT ( 'NONE',  ( 9.680171189290831535, 199.9079932115568852, 20.30113791807857027 ) ) ;
#6683=CARTESIAN_POINT ( 'NONE',  ( -10.95989699996054512, 207.3450541041420081, 103.1859396839448806 ) ) ;
#6687=CARTESIAN_POINT ( 'NONE',  ( -0.05014649552828442242, 219.6175466908591716, 39.24886208192143755 ) ) ;
#6688=CARTESIAN_POINT ( 'NONE',  ( -9.984503880673473830, 210.2968891136704315, 3.651137918078565026 ) ) ;
#6689=CARTESIAN_POINT ( 'NONE',  ( -0.05014649552810635652, 196.4853777576173002, 62.75113791807856956 ) ) ;
#6691=CARTESIAN_POINT ( 'NONE',  ( -2.517493886309087880, 214.5937144450984135, 24.09886208192143897 ) ) ;
#6694=VERTEX_POINT ( 'NONE', #4530 ) ;
#6695=CARTESIAN_POINT ( 'NONE',  ( -6.500168698208244500, 211.6636982574061676, 101.7988620819214560 ) ) ;
#6697=CARTESIAN_POINT ( 'NONE',  ( -8.000000000000008882, 207.0476921513413515, 39.50113791807857666 ) ) ;
#6702=CARTESIAN_POINT ( 'NONE',  ( 6.220909254589536808, 215.4770327129947702, 1.551137918078565825 ) ) ;
#6704=CARTESIAN_POINT ( 'NONE',  ( 6.139770520408223575, 215.5359834540460611, 66.54886208192144181 ) ) ;
#6706=LINE ( 'NONE', #9588, #16735 ) ;
#6707=CARTESIAN_POINT ( 'NONE',  ( 3.044812012440130555, 197.4746971517856764, 5.601137918078566535 ) ) ;
#6711=CARTESIAN_POINT ( 'NONE',  ( 7.984503880673422316, 209.6470497212048372, 78.84886208192143897 ) ) ;
#6717=CARTESIAN_POINT ( 'NONE',  ( 10.01549611932653860, 210.2015048109876716, 22.85113791807856742 ) ) ;
#6721=CARTESIAN_POINT ( 'NONE',  ( 12.01549611932652972, 210.8513442034534933, 88.85113791807857808 ) ) ;
#6724=CARTESIAN_POINT ( 'NONE',  ( 3.662846001189864698, 218.4274158808046593, 72.39886208192143613 ) ) ;
#6726=CARTESIAN_POINT ( 'NONE',  ( 3.135527875058981895, 197.5041725223112792, 76.59886208192142476 ) ) ;
#6727=CARTESIAN_POINT ( 'NONE',  ( -0.05014649552828442242, 219.6175466908591716, 12.24886208192143577 ) ) ;
#6729=CARTESIAN_POINT ( 'NONE',  ( 6.139770520408368348, 198.4640165459539674, 29.45113791807856529 ) ) ;
#6731=CARTESIAN_POINT ( 'NONE',  ( 8.118202686958138514, 201.1607312380088501, 85.29886208192144181 ) ) ;
#6735=CARTESIAN_POINT ( 'NONE',  ( -2.517493886309087880, 214.5937144450984135, 69.09886208192143897 ) ) ;
#6743=CARTESIAN_POINT ( 'NONE',  ( 4.984841277089725686, 213.7757310962907411, 79.55113791807858092 ) ) ;
#6747=CARTESIAN_POINT ( 'NONE',  ( 2.426778023690075337, 214.6231898156240447, 54.39886208192144323 ) ) ;
#6755=CARTESIAN_POINT ( 'NONE',  ( -3.753561863808691168, 195.6020594897209435, 59.90113791807856103 ) ) ;
#6758=CARTESIAN_POINT ( 'NONE',  ( 11.98450388067348271, 203.0532714938637753, 5.151137918078566358 ) ) ;
#6760=CARTESIAN_POINT ( 'NONE',  ( 9.984503880673473830, 203.7031108863295401, 80.15113791807858945 ) ) ;
#6761=CARTESIAN_POINT ( 'NONE',  ( 3.662846001189864698, 218.4274158808046593, 39.39886208192143613 ) ) ;
#6762=CARTESIAN_POINT ( 'NONE',  ( 3.135527875058981895, 197.5041725223112792, 52.59886208192143897 ) ) ;
#6764=CARTESIAN_POINT ( 'NONE',  ( 9.680171189290831535, 199.9079932115568852, 83.30113791807858092 ) ) ;
#6765=CARTESIAN_POINT ( 'NONE',  ( 4.903702542908601636, 200.1653181626581102, 95.45113791807858661 ) ) ;
#6766=CARTESIAN_POINT ( 'NONE',  ( 10.00000000000000711, 207.0476921513415220, 60.99886208192143755 ) ) ;
#6769=CARTESIAN_POINT ( 'NONE',  ( -3.662846001189865142, 195.5725841191952838, 70.89886208192143613 ) ) ;
#6773=CARTESIAN_POINT ( 'NONE',  ( -2.426778023690076225, 199.3768101843759553, 43.89886208192144323 ) ) ;
#6778=CARTESIAN_POINT ( 'NONE',  ( -0.05014649552807731031, 198.5883022060938572, 62.75113791807856245 ) ) ;
#6780=CARTESIAN_POINT ( 'NONE',  ( -10.01549611932659722, 210.2015048109875011, 41.64886208192144323 ) ) ;
#6785=CARTESIAN_POINT ( 'NONE',  ( -0.05014649552828365914, 215.4116977939061144, 24.24886208192144110 ) ) ;
#6786=CARTESIAN_POINT ( 'NONE',  ( 10.00000000000000711, 206.9523078486586201, 65.00113791807856956 ) ) ;
#6787=CARTESIAN_POINT ( 'NONE',  ( 0.05014649552810505201, 217.5146222423826714, 49.25113791807857666 ) ) ;
#6789=CARTESIAN_POINT ( 'NONE',  ( -10.00000000000000711, 207.0476921513413515, 15.50113791807856600 ) ) ;
#6790=CARTESIAN_POINT ( 'NONE',  ( -8.000000000000008882, 207.0476921513413515, 3.501137918078566003 ) ) ;
#6794=CARTESIAN_POINT ( 'NONE',  ( -9.680171189290831535, 214.0920067884431148, 30.80113791807857027 ) ) ;
#6796=CARTESIAN_POINT ( 'NONE',  ( -8.118202686958039038, 201.1607312380087080, 72.20113791807857240 ) ) ;
#6798=CARTESIAN_POINT ( 'NONE',  ( 10.01549611932653860, 210.2015048109876716, 46.85113791807856387 ) ) ;
#6801=CARTESIAN_POINT ( 'NONE',  ( 12.00000000000000711, 207.0476921513415220, 12.99886208192143400 ) ) ;
#6802=CARTESIAN_POINT ( 'NONE',  ( -0.05014649552828402690, 217.5146222423826714, 18.24886208192143755 ) ) ;
#6805=CARTESIAN_POINT ( 'NONE',  ( -12.00000000000000711, 207.0476921513413515, 60.50113791807856956 ) ) ;
#6807=CARTESIAN_POINT ( 'NONE',  ( 6.444103211791042618, 202.2591342207267644, 68.30113791807856671 ) ) ;
#6808=CARTESIAN_POINT ( 'NONE',  ( -8.118202686958138514, 212.8392687619910930, 35.79886208192143471 ) ) ;
#6812=CARTESIAN_POINT ( 'NONE',  ( -6.139770520408369237, 215.5359834540460042, 87.95113791807858661 ) ) ;
#6817=CARTESIAN_POINT ( 'NONE',  ( 4.984841277089725686, 213.7757310962907411, 28.55113791807857027 ) ) ;
#6821=CARTESIAN_POINT ( 'NONE',  ( -3.044812012439970683, 197.4746971517856196, 10.89886208192143613 ) ) ;
#6824=CARTESIAN_POINT ( 'NONE',  ( 6.444103211791042618, 202.2591342207267644, 50.30113791807858092 ) ) ;
#6827=CARTESIAN_POINT ( 'NONE',  ( 8.118202686958138514, 201.1607312380088501, 103.2988620819214418 ) ) ;
#6830=CARTESIAN_POINT ( 'NONE',  ( -9.984503880673473830, 210.2968891136704315, 30.65113791807856813 ) ) ;
#6832=CARTESIAN_POINT ( 'NONE',  ( -6.139770520408369237, 215.5359834540460042, 18.95113791807856884 ) ) ;
#6837=CARTESIAN_POINT ( 'NONE',  ( 11.98450388067348271, 203.0532714938637753, 5.151137918078566358 ) ) ;
#6840=CARTESIAN_POINT ( 'NONE',  ( -6.139770520408369237, 215.5359834540460042, 45.95113791807857950 ) ) ;
#6846=CARTESIAN_POINT ( 'NONE',  ( 11.98450388067348271, 203.0532714938637753, 29.15113791807857169 ) ) ;
#6850=CARTESIAN_POINT ( 'NONE',  ( -12.01549611932659722, 210.8513442034533227, 44.64886208192143613 ) ) ;
#6851=CARTESIAN_POINT ( 'NONE',  ( -0.05014649552810635652, 196.4853777576173002, -0.2488620819214343305 ) ) ;
#6852=CARTESIAN_POINT ( 'NONE',  ( -10.01549611932653860, 203.7984951890123284, 63.35113791807857098 ) ) ;
#6853=CARTESIAN_POINT ( 'NONE',  ( -7.984503880673422316, 204.3529502787951628, 23.34886208192143542 ) ) ;
#6857=CARTESIAN_POINT ( 'NONE',  ( -2.517493886308901807, 199.4062855549015012, 2.901137918078565914 ) ) ;
#6861=CARTESIAN_POINT ( 'NONE',  ( -3.662846001189865142, 195.5725841191952838, 88.89886208192143613 ) ) ;
#6866=FACE_OUTER_BOUND ( 'NONE', #28324, .T. ) ;
#6867=CARTESIAN_POINT ( 'NONE',  ( 9.984503880673420539, 210.2968891136705167, 57.84886208192143897 ) ) ;
#6871=CARTESIAN_POINT ( 'NONE',  ( 3.044812012440130555, 197.4746971517856764, -0.3988620819214342972 ) ) ;
#6875=CARTESIAN_POINT ( 'NONE',  ( -4.903702542908436435, 200.1653181626580249, 80.04886208192144181 ) ) ;
#6877=DIRECTION ( 'NONE',  ( 0.000000000000000000, 0.9988620819214357738, 0.04769215134144196705 ) ) ;
#6878=CARTESIAN_POINT ( 'NONE',  ( -0.05014649552828442242, 219.6175466908591716, 84.24886208192143044 ) ) ;
#6880=CARTESIAN_POINT ( 'NONE',  ( 0.05014649552810506589, 217.5146222423826714, 19.25113791807856600 ) ) ;
#6884=CARTESIAN_POINT ( 'NONE',  ( 7.375838497908181246, 196.7627149292499666, 83.45113791807857240 ) ) ;
#6888=CARTESIAN_POINT ( 'NONE',  ( -9.736236675708031640, 214.0148392665760753, 71.79886208192142760 ) ) ;
#6890=CARTESIAN_POINT ( 'NONE',  ( -6.139770520408224463, 198.4640165459539105, 77.04886208192144181 ) ) ;
#6891=CARTESIAN_POINT ( 'NONE',  ( 7.456977232089471386, 196.8216656703012006, 13.44886208192143684 ) ) ;
#6893=CARTESIAN_POINT ( 'NONE',  ( -6.220909254589537696, 198.5229672870051161, 33.05113791807857382 ) ) ;
#6894=DIRECTION ( 'NONE',  ( 0.5526942671207023539, 0.1536855300543050473, 0.8190908404712123891 ) ) ;
#6895=CARTESIAN_POINT ( 'NONE',  ( 8.062137200540822946, 212.9164362838583315, 96.69886208192143329 ) ) ;
#6900=CARTESIAN_POINT ( 'NONE',  ( -4.903702542908436435, 200.1653181626580249, 71.04886208192142760 ) ) ;
#6910=CARTESIAN_POINT ( 'NONE',  ( 4.903702542908601636, 200.1653181626581102, 74.45113791807855819 ) ) ;
#6915=CARTESIAN_POINT ( 'NONE',  ( 8.015496119326595448, 204.4483345814782638, 52.14886208192145034 ) ) ;
#6922=CARTESIAN_POINT ( 'NONE',  ( 9.736236675707914401, 214.0148392665762458, 58.70113791807857240 ) ) ;
#6924=CARTESIAN_POINT ( 'NONE',  ( -7.375838497908182134, 217.2372850707499765, 0.9511379180785655141 ) ) ;
#6925=CARTESIAN_POINT ( 'NONE',  ( -6.139770520408368348, 215.5359834540460042, 81.95113791807855819 ) ) ;
#6926=CARTESIAN_POINT ( 'NONE',  ( -0.05014649552828442242, 219.6175466908591716, 45.24886208192143755 ) ) ;
#6927=CARTESIAN_POINT ( 'NONE',  ( -9.984503880673420539, 203.7031108863293980, 50.34886208192143187 ) ) ;
#6929=CARTESIAN_POINT ( 'NONE',  ( 12.00000000000000711, 206.9523078486586485, 83.00113791807856956 ) ) ;
#6932=CARTESIAN_POINT ( 'NONE',  ( -6.220909254589537696, 198.5229672870051161, 6.051137918078566713 ) ) ;
#6933=CARTESIAN_POINT ( 'NONE',  ( 10.01549611932659545, 203.7984951890123853, 73.14886208192143613 ) ) ;
#6937=CARTESIAN_POINT ( 'NONE',  ( -9.680171189290716072, 199.9079932115567146, 74.19886208192143329 ) ) ;
#6942=CARTESIAN_POINT ( 'NONE',  ( 2.426778023690075337, 214.6231898156240447, 42.39886208192144323 ) ) ;
#6950=CARTESIAN_POINT ( 'NONE',  ( -3.044812012439970683, 197.4746971517856196, 40.89886208192143613 ) ) ;
#6956=CARTESIAN_POINT ( 'NONE',  ( 7.984503880673422316, 209.6470497212048372, 27.84886208192143897 ) ) ;
#6958=CARTESIAN_POINT ( 'NONE',  ( -6.220909254589537696, 198.5229672870051161, 57.05113791807857382 ) ) ;
#6960=CARTESIAN_POINT ( 'NONE',  ( 10.00000000000000711, 206.9523078486586201, 47.00113791807856956 ) ) ;
#6964=CARTESIAN_POINT ( 'NONE',  ( 6.139770520408368348, 198.4640165459539674, 17.45113791807855819 ) ) ;
#6965=CARTESIAN_POINT ( 'NONE',  ( -4.984841277089726574, 200.2242689037092305, 3.051137918078566269 ) ) ;
#6969=CARTESIAN_POINT ( 'NONE',  ( 12.01549611932652972, 210.8513442034534933, 31.85113791807857453 ) ) ;
#6971=CARTESIAN_POINT ( 'NONE',  ( 6.220909254589536808, 215.4770327129947702, 79.55113791807855250 ) ) ;
#6972=CARTESIAN_POINT ( 'NONE',  ( 0.05014649552810506589, 217.5146222423826714, 49.25113791807856956 ) ) ;
#6976=CARTESIAN_POINT ( 'NONE',  ( -0.05014649552828442242, 219.6175466908591716, 12.24886208192143577 ) ) ;
#6977=CARTESIAN_POINT ( 'NONE',  ( -3.135527875058982783, 216.4958274776886924, 18.09886208192143542 ) ) ;
#6980=CARTESIAN_POINT ( 'NONE',  ( -12.00000000000000711, 207.0476921513413515, 57.50113791807856956 ) ) ;
#6981=CARTESIAN_POINT ( 'NONE',  ( 2.426778023690261410, 199.3768101843759837, 83.60113791807857808 ) ) ;
#6982=CARTESIAN_POINT ( 'NONE',  ( -10.00000000000000711, 206.9523078486584495, 32.49886208192143044 ) ) ;
#6992=CARTESIAN_POINT ( 'NONE',  ( -2.517493886308901807, 199.4062855549015012, 29.90113791807857169 ) ) ;
#6995=CARTESIAN_POINT ( 'NONE',  ( -3.135527875058982783, 216.4958274776886924, 18.09886208192143542 ) ) ;
#6999=CARTESIAN_POINT ( 'NONE',  ( 2.517493886308900919, 214.5937144450984420, 52.40113791807858235 ) ) ;
#7002=CARTESIAN_POINT ( 'NONE',  ( 8.118202686958138514, 201.1607312380088501, 100.2988620819214418 ) ) ;
#7004=CARTESIAN_POINT ( 'NONE',  ( 6.220909254589536808, 215.4770327129947702, 31.55113791807857382 ) ) ;
#7005=CARTESIAN_POINT ( 'NONE',  ( 3.044812012440130555, 197.4746971517856764, 20.60113791807856742 ) ) ;
#7010=CARTESIAN_POINT ( 'NONE',  ( 0.05014649552810505201, 217.5146222423826714, 100.2511379180785838 ) ) ;
#7013=CARTESIAN_POINT ( 'NONE',  ( 8.118202686958039038, 212.8392687619912635, 49.70113791807857240 ) ) ;
#7021=CARTESIAN_POINT ( 'NONE',  ( 12.01549611932652972, 210.8513442034534933, 31.85113791807857453 ) ) ;
#7023=CARTESIAN_POINT ( 'NONE',  ( -9.680171189290716072, 199.9079932115567146, 104.1988620819214475 ) ) ;
#7027=CARTESIAN_POINT ( 'NONE',  ( 10.00000000000000711, 206.9523078486586201, 5.001137918078565114 ) ) ;
#7028=CARTESIAN_POINT ( 'NONE',  ( 6.139770520408368348, 198.4640165459539674, 65.45113791807857240 ) ) ;
#7029=EDGE_CURVE ( 'NONE', #20137, #14046, #6474, .T. ) ;
#7030=CARTESIAN_POINT ( 'NONE',  ( -6.500168698208244500, 211.6636982574061676, 26.79886208192143826 ) ) ;
#7033=CARTESIAN_POINT ( 'NONE',  ( 7.984503880673485376, 204.3529502787953902, -0.8488620819214343083 ) ) ;
#7037=CARTESIAN_POINT ( 'NONE',  ( -0.05014649552828442242, 219.6175466908591716, 87.24886208192144466 ) ) ;
#7043=CARTESIAN_POINT ( 'NONE',  ( -6.220909254589682469, 215.4770327129946850, 71.94886208192144750 ) ) ;
#7046=CARTESIAN_POINT ( 'NONE',  ( 8.118202686958039038, 212.8392687619912635, 7.701137918078566180 ) ) ;
#7051=CARTESIAN_POINT ( 'NONE',  ( 3.135527875058820690, 216.4958274776887492, 91.40113791807857524 ) ) ;
#7055=CARTESIAN_POINT ( 'NONE',  ( 3.753561863808876797, 195.6020594897209719, 88.59886208192143897 ) ) ;
#7057=CARTESIAN_POINT ( 'NONE',  ( 8.062137200540920645, 201.0835637161417822, 23.30113791807856671 ) ) ;
#7061=CARTESIAN_POINT ( 'NONE',  ( 3.662846001190051659, 195.5725841191953691, 86.60113791807857808 ) ) ;
#7066=CARTESIAN_POINT ( 'NONE',  ( 7.456977232089471386, 196.8216656703012006, 73.44886208192143329 ) ) ;
#7067=CARTESIAN_POINT ( 'NONE',  ( 10.01549611932659367, 203.7984951890124421, 73.14886208192143613 ) ) ;
#7068=CARTESIAN_POINT ( 'NONE',  ( 12.01549611932659367, 203.1486557965466773, 10.14886208192143435 ) ) ;
#7070=CARTESIAN_POINT ( 'NONE',  ( 8.118202686958039038, 212.8392687619912635, 34.70113791807857240 ) ) ;
#7073=CARTESIAN_POINT ( 'NONE',  ( -6.139770520408224463, 198.4640165459539389, 101.0488620819214134 ) ) ;
#7077=CARTESIAN_POINT ( 'NONE',  ( 2.426778023690075337, 214.6231898156240447, 81.39886208192143613 ) ) ;
#7084=CARTESIAN_POINT ( 'NONE',  ( -2.517493886308901807, 199.4062855549015012, 77.90113791807856103 ) ) ;
#7088=CARTESIAN_POINT ( 'NONE',  ( 6.500168698208244500, 202.3363017425938324, 58.29886208192143471 ) ) ;
#7096=CARTESIAN_POINT ( 'NONE',  ( -12.01549611932652972, 203.1486557965464499, 54.35113791807857098 ) ) ;
#7098=CARTESIAN_POINT ( 'NONE',  ( -10.01549611932653860, 203.7984951890123284, 102.3511379180785781 ) ) ;
#7100=CARTESIAN_POINT ( 'NONE',  ( 8.062137200540920645, 201.0835637161417822, 80.30113791807858092 ) ) ;
#7101=CARTESIAN_POINT ( 'NONE',  ( 12.00000000000000711, 207.0476921513415220, 45.99886208192143755 ) ) ;
#7102=CARTESIAN_POINT ( 'NONE',  ( -10.01549611932659545, 210.2015048109875011, 44.64886208192142902 ) ) ;
#7104=CARTESIAN_POINT ( 'NONE',  ( 7.375838497908181246, 196.7627149292499666, 83.45113791807857240 ) ) ;
#7106=CARTESIAN_POINT ( 'NONE',  ( 9.984503880673470277, 203.7031108863295401, -0.8488620819214341973 ) ) ;
#7108=CARTESIAN_POINT ( 'NONE',  ( -3.135527875058982783, 216.4958274776886924, 69.09886208192143897 ) ) ;
#7111=CARTESIAN_POINT ( 'NONE',  ( 11.98450388067341876, 210.9467285061363953, 75.84886208192143897 ) ) ;
#7114=CARTESIAN_POINT ( 'NONE',  ( -7.984503880673422316, 204.3529502787951628, 56.34886208192144608 ) ) ;
#7121=CARTESIAN_POINT ( 'NONE',  ( 10.00000000000000711, 207.0476921513415220, 45.99886208192143755 ) ) ;
#7127=CARTESIAN_POINT ( 'NONE',  ( 6.444103211790928043, 211.7408657792734061, 27.69886208192143684 ) ) ;
#7128=CARTESIAN_POINT ( 'NONE',  ( 3.135527875058820690, 216.4958274776887492, 70.40113791807857524 ) ) ;
#7130=CARTESIAN_POINT ( 'NONE',  ( 10.01549611932653860, 210.2015048109876716, 49.85113791807857808 ) ) ;
#7132=CARTESIAN_POINT ( 'NONE',  ( 8.062137200540920645, 201.0835637161417822, 17.30113791807856671 ) ) ;
#7133=CARTESIAN_POINT ( 'NONE',  ( -7.984503880673488041, 209.6470497212046098, 6.651137918078566358 ) ) ;
#7137=CARTESIAN_POINT ( 'NONE',  ( 7.375838497908181246, 196.7627149292499666, 29.45113791807856529 ) ) ;
#7139=CARTESIAN_POINT ( 'NONE',  ( 9.984503880673470277, 203.7031108863295401, 80.15113791807858945 ) ) ;
#7140=CARTESIAN_POINT ( 'NONE',  ( -6.139770520408368348, 215.5359834540460042, 45.95113791807857950 ) ) ;
#7143=CARTESIAN_POINT ( 'NONE',  ( -12.00000000000000711, 206.9523078486584780, 11.49886208192143577 ) ) ;
#7144=CARTESIAN_POINT ( 'NONE',  ( -6.139770520408224463, 198.4640165459539105, 20.04886208192143116 ) ) ;
#7148=CARTESIAN_POINT ( 'NONE',  ( -3.662846001190052991, 218.4274158808045740, 61.10113791807857808 ) ) ;
#7149=CARTESIAN_POINT ( 'NONE',  ( -6.444103211791042618, 211.7408657792732356, 75.80113791807858092 ) ) ;
#7150=CARTESIAN_POINT ( 'NONE',  ( -8.118202686958138514, 212.8392687619910930, 44.79886208192143471 ) ) ;
#7158=CARTESIAN_POINT ( 'NONE',  ( -2.517493886308901807, 199.4062855549015012, 32.90113791807857524 ) ) ;
#7161=CARTESIAN_POINT ( 'NONE',  ( 8.118202686958138514, 201.1607312380088501, 13.29886208192143648 ) ) ;
#7164=CARTESIAN_POINT ( 'NONE',  ( 4.984841277089725686, 213.7757310962907411, 55.55113791807858092 ) ) ;
#7169=CARTESIAN_POINT ( 'NONE',  ( 0.05014649552828275708, 196.4853777576173002, 103.7488620819214589 ) ) ;
#7171=CARTESIAN_POINT ( 'NONE',  ( 8.062137200540920645, 201.0835637161417822, 35.30113791807857382 ) ) ;
#7172=CARTESIAN_POINT ( 'NONE',  ( -4.927659837809095222, 206.3103720916592465, -5.504302862921502282 ) ) ;
#7173=CARTESIAN_POINT ( 'NONE',  ( 3.135527875058820690, 216.4958274776887492, 13.40113791807856636 ) ) ;
#7179=CARTESIAN_POINT ( 'NONE',  ( -3.662846001190052991, 218.4274158808045740, 4.101137918078565647 ) ) ;
#7182=CARTESIAN_POINT ( 'NONE',  ( 3.044812012440130555, 197.4746971517856764, 44.60113791807857098 ) ) ;
#7188=CARTESIAN_POINT ( 'NONE',  ( 9.736236675707914401, 214.0148392665762458, 25.70113791807857240 ) ) ;
#7191=CARTESIAN_POINT ( 'NONE',  ( -3.044812012439970683, 197.4746971517856196, 13.89886208192143613 ) ) ;
#7194=CARTESIAN_POINT ( 'NONE',  ( 10.00000000000000711, 206.9523078486586201, -0.9988620819214343305 ) ) ;
#7195=CARTESIAN_POINT ( 'NONE',  ( -3.044812012440131443, 216.5253028482142952, 61.10113791807857098 ) ) ;
#7197=CARTESIAN_POINT ( 'NONE',  ( -7.984503880673422316, 204.3529502787951628, 20.34886208192143542 ) ) ;
#7201=CARTESIAN_POINT ( 'NONE',  ( -4.903702542908602524, 213.8346818373418898, 3.951137918078566624 ) ) ;
#7203=CARTESIAN_POINT ( 'NONE',  ( 0.05014649552828288198, 194.3824533091408000, 91.74886208192144466 ) ) ;
#7208=CARTESIAN_POINT ( 'NONE',  ( 9.984503880673470277, 203.7031108863295401, 2.151137918078565914 ) ) ;
#7209=CARTESIAN_POINT ( 'NONE',  ( -6.139770520408224463, 198.4640165459539389, 74.04886208192142760 ) ) ;
#7212=CARTESIAN_POINT ( 'NONE',  ( -8.062137200540920645, 212.9164362838581894, 0.8011379180785658249 ) ) ;
#7216=CARTESIAN_POINT ( 'NONE',  ( -6.139770520408369237, 215.5359834540460042, 93.95113791807854398 ) ) ;
#7218=CARTESIAN_POINT ( 'NONE',  ( 0.05014649552810505201, 217.5146222423826714, 79.25113791807856956 ) ) ;
#7221=CARTESIAN_POINT ( 'NONE',  ( 9.680171189290716072, 214.0920067884432854, 87.69886208192144750 ) ) ;
#7223=CARTESIAN_POINT ( 'NONE',  ( -6.139770520408368348, 215.5359834540460042, 33.95113791807856529 ) ) ;
#7228=CARTESIAN_POINT ( 'NONE',  ( 9.680171189290831535, 199.9079932115568852, 92.30113791807858092 ) ) ;
#7233=CARTESIAN_POINT ( 'NONE',  ( -0.05014649552828402690, 217.5146222423826714, 90.24886208192143044 ) ) ;
#7234=CARTESIAN_POINT ( 'NONE',  ( 0.05014649552828288198, 194.3824533091408000, 13.74886208192143577 ) ) ;
#7236=CARTESIAN_POINT ( 'NONE',  ( -0.05014649552810635652, 196.4853777576173002, 32.75113791807856956 ) ) ;
#7238=CARTESIAN_POINT ( 'NONE',  ( -8.062137200540822946, 201.0835637161416400, 98.19886208192143329 ) ) ;
#7243=CARTESIAN_POINT ( 'NONE',  ( -9.981832587775443244, 205.9534224131111273, 104.4516590477787901 ) ) ;
#7244=CARTESIAN_POINT ( 'NONE',  ( 4.984841277089891776, 200.2242689037093726, 79.44886208192144750 ) ) ;
#7256=CARTESIAN_POINT ( 'NONE',  ( -0.05014649552807731031, 198.5883022060938572, 74.75113791807856956 ) ) ;
#7260=CARTESIAN_POINT ( 'NONE',  ( 4.984841277089891776, 200.2242689037093726, 58.44886208192144039 ) ) ;
#7269=CARTESIAN_POINT ( 'NONE',  ( -7.456977232089304408, 196.8216656703010301, 60.05113791807858092 ) ) ;
#7271=CARTESIAN_POINT ( 'NONE',  ( -3.662846001190052991, 218.4274158808045740, 4.101137918078565647 ) ) ;
#7272=CARTESIAN_POINT ( 'NONE',  ( 8.118202686958039038, 212.8392687619912635, 76.70113791807857240 ) ) ;
#7273=CARTESIAN_POINT ( 'NONE',  ( 11.98450388067341876, 210.9467285061363953, 45.84886208192143187 ) ) ;
#7274=CARTESIAN_POINT ( 'NONE',  ( 10.01549611932659367, 203.7984951890124421, 58.14886208192142902 ) ) ;
#7278=CARTESIAN_POINT ( 'NONE',  ( -9.736236675707914401, 199.9851607334237542, 84.20113791807858661 ) ) ;
#7280=CARTESIAN_POINT ( 'NONE',  ( 10.00000000000000711, 206.9523078486586201, 8.001137918078566003 ) ) ;
#7282=CARTESIAN_POINT ( 'NONE',  ( -9.984503880673420539, 203.7031108863293980, 65.34886208192143897 ) ) ;
#7286=CARTESIAN_POINT ( 'NONE',  ( 12.01549611932659367, 203.1486557965466773, 76.14886208192143613 ) ) ;
#7289=CARTESIAN_POINT ( 'NONE',  ( 8.015496119326595448, 204.4483345814782638, 55.14886208192145034 ) ) ;
#7296=FACE_OUTER_BOUND ( 'NONE', #22052, .T. ) ;
#7300=CARTESIAN_POINT ( 'NONE',  ( -8.118202686958138514, 212.8392687619910930, 44.79886208192143471 ) ) ;
#7306=CARTESIAN_POINT ( 'NONE',  ( -6.500168698208244500, 211.6636982574061676, 29.79886208192143826 ) ) ;
#7309=CARTESIAN_POINT ( 'NONE',  ( 10.01549611932653860, 210.2015048109876716, 70.85113791807854966 ) ) ;
#7311=CARTESIAN_POINT ( 'NONE',  ( -10.00000000000000711, 207.0476921513413515, 45.50113791807857666 ) ) ;
#7312=CARTESIAN_POINT ( 'NONE',  ( 9.984503880673470277, 203.7031108863295401, 20.15113791807856813 ) ) ;
#7313=CARTESIAN_POINT ( 'NONE',  ( 8.015496119326531499, 209.5516654185219636, 4.851137918078565647 ) ) ;
#7316=CARTESIAN_POINT ( 'NONE',  ( -3.753561863808691168, 195.6020594897209435, 26.90113791807856813 ) ) ;
#7318=CARTESIAN_POINT ( 'NONE',  ( -3.044812012440131443, 216.5253028482142952, 73.10113791807857808 ) ) ;
#7319=CARTESIAN_POINT ( 'NONE',  ( -6.220909254589537696, 198.5229672870051445, 54.05113791807855961 ) ) ;
#7323=CARTESIAN_POINT ( 'NONE',  ( -7.375838497908014268, 196.7627149292498530, 17.04886208192143471 ) ) ;
#7324=CARTESIAN_POINT ( 'NONE',  ( -10.01549611932659545, 210.2015048109875011, 17.64886208192143613 ) ) ;
#7327=CARTESIAN_POINT ( 'NONE',  ( 0.05014649552807549926, 219.6175466908591716, 55.25113791807857666 ) ) ;
#7328=CARTESIAN_POINT ( 'NONE',  ( 6.444103211791042618, 202.2591342207267644, 77.30113791807858092 ) ) ;
#7329=CARTESIAN_POINT ( 'NONE',  ( 0.05014649552828275708, 196.4853777576173002, 37.74886208192143755 ) ) ;
#7339=CARTESIAN_POINT ( 'NONE',  ( -4.903702542908602524, 213.8346818373418898, 30.95113791807857595 ) ) ;
#7341=CARTESIAN_POINT ( 'NONE',  ( -3.044812012439970683, 197.4746971517856196, 16.89886208192143613 ) ) ;
#7344=CARTESIAN_POINT ( 'NONE',  ( -2.426778023690262742, 214.6231898156240163, 55.10113791807857808 ) ) ;
#7347=CARTESIAN_POINT ( 'NONE',  ( -6.220909254589682469, 215.4770327129946850, 98.94886208192140487 ) ) ;
#7349=CARTESIAN_POINT ( 'NONE',  ( 6.220909254589536808, 215.4770327129947702, 37.55113791807856671 ) ) ;
#7351=CARTESIAN_POINT ( 'NONE',  ( 9.984503880673470277, 203.7031108863295401, 20.15113791807856813 ) ) ;
#7352=CARTESIAN_POINT ( 'NONE',  ( 8.062137200540822946, 212.9164362838583315, 99.69886208192144750 ) ) ;
#7357=CARTESIAN_POINT ( 'NONE',  ( -3.044812012440131443, 216.5253028482142952, 100.1011379180785781 ) ) ;
#7360=CARTESIAN_POINT ( 'NONE',  ( -10.00000000000000711, 207.0476921513413515, 45.50113791807857666 ) ) ;
#7366=CARTESIAN_POINT ( 'NONE',  ( 7.375838497908181246, 196.7627149292499666, 29.45113791807856529 ) ) ;
#7368=CARTESIAN_POINT ( 'NONE',  ( -8.118202686958138514, 212.8392687619910930, 14.79886208192143648 ) ) ;
#7370=ORIENTED_EDGE ( 'NONE', *, *, #20639, .T. ) ;
#7371=CARTESIAN_POINT ( 'NONE',  ( -10.00000000000000711, 207.0476921513413515, 9.501137918078566003 ) ) ;
#7372=CARTESIAN_POINT ( 'NONE',  ( -8.118202686958039038, 201.1607312380087080, 57.20113791807857950 ) ) ;
#7374=CARTESIAN_POINT ( 'NONE',  ( -2.426778023690076225, 199.3768101843759553, 22.89886208192143613 ) ) ;
#7377=CARTESIAN_POINT ( 'NONE',  ( 0.05014649552807626948, 215.4116977939061144, 1.251137918078566225 ) ) ;
#7378=CARTESIAN_POINT ( 'NONE',  ( 12.01549611932659367, 203.1486557965466773, 91.14886208192143613 ) ) ;
#7383=CARTESIAN_POINT ( 'NONE',  ( -6.220909254589537696, 198.5229672870051161, 3.051137918078564937 ) ) ;
#7384=CARTESIAN_POINT ( 'NONE',  ( -10.00000000000000711, 206.9523078486584495, 68.49886208192143044 ) ) ;
#7386=CARTESIAN_POINT ( 'NONE',  ( 8.118202686958039038, 212.8392687619912635, 13.70113791807856707 ) ) ;
#7388=EDGE_CURVE ( 'NONE', #28270, #14862, #30398, .T. ) ;
#7390=CARTESIAN_POINT ( 'NONE',  ( -0.05014649552810635652, 196.4853777576173002, 92.75113791807858377 ) ) ;
#7392=CARTESIAN_POINT ( 'NONE',  ( 10.00000000000000711, 206.9523078486586201, 74.00113791807858377 ) ) ;
#7395=CARTESIAN_POINT ( 'NONE',  ( 3.753561863808876797, 195.6020594897209719, 91.59886208192145318 ) ) ;
#7397=CARTESIAN_POINT ( 'NONE',  ( 3.044812012440130555, 197.4746971517856764, 26.60113791807856742 ) ) ;
#7401=CARTESIAN_POINT ( 'NONE',  ( -3.662846001190052991, 218.4274158808045740, 97.10113791807857808 ) ) ;
#7404=CARTESIAN_POINT ( 'NONE',  ( 10.00000000000000711, 207.0476921513415220, 84.99886208192143044 ) ) ;
#7405=CARTESIAN_POINT ( 'NONE',  ( -3.753561863808878130, 218.3979405102790281, 21.09886208192143897 ) ) ;
#7407=CARTESIAN_POINT ( 'NONE',  ( 6.220909254589536808, 215.4770327129947702, 28.55113791807855961 ) ) ;
#7409=CARTESIAN_POINT ( 'NONE',  ( -10.00000000000000711, 206.9523078486584495, 101.4988620819214304 ) ) ;
#7413=CARTESIAN_POINT ( 'NONE',  ( -2.517493886309087880, 214.5937144450984135, 84.09886208192143897 ) ) ;
#7416=ORIENTED_EDGE ( 'NONE', *, *, #29362, .T. ) ;
#7418=CARTESIAN_POINT ( 'NONE',  ( 2.517493886308900919, 214.5937144450984420, 64.40113791807856103 ) ) ;
#7422=CARTESIAN_POINT ( 'NONE',  ( -8.015496119326531499, 204.4483345814780364, 75.35113791807856387 ) ) ;
#7426=CARTESIAN_POINT ( 'NONE',  ( -2.517493886309087880, 214.5937144450984135, 66.09886208192142476 ) ) ;
#7431=CARTESIAN_POINT ( 'NONE',  ( -8.118202686958039038, 201.1607312380087080, 0.2011379180785657361 ) ) ;
#7436=CARTESIAN_POINT ( 'NONE',  ( -0.05014649552807705357, 194.3824533091408000, 71.75113791807856956 ) ) ;
#7438=CARTESIAN_POINT ( 'NONE',  ( -11.98450388067348804, 210.9467285061362247, 9.651137918078566358 ) ) ;
#7439=CARTESIAN_POINT ( 'NONE',  ( 8.062137200540920645, 201.0835637161417822, 92.30113791807858092 ) ) ;
#7440=CARTESIAN_POINT ( 'NONE',  ( 12.01549611932659367, 203.1486557965466773, 43.14886208192143613 ) ) ;
#7441=CARTESIAN_POINT ( 'NONE',  ( 6.139770520408223575, 215.5359834540460611, 57.54886208192142760 ) ) ;
#7443=CARTESIAN_POINT ( 'NONE',  ( -12.00000000000000711, 207.0476921513413515, 96.50113791807856956 ) ) ;
#7445=CARTESIAN_POINT ( 'NONE',  ( -3.135527875058821579, 197.5041725223112223, -0.09886208192143428053 ) ) ;
#7446=CARTESIAN_POINT ( 'NONE',  ( 3.135527875058981895, 197.5041725223112792, 67.59886208192143897 ) ) ;
#7449=CARTESIAN_POINT ( 'NONE',  ( 7.456977232089471386, 196.8216656703012006, 67.44886208192143329 ) ) ;
#7450=CARTESIAN_POINT ( 'NONE',  ( -8.118202686958039038, 201.1607312380087080, 93.20113791807857240 ) ) ;
#7453=CARTESIAN_POINT ( 'NONE',  ( -4.984841277089891776, 213.7757310962905990, 47.94886208192144039 ) ) ;
#7463=CARTESIAN_POINT ( 'NONE',  ( 0.05014649552828275708, 196.4853777576173002, 52.74886208192143044 ) ) ;
#7469=CARTESIAN_POINT ( 'NONE',  ( 4.903702542908435547, 213.8346818373419751, 24.54886208192144181 ) ) ;
#7470=CARTESIAN_POINT ( 'NONE',  ( -3.044812012440131443, 216.5253028482142952, 70.10113791807857808 ) ) ;
#7472=CARTESIAN_POINT ( 'NONE',  ( -8.118202686958039038, 201.1607312380087080, 57.20113791807857950 ) ) ;
#7474=CARTESIAN_POINT ( 'NONE',  ( -3.044812012440131443, 216.5253028482142952, 25.10113791807856742 ) ) ;
#7475=CARTESIAN_POINT ( 'NONE',  ( -6.444103211791042618, 211.7408657792732356, 3.801137918078566269 ) ) ;
#7480=CARTESIAN_POINT ( 'NONE',  ( -3.753561863808691168, 195.6020594897209435, 38.90113791807856813 ) ) ;
#7483=CARTESIAN_POINT ( 'NONE',  ( 3.044812012440130555, 197.4746971517856764, 80.60113791807857808 ) ) ;
#7484=CARTESIAN_POINT ( 'NONE',  ( -10.01549611932653860, 203.7984951890123000, 45.35113791807857808 ) ) ;
#7488=CARTESIAN_POINT ( 'NONE',  ( 3.662846001189864698, 218.4274158808046593, 15.39886208192143613 ) ) ;
#7489=CARTESIAN_POINT ( 'NONE',  ( -10.00000000000000711, 206.9523078486584495, 29.49886208192143400 ) ) ;
#7492=CARTESIAN_POINT ( 'NONE',  ( 12.01549611932652972, 210.8513442034534933, 55.85113791807856387 ) ) ;
#7493=CARTESIAN_POINT ( 'NONE',  ( -8.015496119326531499, 204.4483345814780364, 81.35113791807857808 ) ) ;
#7495=CARTESIAN_POINT ( 'NONE',  ( -3.135527875058982783, 216.4958274776886924, 42.09886208192143897 ) ) ;
#7499=CARTESIAN_POINT ( 'NONE',  ( 0.05014649552828288198, 194.3824533091408000, 43.74886208192143755 ) ) ;
#7504=CARTESIAN_POINT ( 'NONE',  ( 7.703397592599076305, 206.6253034553826637, 111.3476260793010084 ) ) ;
#7506=CARTESIAN_POINT ( 'NONE',  ( -8.000000000000008882, 207.0476921513413515, 36.50113791807857666 ) ) ;
#7509=CARTESIAN_POINT ( 'NONE',  ( 6.220909254589681581, 198.5229672870052582, 19.44886208192142618 ) ) ;
#7512=CARTESIAN_POINT ( 'NONE',  ( -6.444103211791042618, 211.7408657792732356, 60.80113791807858092 ) ) ;
#7516=CARTESIAN_POINT ( 'NONE',  ( 3.044812012439969795, 216.5253028482143520, 102.3988620819214361 ) ) ;
#7518=CARTESIAN_POINT ( 'NONE',  ( 0.05014649552810505201, 217.5146222423826714, 40.25113791807856956 ) ) ;
#7519=CARTESIAN_POINT ( 'NONE',  ( -10.01549611932653860, 203.7984951890123284, 30.35113791807856742 ) ) ;
#7523=CARTESIAN_POINT ( 'NONE',  ( 4.903702542908435547, 213.8346818373419751, 84.54886208192144181 ) ) ;
#7527=CARTESIAN_POINT ( 'NONE',  ( -12.01549611932652972, 203.1486557965464499, 3.351137918078566091 ) ) ;
#7531=CARTESIAN_POINT ( 'NONE',  ( 6.220909254589536808, 215.4770327129947702, 52.55113791807858092 ) ) ;
#7532=EDGE_CURVE ( 'NONE', #6694, #14046, #24978, .T. ) ;
#7535=CARTESIAN_POINT ( 'NONE',  ( -3.044812012439970683, 197.4746971517856196, 1.898862081921434353 ) ) ;
#7538=CARTESIAN_POINT ( 'NONE',  ( -3.662846001190052991, 218.4274158808045740, 25.10113791807856742 ) ) ;
#7542=CARTESIAN_POINT ( 'NONE',  ( -10.00000000000000711, 206.9523078486584495, 14.49886208192143577 ) ) ;
#7546=CARTESIAN_POINT ( 'NONE',  ( 10.00000000000000711, 206.9523078486586201, 11.00113791807856600 ) ) ;
#7547=CARTESIAN_POINT ( 'NONE',  ( -6.139770520408369237, 215.5359834540460042, 69.95113791807857240 ) ) ;
#7549=CARTESIAN_POINT ( 'NONE',  ( 4.984841277089891776, 200.2242689037093726, 28.44886208192142973 ) ) ;
#7552=CARTESIAN_POINT ( 'NONE',  ( 4.903702542908601636, 200.1653181626581102, 5.451137918078566180 ) ) ;
#7553=CARTESIAN_POINT ( 'NONE',  ( -7.375838497908014268, 196.7627149292498530, 89.04886208192142760 ) ) ;
#7558=CARTESIAN_POINT ( 'NONE',  ( -9.984503880673473830, 210.2968891136704315, 3.651137918078565026 ) ) ;
#7560=CARTESIAN_POINT ( 'NONE',  ( 3.044812012439969795, 216.5253028482143520, 75.39886208192143613 ) ) ;
#7563=CARTESIAN_POINT ( 'NONE',  ( 10.01549611932653860, 210.2015048109876716, 13.85113791807856742 ) ) ;
#7567=CARTESIAN_POINT ( 'NONE',  ( -0.05014649552810635652, 196.4853777576173002, 101.7511379180785411 ) ) ;
#7569=CARTESIAN_POINT ( 'NONE',  ( -8.118202686958039038, 201.1607312380087080, 75.20113791807857240 ) ) ;
#7572=CARTESIAN_POINT ( 'NONE',  ( -7.456977232089471386, 217.1783343296987709, 86.94886208192144750 ) ) ;
#7578=CARTESIAN_POINT ( 'NONE',  ( -12.01549611932652972, 203.1486557965464499, 93.35113791807857808 ) ) ;
#7579=CARTESIAN_POINT ( 'NONE',  ( -10.57145583983291992, 206.1290730434410534, 104.2695288710567780 ) ) ;
#7581=CARTESIAN_POINT ( 'NONE',  ( 10.01549611932659367, 203.7984951890124421, 88.14886208192143613 ) ) ;
#7582=CARTESIAN_POINT ( 'NONE',  ( 12.00000000000000711, 207.0476921513415220, 27.99886208192144110 ) ) ;
#7585=CARTESIAN_POINT ( 'NONE',  ( -10.01549611932653860, 203.7984951890123284, 42.35113791807855677 ) ) ;
#7587=CARTESIAN_POINT ( 'NONE',  ( -6.139770520408224463, 198.4640165459539389, 98.04886208192141339 ) ) ;
#7589=CARTESIAN_POINT ( 'NONE',  ( -4.984841277089726574, 200.2242689037092305, 87.05113791807856671 ) ) ;
#7592=CARTESIAN_POINT ( 'NONE',  ( 4.903702542908435547, 213.8346818373419751, 84.54886208192144181 ) ) ;
#7598=CARTESIAN_POINT ( 'NONE',  ( 7.984503880673485376, 204.3529502787953902, 59.15113791807857524 ) ) ;
#7601=CARTESIAN_POINT ( 'NONE',  ( 4.984841277089725686, 213.7757310962907411, 91.55113791807858092 ) ) ;
#7604=CARTESIAN_POINT ( 'NONE',  ( 7.984503880673422316, 209.6470497212048372, 60.84886208192144608 ) ) ;
#7607=CARTESIAN_POINT ( 'NONE',  ( -3.135527875058821579, 197.5041725223112223, 2.901137918078565914 ) ) ;
#7612=CARTESIAN_POINT ( 'NONE',  ( 7.456977232089302632, 217.1783343296989131, 67.55113791807856671 ) ) ;
#7614=CARTESIAN_POINT ( 'NONE',  ( 9.736236675707914401, 214.0148392665762458, 13.70113791807856707 ) ) ;
#7615=CARTESIAN_POINT ( 'NONE',  ( -6.220909254589537696, 198.5229672870051445, 87.05113791807856671 ) ) ;
#7616=CARTESIAN_POINT ( 'NONE',  ( -9.680171189290716072, 199.9079932115567146, 56.19886208192144039 ) ) ;
#7617=CARTESIAN_POINT ( 'NONE',  ( -10.00000000000000711, 206.9523078486584495, 56.49886208192143755 ) ) ;
#7619=CARTESIAN_POINT ( 'NONE',  ( -9.736236675707914401, 199.9851607334237542, 99.20113791807858661 ) ) ;
#7621=CARTESIAN_POINT ( 'NONE',  ( 3.044812012440130555, 197.4746971517856764, -0.3988620819214342972 ) ) ;
#7622=CARTESIAN_POINT ( 'NONE',  ( -6.139770520408224463, 198.4640165459539389, 68.04886208192142760 ) ) ;
#7625=CARTESIAN_POINT ( 'NONE',  ( -3.662846001189865142, 195.5725841191952838, 79.89886208192143613 ) ) ;
#7626=CARTESIAN_POINT ( 'NONE',  ( 6.139770520408368348, 198.4640165459539674, 92.45113791807857240 ) ) ;
#7629=CARTESIAN_POINT ( 'NONE',  ( 7.984503880673422316, 209.6470497212048372, 54.84886208192144608 ) ) ;
#7637=CARTESIAN_POINT ( 'NONE',  ( 8.062137200540822946, 212.9164362838583315, 51.69886208192143329 ) ) ;
#7641=CARTESIAN_POINT ( 'NONE',  ( -2.517493886309087880, 214.5937144450984135, 39.09886208192143897 ) ) ;
#7642=CARTESIAN_POINT ( 'NONE',  ( 3.135527875058820690, 216.4958274776887492, 67.40113791807857524 ) ) ;
#7644=CARTESIAN_POINT ( 'NONE',  ( 10.00000000000000711, 206.9523078486586201, 59.00113791807857666 ) ) ;
#7646=CARTESIAN_POINT ( 'NONE',  ( 0.05014649552810505201, 217.5146222423826714, 31.25113791807857311 ) ) ;
#7647=CARTESIAN_POINT ( 'NONE',  ( 8.015496119326531499, 209.5516654185219636, 19.85113791807856387 ) ) ;
#7651=CARTESIAN_POINT ( 'NONE',  ( -7.456977232089304408, 196.8216656703010301, 36.05113791807855961 ) ) ;
#7653=CARTESIAN_POINT ( 'NONE',  ( -9.984503880673473830, 210.2968891136704315, 81.65113791807857524 ) ) ;
#7654=CARTESIAN_POINT ( 'NONE',  ( 8.118202686958039038, 212.8392687619912635, 55.70113791807857950 ) ) ;
#7656=CARTESIAN_POINT ( 'NONE',  ( 12.01549611932659367, 203.1486557965466773, 25.14886208192143258 ) ) ;
#7657=CARTESIAN_POINT ( 'NONE',  ( 10.01549611932659367, 203.7984951890124421, 31.14886208192143613 ) ) ;
#7660=CARTESIAN_POINT ( 'NONE',  ( 11.98450388067348271, 203.0532714938637753, 71.15113791807857524 ) ) ;
#7661=CARTESIAN_POINT ( 'NONE',  ( 4.903702542908601636, 200.1653181626581102, 83.45113791807857240 ) ) ;
#7662=CARTESIAN_POINT ( 'NONE',  ( 3.135527875058981895, 197.5041725223112792, 43.59886208192143897 ) ) ;
#7666=CARTESIAN_POINT ( 'NONE',  ( -3.753561863808878130, 218.3979405102790281, 51.09886208192143897 ) ) ;
#7673=CARTESIAN_POINT ( 'NONE',  ( 2.426778023690261410, 199.3768101843759837, 44.60113791807857098 ) ) ;
#7675=CARTESIAN_POINT ( 'NONE',  ( 3.135527875058981895, 197.5041725223112792, 19.59886208192143542 ) ) ;
#7681=CARTESIAN_POINT ( 'NONE',  ( 0.05014649552828262524, 198.5883022060938572, 4.748862081921434886 ) ) ;
#7682=CARTESIAN_POINT ( 'NONE',  ( -8.062137200540920645, 212.9164362838581894, 39.80113791807857382 ) ) ;
#7684=CARTESIAN_POINT ( 'NONE',  ( -3.044812012440131443, 216.5253028482142952, 28.10113791807857098 ) ) ;
#7685=DIRECTION ( 'NONE',  ( 0.000000000000000000, -0.04769215134144032253, 0.9988620819214358848 ) ) ;
#7688=CARTESIAN_POINT ( 'NONE',  ( -2.517493886309087880, 214.5937144450984135, 81.09886208192143897 ) ) ;
#7692=CARTESIAN_POINT ( 'NONE',  ( 3.662846001190051659, 195.5725841191953691, 11.60113791807856742 ) ) ;
#7696=CARTESIAN_POINT ( 'NONE',  ( -8.118202686958039038, 201.1607312380087080, 54.20113791807857240 ) ) ;
#7699=CARTESIAN_POINT ( 'NONE',  ( -8.118202686958138514, 212.8392687619910930, 2.798862081921434708 ) ) ;
#7702=CARTESIAN_POINT ( 'NONE',  ( 7.375838497908181246, 196.7627149292499666, 41.45113791807857240 ) ) ;
#7704=CARTESIAN_POINT ( 'NONE',  ( -10.01549611932659722, 210.2015048109875011, 14.64886208192143258 ) ) ;
#7707=CARTESIAN_POINT ( 'NONE',  ( -9.984503880673473830, 210.2968891136704315, 12.65113791807856281 ) ) ;
#7708=CARTESIAN_POINT ( 'NONE',  ( 6.139770520408368348, 198.4640165459539674, 68.45113791807858661 ) ) ;
#7710=CARTESIAN_POINT ( 'NONE',  ( -2.426778023690076225, 199.3768101843759553, 28.89886208192143613 ) ) ;
#7713=CARTESIAN_POINT ( 'NONE',  ( -4.903702542908602524, 213.8346818373418898, 15.95113791807856707 ) ) ;
#7716=CARTESIAN_POINT ( 'NONE',  ( -0.05014649552828442242, 219.6175466908591716, 102.2488620819214447 ) ) ;
#7721=CARTESIAN_POINT ( 'NONE',  ( 0.05014649552810505201, 217.5146222423826714, 10.25113791807856778 ) ) ;
#7722=CARTESIAN_POINT ( 'NONE',  ( 0.05014649552828275708, 196.4853777576173002, 70.74886208192143044 ) ) ;
#7725=CARTESIAN_POINT ( 'NONE',  ( 6.139770520408368348, 198.4640165459539674, 11.45113791807856707 ) ) ;
#7729=CARTESIAN_POINT ( 'NONE',  ( 8.062137200540920645, 201.0835637161417822, 98.30113791807858092 ) ) ;
#7731=CARTESIAN_POINT ( 'NONE',  ( 3.044812012440130555, 197.4746971517856764, 86.60113791807857808 ) ) ;
#7735=CARTESIAN_POINT ( 'NONE',  ( -0.05014649552828442242, 219.6175466908591716, 96.24886208192144466 ) ) ;
#7741=CARTESIAN_POINT ( 'NONE',  ( 7.456977232089302632, 217.1783343296989131, 100.5511379180785809 ) ) ;
#7744=CARTESIAN_POINT ( 'NONE',  ( 9.984503880673420539, 210.2968891136705736, 81.84886208192143897 ) ) ;
#7746=CARTESIAN_POINT ( 'NONE',  ( 9.736236675708031640, 199.9851607334238963, 25.29886208192143826 ) ) ;
#7748=CARTESIAN_POINT ( 'NONE',  ( -8.062137200540920645, 212.9164362838581894, 45.80113791807856671 ) ) ;
#7750=CARTESIAN_POINT ( 'NONE',  ( -4.984841277089891776, 213.7757310962905990, 5.948862081921435063 ) ) ;
#7753=CARTESIAN_POINT ( 'NONE',  ( 2.517493886309087436, 199.4062855549015865, 88.59886208192143897 ) ) ;
#7755=CARTESIAN_POINT ( 'NONE',  ( 6.500168698208129925, 211.6636982574063381, 34.70113791807857240 ) ) ;
#7762=CARTESIAN_POINT ( 'NONE',  ( 4.903702542908601636, 200.1653181626581102, 89.45113791807857240 ) ) ;
#7767=CARTESIAN_POINT ( 'NONE',  ( 4.984841277089891776, 200.2242689037093726, 61.44886208192144039 ) ) ;
#7768=DIRECTION ( 'NONE',  ( -0.9891821073486152249, -0.1466927349985424900, -2.962715634069391535E-17 ) ) ;
#7775=CARTESIAN_POINT ( 'NONE',  ( 7.456977232089302632, 217.1783343296989131, 64.55113791807856671 ) ) ;
#7777=CARTESIAN_POINT ( 'NONE',  ( 9.680171189290831535, 199.9079932115568852, 8.301137918078564937 ) ) ;
#7778=CARTESIAN_POINT ( 'NONE',  ( 6.139770520408367460, 198.4640165459539389, 89.45113791807857240 ) ) ;
#7779=CARTESIAN_POINT ( 'NONE',  ( -0.05014649552828442242, 219.6175466908591716, 48.24886208192144466 ) ) ;
#7781=CARTESIAN_POINT ( 'NONE',  ( -10.00000000000000711, 206.9523078486584495, 53.49886208192143755 ) ) ;
#7782=CARTESIAN_POINT ( 'NONE',  ( -3.753561863808691168, 195.6020594897209435, 95.90113791807857524 ) ) ;
#7784=CARTESIAN_POINT ( 'NONE',  ( 8.118202686958039038, 212.8392687619912635, 13.70113791807856707 ) ) ;
#7785=CARTESIAN_POINT ( 'NONE',  ( -8.062137200540822946, 201.0835637161416400, 77.19886208192143329 ) ) ;
#7787=CARTESIAN_POINT ( 'NONE',  ( 7.456977232089471386, 196.8216656703012006, 79.44886208192144750 ) ) ;
#7788=CARTESIAN_POINT ( 'NONE',  ( -9.984503880673473830, 210.2968891136704315, 96.65113791807857524 ) ) ;
#7792=CARTESIAN_POINT ( 'NONE',  ( 6.444103211790928043, 211.7408657792734061, 54.69886208192144039 ) ) ;
#7800=CARTESIAN_POINT ( 'NONE',  ( -0.05014649552828403384, 217.5146222423826714, 51.24886208192143755 ) ) ;
#7805=CARTESIAN_POINT ( 'NONE',  ( -7.984503880673422316, 204.3529502787951628, 32.34886208192143897 ) ) ;
#7806=CARTESIAN_POINT ( 'NONE',  ( -10.00000000000000711, 207.0476921513413515, 66.50113791807856956 ) ) ;
#7809=CARTESIAN_POINT ( 'NONE',  ( 8.062137200540920645, 201.0835637161417822, 56.30113791807857382 ) ) ;
#7810=CARTESIAN_POINT ( 'NONE',  ( 10.00000000000000711, 206.9523078486586201, 32.00113791807856956 ) ) ;
#7811=CARTESIAN_POINT ( 'NONE',  ( 4.984841277089725686, 213.7757310962907411, 16.55113791807857027 ) ) ;
#7816=CARTESIAN_POINT ( 'NONE',  ( -11.98450388067348804, 210.9467285061362247, 36.65113791807856103 ) ) ;
#7819=CARTESIAN_POINT ( 'NONE',  ( 6.220909254589536808, 215.4770327129947702, 85.55113791807858092 ) ) ;
#7820=CARTESIAN_POINT ( 'NONE',  ( 8.062137200540920645, 201.0835637161417822, 56.30113791807857382 ) ) ;
#7823=CARTESIAN_POINT ( 'NONE',  ( -9.680171189290716072, 199.9079932115567146, 23.19886208192143684 ) ) ;
#7824=CARTESIAN_POINT ( 'NONE',  ( -3.135527875058982783, 216.4958274776886924, 24.09886208192143542 ) ) ;
#7826=CARTESIAN_POINT ( 'NONE',  ( -11.98450388067348804, 210.9467285061362247, 63.65113791807855392 ) ) ;
#7827=CARTESIAN_POINT ( 'NONE',  ( 4.903702542908601636, 200.1653181626581102, 86.45113791807858661 ) ) ;
#7829=CARTESIAN_POINT ( 'NONE',  ( -10.01549611932659722, 210.2015048109875011, 44.64886208192143613 ) ) ;
#7832=CARTESIAN_POINT ( 'NONE',  ( 3.662846001189864698, 218.4274158808046593, 51.39886208192144323 ) ) ;
#7841=CARTESIAN_POINT ( 'NONE',  ( 6.500168698208129925, 211.6636982574063381, 40.70113791807857240 ) ) ;
#7844=CARTESIAN_POINT ( 'NONE',  ( -3.135527875058982783, 216.4958274776886924, 27.09886208192143542 ) ) ;
#7850=CARTESIAN_POINT ( 'NONE',  ( -7.984503880673422316, 204.3529502787951628, 2.348862081921434974 ) ) ;
#7851=CARTESIAN_POINT ( 'NONE',  ( 3.135527875058820690, 216.4958274776887492, 43.40113791807856813 ) ) ;
#7854=CARTESIAN_POINT ( 'NONE',  ( -8.118202686958039038, 201.1607312380087080, 24.20113791807856884 ) ) ;
#7855=CARTESIAN_POINT ( 'NONE',  ( 10.01549611932659367, 203.7984951890124421, 100.1488620819214361 ) ) ;
#7856=CARTESIAN_POINT ( 'NONE',  ( 7.984503880673422316, 209.6470497212048372, 93.84886208192143897 ) ) ;
#7860=CARTESIAN_POINT ( 'NONE',  ( 3.753561863808689836, 218.3979405102790565, 13.40113791807856636 ) ) ;
#7863=CARTESIAN_POINT ( 'NONE',  ( -8.062137200540920645, 212.9164362838581894, 51.80113791807857382 ) ) ;
#7870=CARTESIAN_POINT ( 'NONE',  ( 0.05014649552807549926, 219.6175466908591716, 34.25113791807857666 ) ) ;
#7873=CARTESIAN_POINT ( 'NONE',  ( -8.062137200540822946, 201.0835637161416400, 11.19886208192143506 ) ) ;
#7876=CARTESIAN_POINT ( 'NONE',  ( -6.220909254589537696, 198.5229672870051161, 12.05113791807856671 ) ) ;
#7877=CARTESIAN_POINT ( 'NONE',  ( -3.135527875058821579, 197.5041725223112223, 71.90113791807857524 ) ) ;
#7880=CARTESIAN_POINT ( 'NONE',  ( -2.426778023690076225, 199.3768101843759553, 34.89886208192144323 ) ) ;
#7884=CARTESIAN_POINT ( 'NONE',  ( 4.903702542908601636, 200.1653181626581102, 11.45113791807856529 ) ) ;
#7886=CARTESIAN_POINT ( 'NONE',  ( 7.456977232089471386, 196.8216656703012006, 94.44886208192143329 ) ) ;
#7891=CARTESIAN_POINT ( 'NONE',  ( -3.135527875058821579, 197.5041725223112223, 11.90113791807856636 ) ) ;
#7892=CARTESIAN_POINT ( 'NONE',  ( 10.00000000000000711, 207.0476921513415220, 81.99886208192143044 ) ) ;
#7895=CARTESIAN_POINT ( 'NONE',  ( 3.135527875058820690, 216.4958274776887492, 16.40113791807856813 ) ) ;
#7897=EDGE_CURVE ( 'NONE', #20665, #16872, #16820, .T. ) ;
#7901=CARTESIAN_POINT ( 'NONE',  ( 3.135527875058820690, 216.4958274776887492, 88.40113791807857524 ) ) ;
#7904=CARTESIAN_POINT ( 'NONE',  ( -3.662846001189865142, 195.5725841191952838, 100.8988620819214361 ) ) ;
#7909=CARTESIAN_POINT ( 'NONE',  ( 11.98450388067348271, 203.0532714938637753, 98.15113791807856103 ) ) ;
#7914=CARTESIAN_POINT ( 'NONE',  ( 8.118202686958138514, 201.1607312380088501, 85.29886208192144181 ) ) ;
#7915=CARTESIAN_POINT ( 'NONE',  ( 9.736236675708031640, 199.9851607334238963, 19.29886208192143471 ) ) ;
#7917=CARTESIAN_POINT ( 'NONE',  ( -0.05014649552810635652, 196.4853777576173002, 41.75113791807855534 ) ) ;
#7920=CARTESIAN_POINT ( 'NONE',  ( 6.444103211790928043, 211.7408657792734061, 6.698862081921435063 ) ) ;
#7923=CARTESIAN_POINT ( 'NONE',  ( -4.903702542908436435, 200.1653181626580249, 92.04886208192142760 ) ) ;
#7926=CARTESIAN_POINT ( 'NONE',  ( -0.05014649552807731031, 198.5883022060938572, 29.75113791807856956 ) ) ;
#7932=CARTESIAN_POINT ( 'NONE',  ( 6.500168698208129925, 211.6636982574063381, 91.70113791807857240 ) ) ;
#7936=CARTESIAN_POINT ( 'NONE',  ( -8.015496119326597224, 209.5516654185217362, 62.64886208192143613 ) ) ;
#7943=CARTESIAN_POINT ( 'NONE',  ( -9.736236675707914401, 199.9851607334237542, 72.20113791807857240 ) ) ;
#7945=CARTESIAN_POINT ( 'NONE',  ( -9.736236675707914401, 199.9851607334237542, 9.201137918078563516 ) ) ;
#7947=CARTESIAN_POINT ( 'NONE',  ( 8.062137200540920645, 201.0835637161417822, 89.30113791807858092 ) ) ;
#7949=CARTESIAN_POINT ( 'NONE',  ( -3.753561863808878130, 218.3979405102790281, 48.09886208192143897 ) ) ;
#7950=CARTESIAN_POINT ( 'NONE',  ( 10.00000000000000711, 207.0476921513415220, 57.99886208192143044 ) ) ;
#7951=CARTESIAN_POINT ( 'NONE',  ( -11.98450388067348804, 210.9467285061362247, 99.65113791807858945 ) ) ;
#7953=CARTESIAN_POINT ( 'NONE',  ( -10.01549611932653860, 203.7984951890123284, 12.35113791807856387 ) ) ;
#7955=CARTESIAN_POINT ( 'NONE',  ( 8.062137200540822946, 212.9164362838583315, 81.69886208192143329 ) ) ;
#7957=CARTESIAN_POINT ( 'NONE',  ( -9.736236675708031640, 214.0148392665760753, 80.79886208192144181 ) ) ;
#7961=CARTESIAN_POINT ( 'NONE',  ( -4.984841277089891776, 213.7757310962905990, 56.94886208192144039 ) ) ;
#7969=CARTESIAN_POINT ( 'NONE',  ( 10.01549611932659545, 203.7984951890123853, 52.14886208192142192 ) ) ;
#7976=CARTESIAN_POINT ( 'NONE',  ( 8.000000000000008882, 207.0476921513415220, 33.99886208192143755 ) ) ;
#7977=CARTESIAN_POINT ( 'NONE',  ( -6.220909254589537696, 198.5229672870051161, 84.05113791807855250 ) ) ;
#7979=CARTESIAN_POINT ( 'NONE',  ( -6.139770520408369237, 215.5359834540460042, 51.95113791807857950 ) ) ;
#7981=CARTESIAN_POINT ( 'NONE',  ( 9.984503880673470277, 203.7031108863295401, 29.15113791807856103 ) ) ;
#7982=CARTESIAN_POINT ( 'NONE',  ( 8.015496119326531499, 209.5516654185219636, 13.85113791807856742 ) ) ;
#7986=CARTESIAN_POINT ( 'NONE',  ( 3.753561863808689836, 218.3979405102790565, 43.40113791807856813 ) ) ;
#7988=CARTESIAN_POINT ( 'NONE',  ( -6.139770520408369237, 215.5359834540460042, 87.95113791807858661 ) ) ;
#7989=CARTESIAN_POINT ( 'NONE',  ( -8.118202686958039038, 201.1607312380087080, 57.20113791807857950 ) ) ;
#7990=CARTESIAN_POINT ( 'NONE',  ( 7.375838497908012492, 217.2372850707501186, 24.54886208192144181 ) ) ;
#7991=CARTESIAN_POINT ( 'NONE',  ( 8.062137200540822946, 212.9164362838583315, 27.69886208192143684 ) ) ;
#7993=CARTESIAN_POINT ( 'NONE',  ( 12.00000000000000711, 206.9523078486586485, 65.00113791807856956 ) ) ;
#7994=CARTESIAN_POINT ( 'NONE',  ( 4.984841277089725686, 213.7757310962907411, 88.55113791807858092 ) ) ;
#7995=CARTESIAN_POINT ( 'NONE',  ( 10.01549611932659545, 203.7984951890123853, 49.14886208192143613 ) ) ;
#7998=EDGE_CURVE ( 'NONE', #860, #29176, #10858, .T. ) ;
#8000=CARTESIAN_POINT ( 'NONE',  ( -7.375838497908014268, 196.7627149292498530, 56.04886208192144181 ) ) ;
#8007=CARTESIAN_POINT ( 'NONE',  ( 8.015496119326531499, 209.5516654185219636, 40.85113791807856387 ) ) ;
#8009=CARTESIAN_POINT ( 'NONE',  ( 0.05014649552828275708, 196.4853777576173002, 25.74886208192143400 ) ) ;
#8012=DIRECTION ( 'NONE',  ( -0.8309481877611850642, 0.02653351925882575443, 0.5557167278498498231 ) ) ;
#8014=CARTESIAN_POINT ( 'NONE',  ( 2.426778023690075337, 214.6231898156240447, 9.398862081921436129 ) ) ;
#8016=CARTESIAN_POINT ( 'NONE',  ( -10.00000000000000711, 207.0476921513413515, 45.50113791807857666 ) ) ;
#8017=CARTESIAN_POINT ( 'NONE',  ( 6.220909254589536808, 215.4770327129947702, 31.55113791807857382 ) ) ;
#8021=AXIS2_PLACEMENT_3D ( 'NONE', #4259, #30497, #14317 ) ;
#8022=CARTESIAN_POINT ( 'NONE',  ( -8.000000000000008882, 206.9523078486584780, 95.49886208192144466 ) ) ;
#8026=CARTESIAN_POINT ( 'NONE',  ( -9.680171189290831535, 214.0920067884431148, 6.801137918078565825 ) ) ;
#8029=CARTESIAN_POINT ( 'NONE',  ( -3.135527875058821579, 197.5041725223112223, 59.90113791807856813 ) ) ;
#8030=CARTESIAN_POINT ( 'NONE',  ( 8.062137200540920645, 201.0835637161417822, 29.30113791807857027 ) ) ;
#8037=CARTESIAN_POINT ( 'NONE',  ( -12.00000000000000711, 207.0476921513413515, 42.50113791807856245 ) ) ;
#8039=CARTESIAN_POINT ( 'NONE',  ( -8.118202686958138514, 212.8392687619910930, 20.79886208192143471 ) ) ;
#8042=CARTESIAN_POINT ( 'NONE',  ( 10.00000000000000711, 206.9523078486586201, 68.00113791807856956 ) ) ;
#8051=CARTESIAN_POINT ( 'NONE',  ( 4.903702542908601636, 200.1653181626581102, 17.45113791807856174 ) ) ;
#8052=CARTESIAN_POINT ( 'NONE',  ( 12.00000000000000711, 207.0476921513415220, 99.99886208192143044 ) ) ;
#8058=CARTESIAN_POINT ( 'NONE',  ( -3.044812012440131443, 216.5253028482142952, 10.10113791807856565 ) ) ;
#8059=CARTESIAN_POINT ( 'NONE',  ( 3.044812012439969795, 216.5253028482143520, 81.39886208192145034 ) ) ;
#8062=CARTESIAN_POINT ( 'NONE',  ( -6.220909254589537696, 198.5229672870051161, 12.05113791807856671 ) ) ;
#8067=CARTESIAN_POINT ( 'NONE',  ( -3.044812012440131443, 216.5253028482142952, 85.10113791807857808 ) ) ;
#8071=CARTESIAN_POINT ( 'NONE',  ( -9.736236675708031640, 214.0148392665760753, 92.79886208192142760 ) ) ;
#8077=CARTESIAN_POINT ( 'NONE',  ( 7.456977232089471386, 196.8216656703012006, 4.448862081921434175 ) ) ;
#8082=CARTESIAN_POINT ( 'NONE',  ( -9.984503880673420539, 203.7031108863293980, 98.34886208192143897 ) ) ;
#8083=CARTESIAN_POINT ( 'NONE',  ( 9.736236675708031640, 199.9851607334238963, 22.29886208192143826 ) ) ;
#8085=CARTESIAN_POINT ( 'NONE',  ( 8.118202686958039038, 212.8392687619912635, 37.70113791807857240 ) ) ;
#8087=CARTESIAN_POINT ( 'NONE',  ( -2.426778023690076225, 199.3768101843759553, 1.898862081921434797 ) ) ;
#8091=CARTESIAN_POINT ( 'NONE',  ( 0.05014649552828262524, 198.5883022060938572, 85.74886208192143044 ) ) ;
#8092=B_SPLINE_CURVE_WITH_KNOTS ( 'NONE', 3,
 ( #3876, #16825, #32832, #1496, #11890, #12395 ),
 .UNSPECIFIED., .F., .F.,
 ( 4, 2, 4 ),
 ( -6.326732604037524437E-06, 0.0006895418312384076452, 0.001385410395080852695 ),
 .UNSPECIFIED. ) ;
#8094=CARTESIAN_POINT ( 'NONE',  ( -4.903702542908602524, 213.8346818373418898, 27.95113791807857240 ) ) ;
#8101=CARTESIAN_POINT ( 'NONE',  ( -0.05014649552807731031, 198.5883022060938572, 92.75113791807858377 ) ) ;
#8105=CARTESIAN_POINT ( 'NONE',  ( -0.05014649552828365914, 215.4116977939061144, 60.24886208192144466 ) ) ;
#8109=CARTESIAN_POINT ( 'NONE',  ( -3.044812012440131443, 216.5253028482142952, 1.101137918078565869 ) ) ;
#8114=CARTESIAN_POINT ( 'NONE',  ( 12.00000000000000711, 206.9523078486586485, 71.00113791807856956 ) ) ;
#8117=CARTESIAN_POINT ( 'NONE',  ( -3.044812012440131443, 216.5253028482142952, 88.10113791807857808 ) ) ;
#8120=CARTESIAN_POINT ( 'NONE',  ( -9.680171189290716072, 199.9079932115567146, 53.19886208192144039 ) ) ;
#8121=CARTESIAN_POINT ( 'NONE',  ( 10.00000000000000711, 207.0476921513415220, 69.99886208192143044 ) ) ;
#8122=CARTESIAN_POINT ( 'NONE',  ( -0.05014649552807705357, 194.3824533091408000, 92.75113791807858377 ) ) ;
#8124=CARTESIAN_POINT ( 'NONE',  ( -10.00000000000000711, 207.0476921513413515, 9.501137918078566003 ) ) ;
#8125=CARTESIAN_POINT ( 'NONE',  ( 6.139770520408223575, 215.5359834540460611, 78.54886208192144181 ) ) ;
#8128=CARTESIAN_POINT ( 'NONE',  ( 6.220909254589536808, 215.4770327129947702, 97.55113791807855250 ) ) ;
#8131=CARTESIAN_POINT ( 'NONE',  ( -2.517493886309087880, 214.5937144450984135, 63.09886208192143187 ) ) ;
#8138=CARTESIAN_POINT ( 'NONE',  ( -0.05014649552807731031, 198.5883022060938572, 62.75113791807856245 ) ) ;
#8144=CARTESIAN_POINT ( 'NONE',  ( 4.903702542908435547, 213.8346818373419751, 33.54886208192144181 ) ) ;
#8145=CARTESIAN_POINT ( 'NONE',  ( -6.139770520408369237, 215.5359834540460042, 78.95113791807858661 ) ) ;
#8148=CARTESIAN_POINT ( 'NONE',  ( 8.118202686958039038, 212.8392687619912635, 55.70113791807857950 ) ) ;
#8149=CARTESIAN_POINT ( 'NONE',  ( -0.05014649552810635652, 196.4853777576173002, 23.75113791807855890 ) ) ;
#8150=CARTESIAN_POINT ( 'NONE',  ( 8.000000000000008882, 206.9523078486586485, 17.00113791807856956 ) ) ;
#8154=CARTESIAN_POINT ( 'NONE',  ( -3.662846001190052991, 218.4274158808045740, 37.10113791807855677 ) ) ;
#8157=CARTESIAN_POINT ( 'NONE',  ( -9.984503880673473830, 210.2968891136704315, 84.65113791807857524 ) ) ;
#8158=CARTESIAN_POINT ( 'NONE',  ( -6.139770520408368348, 215.5359834540460042, 60.95113791807857240 ) ) ;
#8159=CARTESIAN_POINT ( 'NONE',  ( -3.662846001189865142, 195.5725841191952838, 25.89886208192143613 ) ) ;
#8160=CARTESIAN_POINT ( 'NONE',  ( -8.118202686958138514, 212.8392687619910930, 26.79886208192143826 ) ) ;
#8162=CARTESIAN_POINT ( 'NONE',  ( -3.753561863808691168, 195.6020594897209435, 65.90113791807856103 ) ) ;
#8164=CARTESIAN_POINT ( 'NONE',  ( -2.517493886308901807, 199.4062855549015012, 92.90113791807857524 ) ) ;
#8165=CARTESIAN_POINT ( 'NONE',  ( -0.05014649552828403384, 217.5146222423826714, 48.24886208192142334 ) ) ;
#8168=CARTESIAN_POINT ( 'NONE',  ( 9.736236675708031640, 199.9851607334238963, 49.29886208192143471 ) ) ;
#8174=CARTESIAN_POINT ( 'NONE',  ( -6.444103211791042618, 211.7408657792732356, 42.80113791807857382 ) ) ;
#8176=CARTESIAN_POINT ( 'NONE',  ( -3.135527875058982783, 216.4958274776886924, 21.09886208192143897 ) ) ;
#8182=CARTESIAN_POINT ( 'NONE',  ( 8.000000000000008882, 207.0476921513415220, 3.998862081921434442 ) ) ;
#8183=CARTESIAN_POINT ( 'NONE',  ( 3.135527875058820690, 216.4958274776887492, 52.40113791807857524 ) ) ;
#8186=CARTESIAN_POINT ( 'NONE',  ( -6.220909254589537696, 198.5229672870051161, 27.05113791807856671 ) ) ;
#8189=CARTESIAN_POINT ( 'NONE',  ( -8.000000000000008882, 206.9523078486584780, 89.49886208192144466 ) ) ;
#8193=CARTESIAN_POINT ( 'NONE',  ( -11.98450388067348804, 210.9467285061362247, 9.651137918078566358 ) ) ;
#8196=CARTESIAN_POINT ( 'NONE',  ( 0.05014649552810505201, 217.5146222423826714, 52.25113791807856245 ) ) ;
#8197=CARTESIAN_POINT ( 'NONE',  ( -10.00000000000000711, 207.0476921513413515, 33.50113791807856956 ) ) ;
#8200=CARTESIAN_POINT ( 'NONE',  ( 0.05014649552828275014, 196.4853777576173002, 1.748862081921434442 ) ) ;
#8203=CARTESIAN_POINT ( 'NONE',  ( 7.456977232089302632, 217.1783343296989131, 43.55113791807857382 ) ) ;
#8205=CARTESIAN_POINT ( 'NONE',  ( 6.139770520408223575, 215.5359834540460611, 24.54886208192143471 ) ) ;
#8208=CARTESIAN_POINT ( 'NONE',  ( -8.118202686958039038, 201.1607312380087080, 72.20113791807857240 ) ) ;
#8212=ORIENTED_EDGE ( 'NONE', *, *, #16174, .T. ) ;
#8213=CARTESIAN_POINT ( 'NONE',  ( 2.426778023690261410, 199.3768101843759837, 8.601137918078565647 ) ) ;
#8214=CARTESIAN_POINT ( 'NONE',  ( 9.736236675708031640, 199.9851607334238963, 94.29886208192142760 ) ) ;
#8219=CARTESIAN_POINT ( 'NONE',  ( 9.984503880673470277, 203.7031108863295401, 5.151137918078567246 ) ) ;
#8220=CARTESIAN_POINT ( 'NONE',  ( 8.062137200540822946, 212.9164362838583315, 84.69886208192144750 ) ) ;
#8222=CARTESIAN_POINT ( 'NONE',  ( -10.01549611932653860, 203.7984951890123284, 24.35113791807855677 ) ) ;
#8225=CARTESIAN_POINT ( 'NONE',  ( -10.00000000000000711, 207.0476921513413515, 99.50113791807856956 ) ) ;
#8227=CARTESIAN_POINT ( 'NONE',  ( -0.05014649552810635652, 196.4853777576173002, 89.75113791807854113 ) ) ;
#8230=CARTESIAN_POINT ( 'NONE',  ( 12.01549611932659367, 203.1486557965466773, 97.14886208192146455 ) ) ;
#8239=CARTESIAN_POINT ( 'NONE',  ( 0.05014649552828275014, 196.4853777576173002, 97.74886208192141623 ) ) ;
#8241=CARTESIAN_POINT ( 'NONE',  ( 11.98450388067341876, 210.9467285061363953, 30.84886208192143542 ) ) ;
#8243=CARTESIAN_POINT ( 'NONE',  ( 9.984503880673470277, 203.7031108863295401, 41.15113791807855392 ) ) ;
#8246=CARTESIAN_POINT ( 'NONE',  ( -10.05084501415679732, 217.6133941545940047, 104.9910338291041683 ) ) ;
#8249=CARTESIAN_POINT ( 'NONE',  ( 6.500168698208244500, 202.3363017425938324, 91.29886208192142760 ) ) ;
#8250=CARTESIAN_POINT ( 'NONE',  ( 2.517493886308900919, 214.5937144450984420, 31.40113791807857879 ) ) ;
#8256=CARTESIAN_POINT ( 'NONE',  ( -4.903702542908602524, 213.8346818373418898, 84.95113791807858661 ) ) ;
#8260=CARTESIAN_POINT ( 'NONE',  ( 4.984841277089891776, 200.2242689037093726, 70.44886208192144750 ) ) ;
#8264=CARTESIAN_POINT ( 'NONE',  ( 8.118202686958039038, 212.8392687619912635, 13.70113791807856707 ) ) ;
#8267=AXIS2_PLACEMENT_3D ( 'NONE', #32413, #9080, #27309 ) ;
#8270=CARTESIAN_POINT ( 'NONE',  ( -11.98450388067348804, 210.9467285061362247, 78.65113791807858945 ) ) ;
#8273=CARTESIAN_POINT ( 'NONE',  ( -3.135527875058821579, 197.5041725223112223, 95.90113791807858945 ) ) ;
#8274=CARTESIAN_POINT ( 'NONE',  ( -10.17386985161379620, 208.0352956435529563, 102.7846294209004441 ) ) ;
#8277=CARTESIAN_POINT ( 'NONE',  ( -0.05014649552828442242, 219.6175466908591716, 63.24886208192142334 ) ) ;
#8278=CARTESIAN_POINT ( 'NONE',  ( -8.118202686958138514, 212.8392687619910930, 71.79886208192142760 ) ) ;
#8279=CARTESIAN_POINT ( 'NONE',  ( -9.680171189290716072, 199.9079932115567146, 5.198862081921434175 ) ) ;
#8281=CARTESIAN_POINT ( 'NONE',  ( 0.05014649552810505201, 217.5146222423826714, 13.25113791807856778 ) ) ;
#8282=CARTESIAN_POINT ( 'NONE',  ( 10.01549611932659545, 203.7984951890123853, 82.14886208192140771 ) ) ;
#8287=CARTESIAN_POINT ( 'NONE',  ( -7.984503880673422316, 204.3529502787951628, 59.34886208192144608 ) ) ;
#8297=CARTESIAN_POINT ( 'NONE',  ( 4.903702542908601636, 200.1653181626581102, 62.45113791807857240 ) ) ;
#8300=CARTESIAN_POINT ( 'NONE',  ( -2.426778023690076225, 199.3768101843759553, 37.89886208192144323 ) ) ;
#8301=CARTESIAN_POINT ( 'NONE',  ( -6.139770520408369237, 215.5359834540460042, 84.95113791807858661 ) ) ;
#8303=CARTESIAN_POINT ( 'NONE',  ( 6.220909254589536808, 215.4770327129947702, 64.55113791807858092 ) ) ;
#8306=CARTESIAN_POINT ( 'NONE',  ( 7.984503880673485376, 204.3529502787953902, 14.15113791807856991 ) ) ;
#8310=CARTESIAN_POINT ( 'NONE',  ( 11.98450388067348271, 203.0532714938637753, 53.15113791807857524 ) ) ;
#8312=CARTESIAN_POINT ( 'NONE',  ( 10.01549611932653860, 210.2015048109876716, 94.85113791807857808 ) ) ;
#8313=CARTESIAN_POINT ( 'NONE',  ( 10.00000000000000711, 206.9523078486586201, 59.00113791807857666 ) ) ;
#8314=CARTESIAN_POINT ( 'NONE',  ( -12.01549611932659722, 210.8513442034533227, 26.64886208192143968 ) ) ;
#8315=CARTESIAN_POINT ( 'NONE',  ( 10.01549611932659367, 203.7984951890124421, 37.14886208192142192 ) ) ;
#8318=CARTESIAN_POINT ( 'NONE',  ( 9.736236675707914401, 214.0148392665762458, 67.70113791807857240 ) ) ;
#8319=CARTESIAN_POINT ( 'NONE',  ( -4.984841277089726574, 200.2242689037092305, 93.05113791807858092 ) ) ;
#8322=CARTESIAN_POINT ( 'NONE',  ( 6.220909254589681581, 198.5229672870052582, 46.44886208192141908 ) ) ;
#8325=CARTESIAN_POINT ( 'NONE',  ( -7.456977232089471386, 217.1783343296987709, 53.94886208192144039 ) ) ;
#8332=CARTESIAN_POINT ( 'NONE',  ( 4.102348501002488490, 207.3577873115561943, -8.835681806194324750 ) ) ;
#8333=CARTESIAN_POINT ( 'NONE',  ( 4.903702542908601636, 200.1653181626581102, 50.45113791807857240 ) ) ;
#8336=CARTESIAN_POINT ( 'NONE',  ( -8.062137200540822946, 201.0835637161416400, 35.19886208192143329 ) ) ;
#8342=CARTESIAN_POINT ( 'NONE',  ( -2.426778023690076225, 199.3768101843759553, 7.898862081921436129 ) ) ;
#8344=CARTESIAN_POINT ( 'NONE',  ( 10.01549611932653860, 210.2015048109876716, 52.85113791807854966 ) ) ;
#8346=CARTESIAN_POINT ( 'NONE',  ( 10.01549611932653860, 210.2015048109876716, 37.85113791807854966 ) ) ;
#8349=CARTESIAN_POINT ( 'NONE',  ( -7.984503880673422316, 204.3529502787951628, 95.34886208192143897 ) ) ;
#8353=CARTESIAN_POINT ( 'NONE',  ( 9.680171189290831535, 199.9079932115568852, 5.301137918078565825 ) ) ;
#8356=CARTESIAN_POINT ( 'NONE',  ( 9.984503880673470277, 203.7031108863295401, 68.15113791807857524 ) ) ;
#8357=CARTESIAN_POINT ( 'NONE',  ( 0.05014649552810506589, 217.5146222423826714, 31.25113791807857311 ) ) ;
#8360=CARTESIAN_POINT ( 'NONE',  ( 8.062137200540822946, 212.9164362838583315, 12.69886208192143506 ) ) ;
#8363=CARTESIAN_POINT ( 'NONE',  ( 9.736236675707914401, 214.0148392665762458, 34.70113791807856529 ) ) ;
#8365=CARTESIAN_POINT ( 'NONE',  ( -9.984503880673420539, 203.7031108863293980, 26.34886208192142831 ) ) ;
#8370=CARTESIAN_POINT ( 'NONE',  ( 6.220909254589536808, 215.4770327129947702, 79.55113791807855250 ) ) ;
#8378=CARTESIAN_POINT ( 'NONE',  ( 8.015496119326531499, 209.5516654185219636, 10.85113791807856565 ) ) ;
#8380=CARTESIAN_POINT ( 'NONE',  ( 3.662846001189864698, 218.4274158808046593, 102.3988620819214361 ) ) ;
#8382=ORIENTED_EDGE ( 'NONE', *, *, #24563, .T. ) ;
#8386=CARTESIAN_POINT ( 'NONE',  ( 8.118202686958138514, 201.1607312380088501, 76.29886208192144181 ) ) ;
#8388=CARTESIAN_POINT ( 'NONE',  ( 8.062137200540920645, 201.0835637161417822, 23.30113791807856671 ) ) ;
#8394=CARTESIAN_POINT ( 'NONE',  ( 3.044812012440130555, 197.4746971517856764, 89.60113791807857808 ) ) ;
#8398=CARTESIAN_POINT ( 'NONE',  ( -12.01549611932659722, 210.8513442034533227, 92.64886208192143613 ) ) ;
#8401=DIRECTION ( 'NONE',  ( 0.000000000000000000, 0.9949972439410068592, -0.09990237509589369735 ) ) ;
#8407=CARTESIAN_POINT ( 'NONE',  ( -10.00000000000000711, 206.9523078486584495, 92.49886208192144466 ) ) ;
#8408=CARTESIAN_POINT ( 'NONE',  ( 3.662846001189864698, 218.4274158808046593, 36.39886208192143613 ) ) ;
#8410=CARTESIAN_POINT ( 'NONE',  ( 10.00000000000000711, 206.9523078486586201, 50.00113791807856956 ) ) ;
#8412=CARTESIAN_POINT ( 'NONE',  ( 8.000000000000008882, 207.0476921513415220, 3.998862081921434442 ) ) ;
#8415=CARTESIAN_POINT ( 'NONE',  ( 8.015496119326595448, 204.4483345814782638, 88.14886208192143613 ) ) ;
#8416=CARTESIAN_POINT ( 'NONE',  ( 4.984841277089725686, 213.7757310962907411, 28.55113791807857027 ) ) ;
#8422=CARTESIAN_POINT ( 'NONE',  ( -2.426778023690262742, 214.6231898156240163, 100.1011379180785781 ) ) ;
#8425=CARTESIAN_POINT ( 'NONE',  ( -2.426778023690076225, 199.3768101843759553, 73.89886208192143613 ) ) ;
#8428=CARTESIAN_POINT ( 'NONE',  ( 3.135527875058820690, 216.4958274776887492, 10.40113791807856636 ) ) ;
#8433=CARTESIAN_POINT ( 'NONE',  ( 9.736236675707914401, 214.0148392665762458, 79.70113791807857240 ) ) ;
#8435=CARTESIAN_POINT ( 'NONE',  ( -9.984503880673475606, 210.2968891136704315, 99.65113791807856103 ) ) ;
#8438=CARTESIAN_POINT ( 'NONE',  ( -12.00000000000000711, 206.9523078486584780, 62.49886208192143044 ) ) ;
#8439=CARTESIAN_POINT ( 'NONE',  ( -10.00000000000000711, 206.9523078486584495, 65.49886208192143044 ) ) ;
#8440=CARTESIAN_POINT ( 'NONE',  ( -9.736236675707914401, 199.9851607334237542, 102.2011379180785866 ) ) ;
#8442=CARTESIAN_POINT ( 'NONE',  ( -10.01549611932653860, 203.7984951890123284, 15.35113791807856565 ) ) ;
#8443=CARTESIAN_POINT ( 'NONE',  ( -10.00000000000000711, 206.9523078486584495, 74.49886208192144466 ) ) ;
#8445=CARTESIAN_POINT ( 'NONE',  ( -8.118202686958039038, 201.1607312380087080, 102.2011379180785866 ) ) ;
#8448=CARTESIAN_POINT ( 'NONE',  ( 2.426778023690075337, 214.6231898156240447, 57.39886208192144323 ) ) ;
#8456=CARTESIAN_POINT ( 'NONE',  ( -4.984841277089726574, 200.2242689037092305, 69.05113791807856671 ) ) ;
#8458=CARTESIAN_POINT ( 'NONE',  ( -9.790104562688519252, 205.9634215358804852, 104.4517247136924709 ) ) ;
#8461=CARTESIAN_POINT ( 'NONE',  ( 7.984503880673422316, 209.6470497212048372, 48.84886208192143897 ) ) ;
#8462=CARTESIAN_POINT ( 'NONE',  ( -8.062137200540920645, 212.9164362838581894, 81.80113791807858092 ) ) ;
#8463=CARTESIAN_POINT ( 'NONE',  ( -6.220909254589537696, 198.5229672870051161, 63.05113791807858092 ) ) ;
#8465=CARTESIAN_POINT ( 'NONE',  ( 2.517493886308900919, 214.5937144450984420, 22.40113791807856813 ) ) ;
#8469=CARTESIAN_POINT ( 'NONE',  ( -9.680171189290831535, 214.0920067884431148, 48.80113791807857382 ) ) ;
#8470=CARTESIAN_POINT ( 'NONE',  ( -6.220909254589537696, 198.5229672870051161, 99.05113791807858092 ) ) ;
#8471=CARTESIAN_POINT ( 'NONE',  ( 6.139770520408367460, 198.4640165459539389, 68.45113791807858661 ) ) ;
#8472=CARTESIAN_POINT ( 'NONE',  ( -7.375838497908014268, 196.7627149292498530, 29.04886208192143471 ) ) ;
#8473=CARTESIAN_POINT ( 'NONE',  ( 10.00000000000000711, 207.0476921513415220, 42.99886208192143044 ) ) ;
#8475=CARTESIAN_POINT ( 'NONE',  ( 12.01549611932652972, 210.8513442034534933, 73.85113791807857808 ) ) ;
#8476=CARTESIAN_POINT ( 'NONE',  ( 7.984503880673485376, 204.3529502787953902, 89.15113791807856103 ) ) ;
#8478=CARTESIAN_POINT ( 'NONE',  ( 9.984503880673420539, 210.2968891136705167, 45.84886208192141765 ) ) ;
#8481=CARTESIAN_POINT ( 'NONE',  ( -3.753561863808878130, 218.3979405102790281, 60.09886208192143897 ) ) ;
#8483=CARTESIAN_POINT ( 'NONE',  ( 6.444103211790928043, 211.7408657792734061, 33.69886208192144039 ) ) ;
#8484=ORIENTED_EDGE ( 'NONE', *, *, #29774, .F. ) ;
#8490=CARTESIAN_POINT ( 'NONE',  ( 0.05014649552807626948, 215.4116977939061144, 49.25113791807856956 ) ) ;
#8492=CARTESIAN_POINT ( 'NONE',  ( 6.139770520408223575, 215.5359834540460611, 33.54886208192143471 ) ) ;
#8498=CARTESIAN_POINT ( 'NONE',  ( 2.517493886309087436, 199.4062855549015865, 19.59886208192143897 ) ) ;
#8499=CARTESIAN_POINT ( 'NONE',  ( -9.984503880673473830, 210.2968891136704315, 48.65113791807858235 ) ) ;
#8501=CARTESIAN_POINT ( 'NONE',  ( -10.01549611932653860, 203.7984951890123284, 36.35113791807857098 ) ) ;
#8503=CARTESIAN_POINT ( 'NONE',  ( 7.984503880673422316, 209.6470497212048372, 87.84886208192142476 ) ) ;
#8506=CARTESIAN_POINT ( 'NONE',  ( -3.662846001190052991, 218.4274158808045740, 19.10113791807856742 ) ) ;
#8510=CARTESIAN_POINT ( 'NONE',  ( 10.01549611932653860, 210.2015048109876716, 70.85113791807854966 ) ) ;
#8511=CARTESIAN_POINT ( 'NONE',  ( -0.05014649552810635652, 196.4853777576173002, 38.75113791807856956 ) ) ;
#8516=CARTESIAN_POINT ( 'NONE',  ( -6.139770520408224463, 198.4640165459539105, 11.04886208192143648 ) ) ;
#8519=CARTESIAN_POINT ( 'NONE',  ( 9.680171189290831535, 199.9079932115568852, 47.30113791807856671 ) ) ;
#8521=CARTESIAN_POINT ( 'NONE',  ( -10.00000000000000711, 206.9523078486584495, 20.49886208192143755 ) ) ;
#8525=CARTESIAN_POINT ( 'NONE',  ( 0.05014649552810505201, 217.5146222423826714, 76.25113791807855534 ) ) ;
#8530=CARTESIAN_POINT ( 'NONE',  ( -8.015496119326531499, 204.4483345814780364, 21.35113791807856742 ) ) ;
#8533=CARTESIAN_POINT ( 'NONE',  ( 6.220909254589681581, 198.5229672870052582, 1.448862081921434397 ) ) ;
#8541=CARTESIAN_POINT ( 'NONE',  ( -8.118202686958138514, 212.8392687619910930, 89.79886208192144181 ) ) ;
#8543=CARTESIAN_POINT ( 'NONE',  ( 0.05014649552810505201, 217.5146222423826714, 19.25113791807856600 ) ) ;
#8547=CARTESIAN_POINT ( 'NONE',  ( -12.00000000000000711, 206.9523078486584780, 80.49886208192144466 ) ) ;
#8552=CARTESIAN_POINT ( 'NONE',  ( -3.044812012440131443, 216.5253028482142952, 97.10113791807857808 ) ) ;
#8556=CARTESIAN_POINT ( 'NONE',  ( 0.05014649552810505201, 217.5146222423826714, 40.25113791807856956 ) ) ;
#8562=CARTESIAN_POINT ( 'NONE',  ( -3.753561863808691168, 195.6020594897209435, 20.90113791807856813 ) ) ;
#8564=ADVANCED_FACE ( 'NONE', ( #29302 ), #28969, .T. ) ;
#8569=CARTESIAN_POINT ( 'NONE',  ( -3.044812012439970683, 197.4746971517856196, 91.89886208192143613 ) ) ;
#8572=CARTESIAN_POINT ( 'NONE',  ( 9.736236675708031640, 199.9851607334238963, 37.29886208192143471 ) ) ;
#8573=CARTESIAN_POINT ( 'NONE',  ( -10.33420400187145027, 207.8560350444080598, 102.5922263069843581 ) ) ;
#8574=CARTESIAN_POINT ( 'NONE',  ( -6.220909254589537696, 198.5229672870051161, 48.05113791807858092 ) ) ;
#8576=CARTESIAN_POINT ( 'NONE',  ( 8.015496119326595448, 204.4483345814782638, 13.14886208192143613 ) ) ;
#8579=CARTESIAN_POINT ( 'NONE',  ( 6.500168698208244500, 202.3363017425938324, 97.29886208192142760 ) ) ;
#8580=CARTESIAN_POINT ( 'NONE',  ( -6.500168698208129925, 202.3363017425936050, 39.20113791807857240 ) ) ;
#8584=CARTESIAN_POINT ( 'NONE',  ( -6.220909254589682469, 215.4770327129946850, 53.94886208192144039 ) ) ;
#8587=CARTESIAN_POINT ( 'NONE',  ( -7.984503880673488041, 209.6470497212046098, 96.65113791807858945 ) ) ;
#8590=CARTESIAN_POINT ( 'NONE',  ( -2.426778023690076225, 199.3768101843759553, 70.89886208192143613 ) ) ;
#8594=CARTESIAN_POINT ( 'NONE',  ( -10.00000000000000711, 207.0476921513413515, 6.501137918078566003 ) ) ;
#8598=CARTESIAN_POINT ( 'NONE',  ( 9.736236675707914401, 214.0148392665762458, 76.70113791807857240 ) ) ;
#8599=CARTESIAN_POINT ( 'NONE',  ( -10.01549611932653860, 203.7984951890123000, 93.35113791807857808 ) ) ;
#8602=CARTESIAN_POINT ( 'NONE',  ( -9.984503880673420539, 203.7031108863293980, 5.348862081921433642 ) ) ;
#8603=CARTESIAN_POINT ( 'NONE',  ( -7.456977232089471386, 217.1783343296987709, 62.94886208192144039 ) ) ;
#8604=CARTESIAN_POINT ( 'NONE',  ( -3.135527875058982783, 216.4958274776886924, 63.09886208192143187 ) ) ;
#8605=CARTESIAN_POINT ( 'NONE',  ( -0.05014649552828442242, 219.6175466908591716, 3.248862081921433997 ) ) ;
#8608=CARTESIAN_POINT ( 'NONE',  ( 6.139770520408368348, 198.4640165459539674, 26.45113791807856884 ) ) ;
#8609=CARTESIAN_POINT ( 'NONE',  ( 10.00000000000000711, 207.0476921513415220, 87.99886208192144466 ) ) ;
#8615=CARTESIAN_POINT ( 'NONE',  ( 6.500168698208244500, 202.3363017425938324, 61.29886208192144892 ) ) ;
#8622=CARTESIAN_POINT ( 'NONE',  ( -7.984503880673488041, 209.6470497212046098, 66.65113791807856103 ) ) ;
#8623=CARTESIAN_POINT ( 'NONE',  ( 10.00000000000000888, 207.0000000000002842, 5.551115123125782702E-14 ) ) ;
#8624=CARTESIAN_POINT ( 'NONE',  ( -9.139829196538601153, 206.4498403098741335, 104.0238431579207088 ) ) ;
#8626=CARTESIAN_POINT ( 'NONE',  ( -4.903702542908436435, 200.1653181626580249, 41.04886208192144181 ) ) ;
#8628=CARTESIAN_POINT ( 'NONE',  ( -0.05014649552810635652, 196.4853777576173002, 77.75113791807856956 ) ) ;
#8629=CARTESIAN_POINT ( 'NONE',  ( 8.118202686958039038, 212.8392687619912635, 64.70113791807857240 ) ) ;
#8632=CARTESIAN_POINT ( 'NONE',  ( 8.640141755188686545, 206.6086104956403915, 111.6972426105882477 ) ) ;
#8633=CARTESIAN_POINT ( 'NONE',  ( 6.444103211791042618, 202.2591342207267644, 20.30113791807857027 ) ) ;
#8637=CARTESIAN_POINT ( 'NONE',  ( 12.01549611932652972, 210.8513442034534933, 49.85113791807857808 ) ) ;
#8639=CARTESIAN_POINT ( 'NONE',  ( -10.01549611932653860, 203.7984951890123284, 96.35113791807853545 ) ) ;
#8641=CARTESIAN_POINT ( 'NONE',  ( -0.05014649552810635652, 196.4853777576173002, 68.75113791807855534 ) ) ;
#8643=CARTESIAN_POINT ( 'NONE',  ( 12.01549611932659367, 203.1486557965466773, 34.14886208192143613 ) ) ;
#8644=CARTESIAN_POINT ( 'NONE',  ( 9.984503880673420539, 210.2968891136705736, 36.84886208192143187 ) ) ;
#8646=CARTESIAN_POINT ( 'NONE',  ( 0.05014649552807549926, 219.6175466908591716, 76.25113791807856956 ) ) ;
#8647=CARTESIAN_POINT ( 'NONE',  ( -8.000000000000008882, 207.0476921513413515, 102.5011379180785696 ) ) ;
#8648=CARTESIAN_POINT ( 'NONE',  ( -6.139770520408224463, 198.4640165459539389, 53.04886208192142050 ) ) ;
#8651=CARTESIAN_POINT ( 'NONE',  ( -11.98450388067341876, 203.0532714938636047, 62.34886208192143187 ) ) ;
#8653=CARTESIAN_POINT ( 'NONE',  ( 4.903702542908435547, 213.8346818373419751, 30.54886208192144181 ) ) ;
#8657=CARTESIAN_POINT ( 'NONE',  ( -9.736236675707914401, 199.9851607334237542, 72.20113791807857240 ) ) ;
#8659=CARTESIAN_POINT ( 'NONE',  ( 6.444103211791042618, 202.2591342207267644, 47.30113791807858092 ) ) ;
#8661=CARTESIAN_POINT ( 'NONE',  ( -6.220909254589682469, 215.4770327129946850, 35.94886208192141908 ) ) ;
#8667=CARTESIAN_POINT ( 'NONE',  ( 7.984503880673422316, 209.6470497212048372, 12.84886208192143719 ) ) ;
#8668=CARTESIAN_POINT ( 'NONE',  ( 9.984503880673470277, 203.7031108863295401, 53.15113791807857524 ) ) ;
#8670=CARTESIAN_POINT ( 'NONE',  ( 10.00000000000000711, 206.9523078486586201, 41.00113791807856956 ) ) ;
#8673=CARTESIAN_POINT ( 'NONE',  ( -6.500168698208244500, 211.6636982574061676, 101.7988620819214560 ) ) ;
#8677=CARTESIAN_POINT ( 'NONE',  ( 7.375838497908181246, 196.7627149292499666, 17.45113791807856174 ) ) ;
#8680=CARTESIAN_POINT ( 'NONE',  ( 0.05014649552810505201, 217.5146222423826714, 64.25113791807856956 ) ) ;
#8682=CARTESIAN_POINT ( 'NONE',  ( 0.05014649552810506589, 217.5146222423826714, 37.25113791807856956 ) ) ;
#8685=CARTESIAN_POINT ( 'NONE',  ( 12.00000000000000711, 207.0476921513415220, 3.998862081921433997 ) ) ;
#8686=CARTESIAN_POINT ( 'NONE',  ( 0.05014649552828275014, 196.4853777576173002, 10.74886208192143577 ) ) ;
#8689=CARTESIAN_POINT ( 'NONE',  ( -3.753561863808691168, 195.6020594897209435, 44.90113791807856813 ) ) ;
#8690=CARTESIAN_POINT ( 'NONE',  ( 6.500168698208129925, 211.6636982574063381, 73.70113791807857240 ) ) ;
#8692=CARTESIAN_POINT ( 'NONE',  ( -8.062137200540822946, 201.0835637161416400, 23.19886208192143684 ) ) ;
#8696=CARTESIAN_POINT ( 'NONE',  ( -6.139770520408369237, 215.5359834540460042, 84.95113791807858661 ) ) ;
#8701=CARTESIAN_POINT ( 'NONE',  ( 4.903702542908601636, 200.1653181626581102, 20.45113791807856529 ) ) ;
#8705=CARTESIAN_POINT ( 'NONE',  ( -3.135527875058982783, 216.4958274776886924, 6.098862081921434530 ) ) ;
#8712=CARTESIAN_POINT ( 'NONE',  ( -6.139770520408224463, 198.4640165459539389, 86.04886208192144181 ) ) ;
#8713=EDGE_CURVE ( 'NONE', #11826, #6436, #4894, .T. ) ;
#8715=CARTESIAN_POINT ( 'NONE',  ( -3.135527875058821579, 197.5041725223112223, 26.90113791807856813 ) ) ;
#8717=CARTESIAN_POINT ( 'NONE',  ( 12.00000000000000711, 207.0476921513415220, 78.99886208192144466 ) ) ;
#8721=CARTESIAN_POINT ( 'NONE',  ( 8.118202686958039038, 212.8392687619912635, 94.70113791807857240 ) ) ;
#8724=CARTESIAN_POINT ( 'NONE',  ( -6.139770520408369237, 215.5359834540460042, 36.95113791807857240 ) ) ;
#8727=ORIENTED_EDGE ( 'NONE', *, *, #24292, .F. ) ;
#8729=CARTESIAN_POINT ( 'NONE',  ( -12.01549611932652972, 203.1486557965464499, 15.35113791807856387 ) ) ;
#8733=CARTESIAN_POINT ( 'NONE',  ( 0.05014649552828288198, 194.3824533091408000, 28.74886208192144110 ) ) ;
#8735=CARTESIAN_POINT ( 'NONE',  ( 6.139770520408368348, 198.4640165459539674, 50.45113791807857240 ) ) ;
#8737=CARTESIAN_POINT ( 'NONE',  ( -6.444103211790928043, 202.2591342207265939, 14.19886208192143684 ) ) ;
#8743=CARTESIAN_POINT ( 'NONE',  ( -0.05014649552828365914, 215.4116977939061144, 96.24886208192144466 ) ) ;
#8745=CARTESIAN_POINT ( 'NONE',  ( -6.444103211791042618, 211.7408657792732356, 42.80113791807857382 ) ) ;
#8746=DIRECTION ( 'NONE',  ( -0.2649168722799636333, 0.9642688156137663169, -0.002168413296789690158 ) ) ;
#8749=CARTESIAN_POINT ( 'NONE',  ( -0.05014649552828403384, 217.5146222423826714, 60.24886208192142334 ) ) ;
#8753=CARTESIAN_POINT ( 'NONE',  ( 7.984503880673485376, 204.3529502787953902, 95.15113791807856103 ) ) ;
#8755=CARTESIAN_POINT ( 'NONE',  ( -6.500168698208244500, 211.6636982574061676, 71.79886208192142760 ) ) ;
#8758=CARTESIAN_POINT ( 'NONE',  ( 9.984503880673473830, 203.7031108863295401, 14.15113791807856636 ) ) ;
#8764=CARTESIAN_POINT ( 'NONE',  ( -9.680171189290831535, 214.0920067884431148, 75.80113791807858092 ) ) ;
#8765=CARTESIAN_POINT ( 'NONE',  ( -6.139770520408368348, 215.5359834540460042, 96.95113791807857240 ) ) ;
#8768=CARTESIAN_POINT ( 'NONE',  ( -8.062137200540822946, 201.0835637161416400, 2.198862081921434175 ) ) ;
#8769=CARTESIAN_POINT ( 'NONE',  ( -7.456977232089471386, 217.1783343296987709, 65.94886208192144750 ) ) ;
#8770=CARTESIAN_POINT ( 'NONE',  ( 10.00000000000000711, 207.0476921513415220, 66.99886208192143044 ) ) ;
#8771=CARTESIAN_POINT ( 'NONE',  ( -7.456977232089471386, 217.1783343296987709, 5.948862081921435063 ) ) ;
#8773=CARTESIAN_POINT ( 'NONE',  ( -10.01549611932653860, 203.7984951890123284, 18.35113791807856742 ) ) ;
#8774=CARTESIAN_POINT ( 'NONE',  ( 8.118202686958138514, 201.1607312380088501, 88.29886208192142760 ) ) ;
#8779=CARTESIAN_POINT ( 'NONE',  ( 4.984841277089891776, 200.2242689037093726, 73.44886208192143329 ) ) ;
#8786=CARTESIAN_POINT ( 'NONE',  ( -6.444103211791042618, 211.7408657792732356, 66.80113791807858092 ) ) ;
#8790=CARTESIAN_POINT ( 'NONE',  ( -2.426778023690076225, 199.3768101843759553, 40.89886208192144323 ) ) ;
#8791=CARTESIAN_POINT ( 'NONE',  ( 10.01549611932653860, 210.2015048109876716, 88.85113791807857808 ) ) ;
#8792=CARTESIAN_POINT ( 'NONE',  ( 8.118202686958039038, 212.8392687619912635, 67.70113791807858661 ) ) ;
#8794=CARTESIAN_POINT ( 'NONE',  ( -2.517493886308901807, 199.4062855549015012, 20.90113791807856813 ) ) ;
#8798=CARTESIAN_POINT ( 'NONE',  ( 7.375838497908181246, 196.7627149292499666, 44.45113791807857240 ) ) ;
#8800=CARTESIAN_POINT ( 'NONE',  ( 9.984503880673470277, 203.7031108863295401, 98.15113791807858945 ) ) ;
#8801=CARTESIAN_POINT ( 'NONE',  ( 10.00000000000000711, 206.9523078486586201, 65.00113791807856956 ) ) ;
#8802=CARTESIAN_POINT ( 'NONE',  ( -0.05014649552828442242, 219.6175466908591716, 33.24886208192143755 ) ) ;
#8803=CARTESIAN_POINT ( 'NONE',  ( 10.01549611932659367, 203.7984951890124421, 34.14886208192143613 ) ) ;
#8805=CARTESIAN_POINT ( 'NONE',  ( -9.680171189290831535, 214.0920067884431148, 72.80113791807858092 ) ) ;
#8806=CARTESIAN_POINT ( 'NONE',  ( -6.500168698208129925, 202.3363017425936050, 99.20113791807858661 ) ) ;
#8807=CARTESIAN_POINT ( 'NONE',  ( -3.044812012439970683, 197.4746971517856196, 61.89886208192143613 ) ) ;
#8809=CARTESIAN_POINT ( 'NONE',  ( 12.01549611932659367, 203.1486557965466773, 61.14886208192143613 ) ) ;
#8812=CARTESIAN_POINT ( 'NONE',  ( 0.05014649552828262524, 198.5883022060938572, 43.74886208192144466 ) ) ;
#8817=CARTESIAN_POINT ( 'NONE',  ( -4.903702542908602524, 213.8346818373418898, 54.95113791807857240 ) ) ;
#8819=CARTESIAN_POINT ( 'NONE',  ( -8.062137200540822946, 201.0835637161416400, 29.19886208192143684 ) ) ;
#8827=CARTESIAN_POINT ( 'NONE',  ( -4.903702542908436435, 200.1653181626580249, 20.04886208192143471 ) ) ;
#8828=CARTESIAN_POINT ( 'NONE',  ( 9.984503880673470277, 203.7031108863295401, 47.15113791807857524 ) ) ;
#8829=CARTESIAN_POINT ( 'NONE',  ( 10.00000000000000711, 206.9523078486586201, 35.00113791807856956 ) ) ;
#8832=CARTESIAN_POINT ( 'NONE',  ( 7.984503880673485376, 204.3529502787953902, -0.8488620819214343083 ) ) ;
#8837=CARTESIAN_POINT ( 'NONE',  ( -11.98450388067348804, 210.9467285061362247, 15.65113791807856636 ) ) ;
#8841=CARTESIAN_POINT ( 'NONE',  ( 10.00000000000000711, 206.9523078486586201, 62.00113791807856956 ) ) ;
#8842=CARTESIAN_POINT ( 'NONE',  ( -3.044812012440131443, 216.5253028482142952, 43.10113791807857808 ) ) ;
#8845=CARTESIAN_POINT ( 'NONE',  ( 7.375838497908012492, 217.2372850707501186, 6.548862081921433820 ) ) ;
#8846=CARTESIAN_POINT ( 'NONE',  ( -0.05014649552828402690, 217.5146222423826714, 6.248862081921433997 ) ) ;
#8849=CARTESIAN_POINT ( 'NONE',  ( 11.98450388067348271, 203.0532714938637753, 50.15113791807857524 ) ) ;
#8850=CARTESIAN_POINT ( 'NONE',  ( 7.984503880673485376, 204.3529502787953902, 65.15113791807856103 ) ) ;
#8852=CARTESIAN_POINT ( 'NONE',  ( 8.062137200540822946, 212.9164362838583315, 33.69886208192143329 ) ) ;
#8855=CARTESIAN_POINT ( 'NONE',  ( 6.139770520408368348, 198.4640165459539674, 77.45113791807854398 ) ) ;
#8861=CARTESIAN_POINT ( 'NONE',  ( -8.015496119326531499, 204.4483345814780364, 24.35113791807856742 ) ) ;
#8865=CARTESIAN_POINT ( 'NONE',  ( 6.220909254589681581, 198.5229672870052582, 7.448862081921433287 ) ) ;
#8872=CARTESIAN_POINT ( 'NONE',  ( 0.000000000000000000, 0.000000000000000000, 0.000000000000000000 ) ) ;
#8874=CARTESIAN_POINT ( 'NONE',  ( 6.220909254589681581, 198.5229672870052582, 88.44886208192144750 ) ) ;
#8876=CARTESIAN_POINT ( 'NONE',  ( 6.220909254589536808, 215.4770327129947702, 22.55113791807856671 ) ) ;
#8878=CARTESIAN_POINT ( 'NONE',  ( -12.01549611932659722, 210.8513442034533227, 80.64886208192145034 ) ) ;
#8882=DIRECTION ( 'NONE',  ( -0.5526942671207060176, -0.1536855300543007452, -0.8190908404712106128 ) ) ;
#8884=CARTESIAN_POINT ( 'NONE',  ( -8.062137200540920645, 212.9164362838581894, 90.80113791807858092 ) ) ;
#8887=CARTESIAN_POINT ( 'NONE',  ( -3.044812012440131443, 216.5253028482142952, 37.10113791807857098 ) ) ;
#8892=CARTESIAN_POINT ( 'NONE',  ( -3.662846001190052991, 218.4274158808045740, 22.10113791807856742 ) ) ;
#8898=CARTESIAN_POINT ( 'NONE',  ( -7.375838497908014268, 196.7627149292498530, 32.04886208192143471 ) ) ;
#8900=CARTESIAN_POINT ( 'NONE',  ( 8.118202686958039038, 212.8392687619912635, 55.70113791807857950 ) ) ;
#8904=CARTESIAN_POINT ( 'NONE',  ( 2.517493886309087436, 199.4062855549015865, 16.59886208192143897 ) ) ;
#8908=CARTESIAN_POINT ( 'NONE',  ( -8.015496119326597224, 209.5516654185217362, 98.64886208192146455 ) ) ;
#8911=CARTESIAN_POINT ( 'NONE',  ( -6.444103211791042618, 211.7408657792732356, 39.80113791807857382 ) ) ;
#8917=CARTESIAN_POINT ( 'NONE',  ( 6.139770520408223575, 215.5359834540460611, 63.54886208192144181 ) ) ;
#8918=CIRCLE ( 'NONE', #3465, 0.9999999999999941158 ) ;
#8921=CARTESIAN_POINT ( 'NONE',  ( -4.903702542908602524, 213.8346818373418898, 93.95113791807857240 ) ) ;
#8924=CARTESIAN_POINT ( 'NONE',  ( -4.903702542908436435, 200.1653181626580249, 71.04886208192142760 ) ) ;
#8930=CARTESIAN_POINT ( 'NONE',  ( -0.05014649552810635652, 196.4853777576173002, 17.75113791807856245 ) ) ;
#8934=CARTESIAN_POINT ( 'NONE',  ( -12.01549611932652972, 203.1486557965464499, 81.35113791807857808 ) ) ;
#8936=CARTESIAN_POINT ( 'NONE',  ( -0.05014649552810635652, 196.4853777576173002, 92.75113791807858377 ) ) ;
#8939=CARTESIAN_POINT ( 'NONE',  ( 10.01549611932659545, 203.7984951890123853, 1.148862081921433909 ) ) ;
#8940=CARTESIAN_POINT ( 'NONE',  ( 0.05014649552828288198, 194.3824533091408000, 58.74886208192142334 ) ) ;
#8941=CARTESIAN_POINT ( 'NONE',  ( 6.220909254589680693, 198.5229672870052582, 73.44886208192141908 ) ) ;
#8942=CARTESIAN_POINT ( 'NONE',  ( 12.00000000000000711, 207.0476921513415220, 0.9988620819214339974 ) ) ;
#8944=CARTESIAN_POINT ( 'NONE',  ( 9.984503880673470277, 203.7031108863295401, 26.15113791807856813 ) ) ;
#8946=CARTESIAN_POINT ( 'NONE',  ( -10.00000000000000711, 206.9523078486584495, 92.49886208192144466 ) ) ;
#8951=CARTESIAN_POINT ( 'NONE',  ( -0.05014649552828365914, 215.4116977939061144, 69.24886208192143044 ) ) ;
#8957=CARTESIAN_POINT ( 'NONE',  ( -6.500168698208129925, 202.3363017425936050, 72.20113791807857240 ) ) ;
#8961=CARTESIAN_POINT ( 'NONE',  ( 4.903702542908435547, 213.8346818373419751, 39.54886208192143471 ) ) ;
#8962=CARTESIAN_POINT ( 'NONE',  ( 6.220909254589536808, 215.4770327129947702, 85.55113791807858092 ) ) ;
#8964=CARTESIAN_POINT ( 'NONE',  ( -3.044812012440131443, 216.5253028482142952, 64.10113791807857808 ) ) ;
#8970=CARTESIAN_POINT ( 'NONE',  ( 3.662846001190051659, 195.5725841191953691, 44.60113791807857098 ) ) ;
#8972=ADVANCED_FACE ( 'NONE', ( #15930 ), #23924, .T. ) ;
#8974=CARTESIAN_POINT ( 'NONE',  ( -8.118202686958039038, 201.1607312380087080, 96.20113791807857240 ) ) ;
#8977=CARTESIAN_POINT ( 'NONE',  ( -6.139770520408368348, 215.5359834540460042, 69.95113791807858661 ) ) ;
#8978=CARTESIAN_POINT ( 'NONE',  ( 7.456977232089471386, 196.8216656703012006, 37.44886208192143329 ) ) ;
#8979=CARTESIAN_POINT ( 'NONE',  ( -0.05014649552828402690, 217.5146222423826714, 42.24886208192143044 ) ) ;
#8981=CARTESIAN_POINT ( 'NONE',  ( -9.680171189290831535, 214.0920067884431148, 75.80113791807858092 ) ) ;
#8982=CARTESIAN_POINT ( 'NONE',  ( 0.05014649552807626948, 215.4116977939061144, 97.25113791807856956 ) ) ;
#8983=CARTESIAN_POINT ( 'NONE',  ( -6.220909254589682469, 215.4770327129946850, 62.94886208192143329 ) ) ;
#8986=CARTESIAN_POINT ( 'NONE',  ( 7.456977232089471386, 196.8216656703012006, 58.44886208192144039 ) ) ;
#8989=CARTESIAN_POINT ( 'NONE',  ( -6.444103211790928043, 202.2591342207265939, 44.19886208192144750 ) ) ;
#8994=CARTESIAN_POINT ( 'NONE',  ( -4.984841277089726574, 200.2242689037092305, 48.05113791807858092 ) ) ;
#8996=CARTESIAN_POINT ( 'NONE',  ( -0.05014649552828403384, 217.5146222423826714, 30.24886208192142689 ) ) ;
#9002=CARTESIAN_POINT ( 'NONE',  ( -2.426778023690076225, 199.3768101843759553, 19.89886208192143613 ) ) ;
#9003=CARTESIAN_POINT ( 'NONE',  ( 10.00000000000000711, 206.9523078486586201, 59.00113791807857666 ) ) ;
#9005=CARTESIAN_POINT ( 'NONE',  ( 9.984503880673470277, 203.7031108863295401, 38.15113791807856813 ) ) ;
#9008=CARTESIAN_POINT ( 'NONE',  ( -2.517493886308901807, 199.4062855549015012, -0.09886208192143407236 ) ) ;
#9012=CARTESIAN_POINT ( 'NONE',  ( -9.736236675707914401, 199.9851607334237542, 18.20113791807856529 ) ) ;
#9014=CARTESIAN_POINT ( 'NONE',  ( -3.135527875058821579, 197.5041725223112223, 65.90113791807857524 ) ) ;
#9015=CARTESIAN_POINT ( 'NONE',  ( 0.05014649552810506589, 217.5146222423826714, 40.25113791807856956 ) ) ;
#9019=CARTESIAN_POINT ( 'NONE',  ( -7.456977232089304408, 196.8216656703010301, 102.0511379180785809 ) ) ;
#9020=CARTESIAN_POINT ( 'NONE',  ( -8.062137200540822946, 201.0835637161416400, 5.198862081921435063 ) ) ;
#9023=CARTESIAN_POINT ( 'NONE',  ( 3.662846001190051659, 195.5725841191953691, 44.60113791807857098 ) ) ;
#9024=CARTESIAN_POINT ( 'NONE',  ( 8.015496119326531499, 209.5516654185219636, 70.85113791807857808 ) ) ;
#9025=CARTESIAN_POINT ( 'NONE',  ( 10.00000000000000711, 207.0476921513415220, 30.99886208192143755 ) ) ;
#9028=CARTESIAN_POINT ( 'NONE',  ( 3.135527875058820690, 216.4958274776887492, 79.40113791807857524 ) ) ;
#9033=CARTESIAN_POINT ( 'NONE',  ( -6.444103211791042618, 211.7408657792732356, 21.80113791807856671 ) ) ;
#9035=CARTESIAN_POINT ( 'NONE',  ( -7.375838497908014268, 196.7627149292498530, 104.0488620819214560 ) ) ;
#9039=CARTESIAN_POINT ( 'NONE',  ( 4.903702542908601636, 200.1653181626581102, 47.45113791807857950 ) ) ;
#9042=CARTESIAN_POINT ( 'NONE',  ( 6.220909254589681581, 198.5229672870052582, 94.44886208192140487 ) ) ;
#9044=CARTESIAN_POINT ( 'NONE',  ( 9.984503880673470277, 203.7031108863295401, 29.15113791807856103 ) ) ;
#9046=CARTESIAN_POINT ( 'NONE',  ( -9.680171189290716072, 199.9079932115567146, 80.19886208192143329 ) ) ;
#9051=CARTESIAN_POINT ( 'NONE',  ( 9.984503880673470277, 203.7031108863295401, 98.15113791807858945 ) ) ;
#9054=CARTESIAN_POINT ( 'NONE',  ( -10.01549611932653860, 203.7984951890123284, 36.35113791807857098 ) ) ;
#9060=CARTESIAN_POINT ( 'NONE',  ( -3.753561863808691168, 195.6020594897209435, 17.90113791807856458 ) ) ;
#9065=CARTESIAN_POINT ( 'NONE',  ( 7.375838497908012492, 217.2372850707501186, 45.54886208192143471 ) ) ;
#9066=CARTESIAN_POINT ( 'NONE',  ( -0.05014649552810635652, 196.4853777576173002, 5.751137918078563338 ) ) ;
#9067=CARTESIAN_POINT ( 'NONE',  ( -9.984503880673473830, 210.2968891136704315, 51.65113791807855392 ) ) ;
#9068=CARTESIAN_POINT ( 'NONE',  ( -2.517493886309087880, 214.5937144450984135, 12.09886208192143364 ) ) ;
#9073=CARTESIAN_POINT ( 'NONE',  ( 6.444103211790928043, 211.7408657792734061, 96.69886208192144750 ) ) ;
#9075=CARTESIAN_POINT ( 'NONE',  ( -2.517493886308901807, 199.4062855549015012, 44.90113791807856813 ) ) ;
#9080=DIRECTION ( 'NONE',  ( 0.000000000000000000, 0.9988620819214357738, 0.04769215134144196705 ) ) ;
#9081=CARTESIAN_POINT ( 'NONE',  ( -8.118202686958138514, 212.8392687619910930, 59.79886208192143471 ) ) ;
#9084=CARTESIAN_POINT ( 'NONE',  ( -6.444103211791042618, 211.7408657792732356, 99.80113791807858092 ) ) ;
#9087=CARTESIAN_POINT ( 'NONE',  ( 8.015496119326595448, 204.4483345814782638, 85.14886208192143613 ) ) ;
#9094=CARTESIAN_POINT ( 'NONE',  ( -0.05014649552810635652, 196.4853777576173002, 20.75113791807856245 ) ) ;
#9098=CARTESIAN_POINT ( 'NONE',  ( 7.456977232089302632, 217.1783343296989131, 88.55113791807858092 ) ) ;
#9103=EDGE_LOOP ( 'NONE', ( #31565, #15573, #22061, #31165, #11509, #17342 ) ) ;
#9104=CARTESIAN_POINT ( 'NONE',  ( 7.375838497908012492, 217.2372850707501186, 72.54886208192141339 ) ) ;
#9105=CARTESIAN_POINT ( 'NONE',  ( -8.118202686958138514, 212.8392687619910930, 80.79886208192144181 ) ) ;
#9106=CARTESIAN_POINT ( 'NONE',  ( -9.680171189290716072, 199.9079932115567146, 11.19886208192143506 ) ) ;
#9108=CARTESIAN_POINT ( 'NONE',  ( -6.220909254589537696, 198.5229672870051161, 21.05113791807855961 ) ) ;
#9109=CARTESIAN_POINT ( 'NONE',  ( -8.062137200540822946, 201.0835637161416400, 86.19886208192144750 ) ) ;
#9115=CARTESIAN_POINT ( 'NONE',  ( -8.015496119326597224, 209.5516654185217362, 68.64886208192142192 ) ) ;
#9125=CARTESIAN_POINT ( 'NONE',  ( 2.426778023690261410, 199.3768101843759837, 65.60113791807857808 ) ) ;
#9129=CARTESIAN_POINT ( 'NONE',  ( 7.984503880673422316, 209.6470497212048372, 54.84886208192144608 ) ) ;
#9130=EDGE_CURVE ( 'NONE', #13603, #11012, #25309, .T. ) ;
#9131=CARTESIAN_POINT ( 'NONE',  ( -10.01549611932653860, 203.7984951890123284, 75.35113791807853545 ) ) ;
#9137=CARTESIAN_POINT ( 'NONE',  ( 12.01549611932652972, 210.8513442034534933, 61.85113791807857098 ) ) ;
#9140=CARTESIAN_POINT ( 'NONE',  ( -12.01549611932652972, 203.1486557965464499, 3.351137918078566091 ) ) ;
#9141=CARTESIAN_POINT ( 'NONE',  ( -3.044812012440131443, 216.5253028482142952, 67.10113791807857808 ) ) ;
#9143=CARTESIAN_POINT ( 'NONE',  ( -3.662846001189865142, 195.5725841191952838, 34.89886208192143613 ) ) ;
#9144=CARTESIAN_POINT ( 'NONE',  ( -6.139770520408224463, 198.4640165459539105, 47.04886208192143471 ) ) ;
#9146=CARTESIAN_POINT ( 'NONE',  ( -0.05014649552807705357, 194.3824533091408000, 86.75113791807856956 ) ) ;
#9147=CARTESIAN_POINT ( 'NONE',  ( -0.05014649552807731031, 198.5883022060938572, 101.7511379180785696 ) ) ;
#9148=CARTESIAN_POINT ( 'NONE',  ( -3.135527875058982783, 216.4958274776886924, 60.09886208192143897 ) ) ;
#9152=CARTESIAN_POINT ( 'NONE',  ( -9.736236675708031640, 214.0148392665760753, 65.79886208192144181 ) ) ;
#9155=CARTESIAN_POINT ( 'NONE',  ( 4.984841277089891776, 200.2242689037093726, 46.44886208192144039 ) ) ;
#9160=CARTESIAN_POINT ( 'NONE',  ( 4.102348501002488490, 207.3577873115561943, -8.835681806194324750 ) ) ;
#9162=CARTESIAN_POINT ( 'NONE',  ( 4.903702542908601636, 200.1653181626581102, 59.45113791807857240 ) ) ;
#9167=CARTESIAN_POINT ( 'NONE',  ( -10.00000000000000711, 206.9523078486584495, 41.49886208192143044 ) ) ;
#9172=( NAMED_UNIT ( * ) SI_UNIT ( $, .STERADIAN. ) SOLID_ANGLE_UNIT ( ) );
#9175=CARTESIAN_POINT ( 'NONE',  ( 4.903702542908435547, 213.8346818373419751, 18.54886208192143116 ) ) ;
#9177=CARTESIAN_POINT ( 'NONE',  ( -10.01549611932653860, 203.7984951890123284, 63.35113791807857098 ) ) ;
#9178=CARTESIAN_POINT ( 'NONE',  ( -10.01549611932653860, 203.7984951890123284, 45.35113791807857808 ) ) ;
#9181=CARTESIAN_POINT ( 'NONE',  ( 3.044812012440130555, 197.4746971517856764, 17.60113791807856742 ) ) ;
#9182=CARTESIAN_POINT ( 'NONE',  ( 6.444103211790928043, 211.7408657792734061, 102.6988620819214475 ) ) ;
#9186=CARTESIAN_POINT ( 'NONE',  ( -7.456977232089304408, 196.8216656703010301, 15.05113791807856849 ) ) ;
#9188=CARTESIAN_POINT ( 'NONE',  ( 3.044812012440130555, 197.4746971517856764, 77.60113791807857808 ) ) ;
#9189=CARTESIAN_POINT ( 'NONE',  ( -10.01549611932653860, 203.7984951890123000, 42.35113791807857098 ) ) ;
#9192=CARTESIAN_POINT ( 'NONE',  ( -12.01549611932659722, 210.8513442034533227, 8.648862081921436129 ) ) ;
#9193=CARTESIAN_POINT ( 'NONE',  ( -8.118202686958138514, 212.8392687619910930, 20.79886208192143471 ) ) ;
#9196=CARTESIAN_POINT ( 'NONE',  ( 12.00000000000000711, 206.9523078486586485, 47.00113791807856956 ) ) ;
#9198=CARTESIAN_POINT ( 'NONE',  ( 4.984841277089725686, 213.7757310962907411, 73.55113791807856671 ) ) ;
#9199=CARTESIAN_POINT ( 'NONE',  ( -6.220909254589682469, 215.4770327129946850, 32.94886208192144039 ) ) ;
#9204=CARTESIAN_POINT ( 'NONE',  ( -10.00000000000000711, 207.0476921513413515, 93.50113791807858377 ) ) ;
#9210=CARTESIAN_POINT ( 'NONE',  ( 6.500168698208129925, 211.6636982574063381, 19.70113791807856884 ) ) ;
#9212=CARTESIAN_POINT ( 'NONE',  ( 0.05014649552828275708, 196.4853777576173002, 7.748862081921435774 ) ) ;
#9215=CARTESIAN_POINT ( 'NONE',  ( 7.984503880673485376, 204.3529502787953902, 53.15113791807857524 ) ) ;
#9219=CARTESIAN_POINT ( 'NONE',  ( 9.984503880673420539, 210.2968891136705167, 90.84886208192143897 ) ) ;
#9221=CARTESIAN_POINT ( 'NONE',  ( 10.01549611932653860, 210.2015048109876716, 28.85113791807855677 ) ) ;
#9223=CARTESIAN_POINT ( 'NONE',  ( -7.375838497908014268, 196.7627149292498530, 80.04886208192144181 ) ) ;
#9228=CARTESIAN_POINT ( 'NONE',  ( -9.984503880673473830, 210.2968891136704315, 93.65113791807857524 ) ) ;
#9231=CARTESIAN_POINT ( 'NONE',  ( 0.05014649552810505201, 217.5146222423826714, 34.25113791807856956 ) ) ;
#9237=CARTESIAN_POINT ( 'NONE',  ( 9.736236675707914401, 214.0148392665762458, 19.70113791807856884 ) ) ;
#9241=CARTESIAN_POINT ( 'NONE',  ( 7.456977232089471386, 196.8216656703012006, 43.44886208192143329 ) ) ;
#9242=CARTESIAN_POINT ( 'NONE',  ( -3.044812012440131443, 216.5253028482142952, 4.101137918078565647 ) ) ;
#9243=CARTESIAN_POINT ( 'NONE',  ( 10.00000000000000711, 206.9523078486586201, 59.00113791807857666 ) ) ;
#9244=CARTESIAN_POINT ( 'NONE',  ( 7.984503880673422316, 209.6470497212048372, 9.848862081921433642 ) ) ;
#9247=CARTESIAN_POINT ( 'NONE',  ( 0.05014649552828262524, 198.5883022060938572, 97.74886208192141623 ) ) ;
#9249=CARTESIAN_POINT ( 'NONE',  ( -6.500168698208129925, 202.3363017425936050, 42.20113791807857240 ) ) ;
#9255=CARTESIAN_POINT ( 'NONE',  ( 10.00000000000000711, 207.0476921513415220, 60.99886208192143755 ) ) ;
#9258=CARTESIAN_POINT ( 'NONE',  ( -10.01549611932653860, 203.7984951890123284, 6.351137918078566535 ) ) ;
#9262=CARTESIAN_POINT ( 'NONE',  ( -8.015496119326597224, 209.5516654185217362, 83.64886208192143613 ) ) ;
#9266=CARTESIAN_POINT ( 'NONE',  ( -10.00000000000000711, 207.0476921513413515, 24.50113791807856600 ) ) ;
#9270=CARTESIAN_POINT ( 'NONE',  ( -7.375838497908182134, 217.2372850707499765, 84.95113791807858661 ) ) ;
#9273=CARTESIAN_POINT ( 'NONE',  ( -9.680171189290716072, 199.9079932115567146, 71.19886208192144750 ) ) ;
#9274=CARTESIAN_POINT ( 'NONE',  ( 6.220909254589680693, 198.5229672870052582, 79.44886208192143329 ) ) ;
#9275=CARTESIAN_POINT ( 'NONE',  ( 7.375838497908012492, 217.2372850707501186, 15.54886208192143826 ) ) ;
#9278=CARTESIAN_POINT ( 'NONE',  ( -3.044812012440131443, 216.5253028482142952, 34.10113791807857808 ) ) ;
#9280=CARTESIAN_POINT ( 'NONE',  ( -6.220909254589682469, 215.4770327129946850, 89.94886208192140487 ) ) ;
#9284=CARTESIAN_POINT ( 'NONE',  ( 7.984503880673422316, 209.6470497212048372, 72.84886208192143897 ) ) ;
#9291=CARTESIAN_POINT ( 'NONE',  ( -7.984503880673488041, 209.6470497212046098, 81.65113791807856103 ) ) ;
#9296=CARTESIAN_POINT ( 'NONE',  ( 6.500168698208244500, 202.3363017425938324, 49.29886208192144892 ) ) ;
#9304=CARTESIAN_POINT ( 'NONE',  ( -3.662846001190052991, 218.4274158808045740, 58.10113791807857808 ) ) ;
#9306=CARTESIAN_POINT ( 'NONE',  ( -9.949154985843399857, 217.7087784572769067, 102.9933096652613074 ) ) ;
#9307=CARTESIAN_POINT ( 'NONE',  ( 0.05014649552810506589, 217.5146222423826714, 79.25113791807856956 ) ) ;
#9308=CARTESIAN_POINT ( 'NONE',  ( 9.680171189290716072, 214.0920067884432854, 39.69886208192144039 ) ) ;
#9309=CARTESIAN_POINT ( 'NONE',  ( -3.135527875058982783, 216.4958274776886924, 48.09886208192143187 ) ) ;
#9311=CARTESIAN_POINT ( 'NONE',  ( -3.753561863808691168, 195.6020594897209435, 83.90113791807856103 ) ) ;
#9312=CARTESIAN_POINT ( 'NONE',  ( -2.426778023690262742, 214.6231898156240163, 100.1011379180785781 ) ) ;
#9314=CARTESIAN_POINT ( 'NONE',  ( -9.984503880673420539, 203.7031108863293980, 56.34886208192141765 ) ) ;
#9317=CARTESIAN_POINT ( 'NONE',  ( 9.736236675708031640, 199.9851607334238963, 67.29886208192144181 ) ) ;
#9321=CARTESIAN_POINT ( 'NONE',  ( -2.426778023690076225, 199.3768101843759553, 37.89886208192144323 ) ) ;
#9327=CARTESIAN_POINT ( 'NONE',  ( -8.015496119326531499, 204.4483345814780364, 60.35113791807857098 ) ) ;
#9329=CARTESIAN_POINT ( 'NONE',  ( -10.01549611932659722, 210.2015048109875011, 38.64886208192142192 ) ) ;
#9336=CARTESIAN_POINT ( 'NONE',  ( 8.000000000000008882, 207.0476921513415220, 21.99886208192143400 ) ) ;
#9337=CARTESIAN_POINT ( 'NONE',  ( -3.135527875058821579, 197.5041725223112223, 62.90113791807858235 ) ) ;
#9338=CARTESIAN_POINT ( 'NONE',  ( -8.062137200540920645, 212.9164362838581894, 48.80113791807857382 ) ) ;
#9340=CARTESIAN_POINT ( 'NONE',  ( 3.135527875058820690, 216.4958274776887492, 16.40113791807856813 ) ) ;
#9341=CARTESIAN_POINT ( 'NONE',  ( -8.015496119326597224, 209.5516654185217362, 101.6488620819214361 ) ) ;
#9344=CARTESIAN_POINT ( 'NONE',  ( 12.01549611932652972, 210.8513442034534933, 28.85113791807856032 ) ) ;
#9347=CARTESIAN_POINT ( 'NONE',  ( -6.139770520408369237, 215.5359834540460042, 78.95113791807858661 ) ) ;
#9348=CARTESIAN_POINT ( 'NONE',  ( 8.118202686958039038, 212.8392687619912635, 52.70113791807857240 ) ) ;
#9351=CARTESIAN_POINT ( 'NONE',  ( -3.753561863808878130, 218.3979405102790281, 12.09886208192143364 ) ) ;
#9352=CARTESIAN_POINT ( 'NONE',  ( 3.044812012439969795, 216.5253028482143520, 15.39886208192143613 ) ) ;
#9356=CARTESIAN_POINT ( 'NONE',  ( -12.00000000000000711, 207.0476921513413515, 54.50113791807857666 ) ) ;
#9357=CARTESIAN_POINT ( 'NONE',  ( -6.444103211791042618, 211.7408657792732356, 72.80113791807858092 ) ) ;
#9359=CARTESIAN_POINT ( 'NONE',  ( -8.118202686958138514, 212.8392687619910930, 32.79886208192143471 ) ) ;
#9363=CARTESIAN_POINT ( 'NONE',  ( -8.062137200540920645, 212.9164362838581894, 87.80113791807856671 ) ) ;
#9370=CARTESIAN_POINT ( 'NONE',  ( -7.984503880673488041, 209.6470497212046098, 33.65113791807856813 ) ) ;
#9372=CARTESIAN_POINT ( 'NONE',  ( -6.139770520408224463, 198.4640165459539389, 11.04886208192143648 ) ) ;
#9374=ORIENTED_EDGE ( 'NONE', *, *, #15586, .F. ) ;
#9375=CARTESIAN_POINT ( 'NONE',  ( 2.426778023690261410, 199.3768101843759837, 53.60113791807856387 ) ) ;
#9380=CARTESIAN_POINT ( 'NONE',  ( 6.139770520408223575, 215.5359834540460611, 102.5488620819214134 ) ) ;
#9382=CARTESIAN_POINT ( 'NONE',  ( 6.139770520408368348, 198.4640165459539674, 35.45113791807857240 ) ) ;
#9384=CARTESIAN_POINT ( 'NONE',  ( 10.00000000000000711, 206.9523078486586201, 17.00113791807856600 ) ) ;
#9389=CARTESIAN_POINT ( 'NONE',  ( -9.680171189290831535, 214.0920067884431148, 0.8011379180785656029 ) ) ;
#9392=CARTESIAN_POINT ( 'NONE',  ( 10.00000000000000711, 206.9523078486586201, 44.00113791807857666 ) ) ;
#9400=CARTESIAN_POINT ( 'NONE',  ( -9.736236675707914401, 199.9851607334237542, 30.20113791807856529 ) ) ;
#9404=CARTESIAN_POINT ( 'NONE',  ( -10.00000000000000178, 208.0352956435529563, 102.7846294209004441 ) ) ;
#9405=ORIENTED_EDGE ( 'NONE', *, *, #7998, .F. ) ;
#9407=CARTESIAN_POINT ( 'NONE',  ( 9.680171189290716072, 214.0920067884432854, 42.69886208192142618 ) ) ;
#9409=CARTESIAN_POINT ( 'NONE',  ( 10.01549611932653860, 210.2015048109876716, 61.85113791807857098 ) ) ;
#9411=CARTESIAN_POINT ( 'NONE',  ( -4.984841277089891776, 213.7757310962905990, 20.94886208192143684 ) ) ;
#9414=CARTESIAN_POINT ( 'NONE',  ( 6.444103211791042618, 202.2591342207267644, 2.301137918078565825 ) ) ;
#9416=CARTESIAN_POINT ( 'NONE',  ( 12.00000000000000711, 207.0476921513415220, 90.99886208192144466 ) ) ;
#9423=CARTESIAN_POINT ( 'NONE',  ( 9.984503880673420539, 210.2968891136705167, 60.84886208192142476 ) ) ;
#9426=CARTESIAN_POINT ( 'NONE',  ( 6.139770520408368348, 198.4640165459539674, 2.451137918078566180 ) ) ;
#9432=CARTESIAN_POINT ( 'NONE',  ( -6.444103211790928043, 202.2591342207265939, 86.19886208192144750 ) ) ;
#9436=CARTESIAN_POINT ( 'NONE',  ( 0.05014649552828288198, 194.3824533091408000, 85.74886208192143044 ) ) ;
#9439=CARTESIAN_POINT ( 'NONE',  ( 9.984503880673473830, 203.7031108863295401, 17.15113791807856458 ) ) ;
#9443=CARTESIAN_POINT ( 'NONE',  ( 3.662846001190051659, 195.5725841191953691, 89.60113791807857808 ) ) ;
#9444=CARTESIAN_POINT ( 'NONE',  ( -8.118202686958039038, 201.1607312380087080, 102.2011379180785866 ) ) ;
#9446=CARTESIAN_POINT ( 'NONE',  ( 9.736236675708031640, 199.9851607334238963, 73.29886208192142760 ) ) ;
#9447=CARTESIAN_POINT ( 'NONE',  ( -8.118202686958138514, 212.8392687619910930, 74.79886208192144181 ) ) ;
#9448=CARTESIAN_POINT ( 'NONE',  ( -12.01549611932659722, 210.8513442034533227, 14.64886208192143258 ) ) ;
#9451=CARTESIAN_POINT ( 'NONE',  ( 3.044812012440130555, 197.4746971517856764, 29.60113791807856742 ) ) ;
#9453=CARTESIAN_POINT ( 'NONE',  ( 10.00000000000000711, 207.0476921513415220, 102.9988620819214447 ) ) ;
#9458=CARTESIAN_POINT ( 'NONE',  ( 4.903702542908435547, 213.8346818373419751, 66.54886208192144181 ) ) ;
#9465=CARTESIAN_POINT ( 'NONE',  ( 0.05014649552807626948, 215.4116977939061144, 76.25113791807856956 ) ) ;
#9468=CARTESIAN_POINT ( 'NONE',  ( -4.984841277089891776, 213.7757310962905990, 53.94886208192144039 ) ) ;
#9471=CARTESIAN_POINT ( 'NONE',  ( -10.00000000000000178, 208.0352956435529563, 102.7846294209004441 ) ) ;
#9474=CARTESIAN_POINT ( 'NONE',  ( -0.05014649552807705357, 194.3824533091408000, 53.75113791807857666 ) ) ;
#9476=CARTESIAN_POINT ( 'NONE',  ( -8.062137200540920645, 212.9164362838581894, 99.80113791807858092 ) ) ;
#9477=CARTESIAN_POINT ( 'NONE',  ( -10.00000000000000711, 207.0476921513413515, 81.50113791807856956 ) ) ;
#9478=CARTESIAN_POINT ( 'NONE',  ( 9.680171189290716072, 214.0920067884432854, 42.69886208192142618 ) ) ;
#9479=CARTESIAN_POINT ( 'NONE',  ( 8.118202686958138514, 201.1607312380088501, 49.29886208192143471 ) ) ;
#9481=CARTESIAN_POINT ( 'NONE',  ( 3.662846001190051659, 195.5725841191953691, 83.60113791807857808 ) ) ;
#9483=CARTESIAN_POINT ( 'NONE',  ( 0.05014649552810505201, 217.5146222423826714, 4.251137918078566003 ) ) ;
#9484=CARTESIAN_POINT ( 'NONE',  ( 9.984503880673420539, 210.2968891136705167, 63.84886208192142476 ) ) ;
#9488=CARTESIAN_POINT ( 'NONE',  ( 0.05014649552828288198, 194.3824533091408000, 70.74886208192144466 ) ) ;
#9492=CARTESIAN_POINT ( 'NONE',  ( 7.984503880673422316, 209.6470497212048372, 45.84886208192143897 ) ) ;
#9498=CARTESIAN_POINT ( 'NONE',  ( -6.444103211791042618, 211.7408657792732356, 63.80113791807858092 ) ) ;
#9500=CARTESIAN_POINT ( 'NONE',  ( -3.044812012439970683, 197.4746971517856196, 37.89886208192143613 ) ) ;
#9501=ORIENTED_EDGE ( 'NONE', *, *, #20637, .T. ) ;
#9505=CARTESIAN_POINT ( 'NONE',  ( 6.500168698208244500, 202.3363017425938324, 25.29886208192143826 ) ) ;
#9506=CARTESIAN_POINT ( 'NONE',  ( -0.05014649552810635652, 196.4853777576173002, 65.75113791807856956 ) ) ;
#9507=CARTESIAN_POINT ( 'NONE',  ( -3.135527875058821579, 197.5041725223112223, 44.90113791807857524 ) ) ;
#9510=CARTESIAN_POINT ( 'NONE',  ( -3.044812012440131443, 216.5253028482142952, 16.10113791807856742 ) ) ;
#9511=CARTESIAN_POINT ( 'NONE',  ( 4.903702542908601636, 200.1653181626581102, 2.451137918078566180 ) ) ;
#9515=CARTESIAN_POINT ( 'NONE',  ( -7.375838497908182134, 217.2372850707499765, 30.95113791807857595 ) ) ;
#9518=CARTESIAN_POINT ( 'NONE',  ( -3.044812012440131443, 216.5253028482142952, 79.10113791807857808 ) ) ;
#9519=CARTESIAN_POINT ( 'NONE',  ( 0.05014649552810506589, 217.5146222423826714, 46.25113791807857666 ) ) ;
#9522=CARTESIAN_POINT ( 'NONE',  ( -0.05014649552828442242, 219.6175466908591716, 9.248862081921435774 ) ) ;
#9523=CARTESIAN_POINT ( 'NONE',  ( 6.220909254589680693, 198.5229672870052582, 16.44886208192142973 ) ) ;
#9526=CARTESIAN_POINT ( 'NONE',  ( 12.01549611932652972, 210.8513442034534933, 58.85113791807857098 ) ) ;
#9527=CARTESIAN_POINT ( 'NONE',  ( -2.426778023690262742, 214.6231898156240163, 82.10113791807857808 ) ) ;
#9528=CARTESIAN_POINT ( 'NONE',  ( 8.118202686958138514, 201.1607312380088501, 31.29886208192143826 ) ) ;
#9537=CARTESIAN_POINT ( 'NONE',  ( 6.444103211791042618, 202.2591342207267644, 29.30113791807857027 ) ) ;
#9539=CARTESIAN_POINT ( 'NONE',  ( 8.118202686958138514, 201.1607312380088501, 16.29886208192143471 ) ) ;
#9542=CARTESIAN_POINT ( 'NONE',  ( -4.903702542908602524, 213.8346818373418898, 45.95113791807857950 ) ) ;
#9546=CARTESIAN_POINT ( 'NONE',  ( -9.984503880673420539, 203.7031108863293980, 98.34886208192143897 ) ) ;
#9548=CARTESIAN_POINT ( 'NONE',  ( -0.05014649552810635652, 196.4853777576173002, 35.75113791807857666 ) ) ;
#9549=PLANE ( 'NONE',  #11625 ) ;
#9551=CARTESIAN_POINT ( 'NONE',  ( 3.135527875058820690, 216.4958274776887492, 16.40113791807856813 ) ) ;
#9556=CARTESIAN_POINT ( 'NONE',  ( -10.00000000000000711, 207.0476921513413515, 102.5011379180785838 ) ) ;
#9559=CARTESIAN_POINT ( 'NONE',  ( 6.139770520408368348, 198.4640165459539674, 47.45113791807857950 ) ) ;
#9565=CARTESIAN_POINT ( 'NONE',  ( -3.753561863808691168, 195.6020594897209435, 29.90113791807857169 ) ) ;
#9566=CARTESIAN_POINT ( 'NONE',  ( -10.47863426674271814, 207.9189531262114770, 102.6635298682156758 ) ) ;
#9567=CARTESIAN_POINT ( 'NONE',  ( -3.044812012439970683, 197.4746971517856196, 4.898862081921434353 ) ) ;
#9570=CARTESIAN_POINT ( 'NONE',  ( -3.044812012440131443, 216.5253028482142952, 1.101137918078565869 ) ) ;
#9571=CARTESIAN_POINT ( 'NONE',  ( 10.01549611932653860, 210.2015048109876716, 64.85113791807857808 ) ) ;
#9572=CARTESIAN_POINT ( 'NONE',  ( 4.984841277089891776, 200.2242689037093726, 19.44886208192143329 ) ) ;
#9574=VERTEX_POINT ( 'NONE', #6495 ) ;
#9575=CARTESIAN_POINT ( 'NONE',  ( -6.444103211791042618, 211.7408657792732356, 6.801137918078567601 ) ) ;
#9580=CARTESIAN_POINT ( 'NONE',  ( -0.05014649552828442242, 219.6175466908591716, 90.24886208192144466 ) ) ;
#9584=DIRECTION ( 'NONE',  ( -0.9998603841633338929, 0.01669062914075312987, 0.0007969188393214247284 ) ) ;
#9586=CARTESIAN_POINT ( 'NONE',  ( 10.00000000000000711, 207.0476921513415220, 66.99886208192143044 ) ) ;
#9588=CARTESIAN_POINT ( 'NONE',  ( -10.00000000000000178, 207.9988620819213168, 103.5476921513414794 ) ) ;
#9589=CARTESIAN_POINT ( 'NONE',  ( 10.01549611932653860, 210.2015048109876716, 4.851137918078563871 ) ) ;
#9593=CARTESIAN_POINT ( 'NONE',  ( -8.118202686958039038, 201.1607312380087080, 87.20113791807858661 ) ) ;
#9596=CARTESIAN_POINT ( 'NONE',  ( -0.05014649552828365914, 215.4116977939061144, 87.24886208192144466 ) ) ;
#9600=CARTESIAN_POINT ( 'NONE',  ( -9.680171189290716072, 199.9079932115567146, 86.19886208192144750 ) ) ;
#9602=CARTESIAN_POINT ( 'NONE',  ( -3.044812012440131443, 216.5253028482142952, 16.10113791807856742 ) ) ;
#9606=CARTESIAN_POINT ( 'NONE',  ( -0.05014649552807705357, 194.3824533091408000, 86.75113791807856956 ) ) ;
#9609=CARTESIAN_POINT ( 'NONE',  ( 0.05014649552828288198, 194.3824533091408000, 70.74886208192144466 ) ) ;
#9610=CARTESIAN_POINT ( 'NONE',  ( 3.044812012439969795, 216.5253028482143520, 72.39886208192143613 ) ) ;
#9611=CARTESIAN_POINT ( 'NONE',  ( 0.05014649552828288198, 194.3824533091408000, 16.74886208192143755 ) ) ;
#9613=CARTESIAN_POINT ( 'NONE',  ( -10.01549611932653860, 203.7984951890123284, 33.35113791807855677 ) ) ;
#9615=CARTESIAN_POINT ( 'NONE',  ( 6.139770520408223575, 215.5359834540460611, 96.54886208192141339 ) ) ;
#9618=ORIENTED_EDGE ( 'NONE', *, *, #7029, .F. ) ;
#9620=CARTESIAN_POINT ( 'NONE',  ( 6.500168698208244500, 202.3363017425938324, 76.29886208192142760 ) ) ;
#9627=DIRECTION ( 'NONE',  ( 0.000000000000000000, 0.9988620819214357738, 0.04769215134144196705 ) ) ;
#9628=CARTESIAN_POINT ( 'NONE',  ( 0.05014649552807626948, 215.4116977939061144, 82.25113791807856956 ) ) ;
#9634=CARTESIAN_POINT ( 'NONE',  ( 8.000000000000008882, 207.0476921513415220, 57.99886208192144466 ) ) ;
#9641=CARTESIAN_POINT ( 'NONE',  ( -3.753561863808691168, 195.6020594897209435, 56.90113791807858235 ) ) ;
#9643=CARTESIAN_POINT ( 'NONE',  ( 6.220909254589536808, 215.4770327129947702, 100.5511379180785809 ) ) ;
#9644=CARTESIAN_POINT ( 'NONE',  ( -3.135527875058821579, 197.5041725223112223, 77.90113791807857524 ) ) ;
#9645=CARTESIAN_POINT ( 'NONE',  ( -9.736236675708031640, 214.0148392665760753, 38.79886208192142050 ) ) ;
#9646=CARTESIAN_POINT ( 'NONE',  ( 8.062137200540822946, 212.9164362838583315, 48.69886208192144039 ) ) ;
#9649=CARTESIAN_POINT ( 'NONE',  ( 11.98450388067348271, 203.0532714938637753, 86.15113791807856103 ) ) ;
#9652=CARTESIAN_POINT ( 'NONE',  ( 8.062137200540920645, 201.0835637161417822, 5.301137918078566713 ) ) ;
#9653=CARTESIAN_POINT ( 'NONE',  ( 10.00000000000000711, 207.0476921513415220, 69.99886208192143044 ) ) ;
#9658=CARTESIAN_POINT ( 'NONE',  ( 9.680171189290716072, 214.0920067884432854, 75.69886208192143329 ) ) ;
#9661=CARTESIAN_POINT ( 'NONE',  ( -4.903702542908436435, 200.1653181626580249, 56.04886208192144181 ) ) ;
#9669=CARTESIAN_POINT ( 'NONE',  ( -0.05014649552828403384, 217.5146222423826714, 45.24886208192143755 ) ) ;
#9675=CARTESIAN_POINT ( 'NONE',  ( 4.903702542908435547, 213.8346818373419751, 21.54886208192143471 ) ) ;
#9677=CARTESIAN_POINT ( 'NONE',  ( -3.135527875058821579, 197.5041725223112223, 59.90113791807856813 ) ) ;
#9679=CARTESIAN_POINT ( 'NONE',  ( 8.118202686958039038, 212.8392687619912635, 46.70113791807857240 ) ) ;
#9681=CARTESIAN_POINT ( 'NONE',  ( 9.984503880673470277, 203.7031108863295401, 14.15113791807856458 ) ) ;
#9682=CARTESIAN_POINT ( 'NONE',  ( 0.05014649552807626948, 215.4116977939061144, 4.251137918078566891 ) ) ;
#9686=CARTESIAN_POINT ( 'NONE',  ( -9.736236675707914401, 199.9851607334237542, 33.20113791807856529 ) ) ;
#9688=CARTESIAN_POINT ( 'NONE',  ( 8.062137200540920645, 201.0835637161417822, 80.30113791807858092 ) ) ;
#9689=CARTESIAN_POINT ( 'NONE',  ( 9.984503880673473830, 203.7031108863295401, 50.15113791807856813 ) ) ;
#9694=CARTESIAN_POINT ( 'NONE',  ( -0.05014649552828442242, 219.6175466908591716, 15.24886208192143577 ) ) ;
#9695=CARTESIAN_POINT ( 'NONE',  ( 3.044812012439969795, 216.5253028482143520, 18.39886208192143613 ) ) ;
#9698=CARTESIAN_POINT ( 'NONE',  ( -3.753561863808691168, 195.6020594897209435, 56.90113791807858235 ) ) ;
#9699=CARTESIAN_POINT ( 'NONE',  ( -0.05014649552807731031, 198.5883022060938572, 80.75113791807856956 ) ) ;
#9700=CARTESIAN_POINT ( 'NONE',  ( -3.135527875058982783, 216.4958274776886924, 39.09886208192143187 ) ) ;
#9712=CARTESIAN_POINT ( 'NONE',  ( 4.984841277089725686, 213.7757310962907411, 34.55113791807856671 ) ) ;
#9714=CARTESIAN_POINT ( 'NONE',  ( -3.135527875058982783, 216.4958274776886924, 9.098862081921435419 ) ) ;
#9718=CARTESIAN_POINT ( 'NONE',  ( 4.984841277089725686, 213.7757310962907411, 46.55113791807856671 ) ) ;
#9721=CARTESIAN_POINT ( 'NONE',  ( 10.01549611932659545, 203.7984951890123853, 97.14886208192145034 ) ) ;
#9723=CARTESIAN_POINT ( 'NONE',  ( -8.118202686958039038, 201.1607312380087080, 33.20113791807857240 ) ) ;
#9726=CARTESIAN_POINT ( 'NONE',  ( -6.139770520408369237, 215.5359834540460042, 21.95113791807856884 ) ) ;
#9731=CARTESIAN_POINT ( 'NONE',  ( 12.00000000000000711, 206.9523078486586485, -0.9988620819214344415 ) ) ;
#9735=CARTESIAN_POINT ( 'NONE',  ( -9.984503880673473830, 210.2968891136704315, 48.65113791807858235 ) ) ;
#9740=CARTESIAN_POINT ( 'NONE',  ( 10.01549611932659367, 203.7984951890124421, 28.14886208192144323 ) ) ;
#9744=CARTESIAN_POINT ( 'NONE',  ( 11.98450388067348271, 203.0532714938637753, 32.15113791807856103 ) ) ;
#9746=CARTESIAN_POINT ( 'NONE',  ( 12.01549611932659367, 203.1486557965466773, 103.1488620819214361 ) ) ;
#9750=CARTESIAN_POINT ( 'NONE',  ( -6.139770520408369237, 215.5359834540460042, 0.9511379180785658471 ) ) ;
#9751=CARTESIAN_POINT ( 'NONE',  ( -6.139770520408369237, 215.5359834540460042, 60.95113791807857950 ) ) ;
#9754=CARTESIAN_POINT ( 'NONE',  ( 7.984503880673422316, 209.6470497212048372, 24.84886208192143897 ) ) ;
#9757=CARTESIAN_POINT ( 'NONE',  ( -8.000000000000008882, 207.0476921513413515, 3.501137918078566003 ) ) ;
#9761=CARTESIAN_POINT ( 'NONE',  ( 9.736236675708031640, 199.9851607334238963, 88.29886208192142760 ) ) ;
#9767=CARTESIAN_POINT ( 'NONE',  ( 3.135527875058981895, 197.5041725223112792, 73.59886208192143897 ) ) ;
#9770=CARTESIAN_POINT ( 'NONE',  ( 8.062137200540920645, 201.0835637161417822, 8.301137918078566713 ) ) ;
#9773=CARTESIAN_POINT ( 'NONE',  ( -8.118202686958039038, 201.1607312380087080, 93.20113791807857240 ) ) ;
#9775=CARTESIAN_POINT ( 'NONE',  ( 6.139770520408368348, 198.4640165459539674, 77.45113791807854398 ) ) ;
#9777=FACE_OUTER_BOUND ( 'NONE', #1325, .T. ) ;
#9778=CARTESIAN_POINT ( 'NONE',  ( 12.00000000000000711, 207.0476921513415220, 90.99886208192144466 ) ) ;
#9780=CARTESIAN_POINT ( 'NONE',  ( 3.044812012440130555, 197.4746971517856764, 32.60113791807857098 ) ) ;
#9784=CARTESIAN_POINT ( 'NONE',  ( -0.05014649552807705357, 194.3824533091408000, 89.75113791807858377 ) ) ;
#9789=CARTESIAN_POINT ( 'NONE',  ( -12.01549611932659722, 210.8513442034533227, 68.64886208192142192 ) ) ;
#9790=CARTESIAN_POINT ( 'NONE',  ( 6.220909254589680693, 198.5229672870052582, 88.44886208192144750 ) ) ;
#9791=CARTESIAN_POINT ( 'NONE',  ( -3.662846001189865142, 195.5725841191952838, 13.89886208192143613 ) ) ;
#9793=CARTESIAN_POINT ( 'NONE',  ( -0.05014649552810635652, 196.4853777576173002, 29.75113791807856956 ) ) ;
#9796=CARTESIAN_POINT ( 'NONE',  ( -10.00000000000000711, 206.9523078486584495, 98.49886208192143044 ) ) ;
#9798=ORIENTED_EDGE ( 'NONE', *, *, #15338, .T. ) ;
#9800=CARTESIAN_POINT ( 'NONE',  ( 2.426778023690075337, 214.6231898156240447, 78.39886208192143613 ) ) ;
#9803=B_SPLINE_CURVE_WITH_KNOTS ( 'NONE', 3,
 ( #4758, #23329, #4312, #1867 ),
 .UNSPECIFIED., .F., .F.,
 ( 4, 4 ),
 ( 0.0001200665308319763828, 0.0006294823820153499106 ),
 .UNSPECIFIED. ) ;
#9812=CARTESIAN_POINT ( 'NONE',  ( -0.05014649552807731031, 198.5883022060938572, 77.75113791807856956 ) ) ;
#9816=CARTESIAN_POINT ( 'NONE',  ( 4.984841277089891776, 200.2242689037093726, 52.44886208192144039 ) ) ;
#9822=CARTESIAN_POINT ( 'NONE',  ( 12.01549611932652972, 210.8513442034534933, 55.85113791807856387 ) ) ;
#9824=CARTESIAN_POINT ( 'NONE',  ( -7.375838497908182134, 217.2372850707499765, 3.951137918078565736 ) ) ;
#9826=CARTESIAN_POINT ( 'NONE',  ( -9.984503880673475606, 210.2968891136704315, 75.65113791807857524 ) ) ;
#9828=CARTESIAN_POINT ( 'NONE',  ( -3.662846001189865142, 195.5725841191952838, 37.89886208192143613 ) ) ;
#9829=CARTESIAN_POINT ( 'NONE',  ( -9.984503880673420539, 203.7031108863293980, 44.34886208192143187 ) ) ;
#9831=CARTESIAN_POINT ( 'NONE',  ( -11.98450388067348804, 210.9467285061362247, 87.65113791807857524 ) ) ;
#9833=CARTESIAN_POINT ( 'NONE',  ( 3.135527875058820690, 216.4958274776887492, 7.401137918078566358 ) ) ;
#9835=CARTESIAN_POINT ( 'NONE',  ( 9.984503880673420539, 210.2968891136705167, 72.84886208192143897 ) ) ;
#9838=CARTESIAN_POINT ( 'NONE',  ( -9.736236675708031640, 214.0148392665760753, 74.79886208192142760 ) ) ;
#9841=CARTESIAN_POINT ( 'NONE',  ( 6.500168698208244500, 202.3363017425938324, 52.29886208192144892 ) ) ;
#9848=CARTESIAN_POINT ( 'NONE',  ( 0.05014649552828275708, 196.4853777576173002, 40.74886208192143044 ) ) ;
#9854=CARTESIAN_POINT ( 'NONE',  ( 0.05014649552828262524, 198.5883022060938572, 22.74886208192143755 ) ) ;
#9855=CARTESIAN_POINT ( 'NONE',  ( 10.00000000000000711, 206.9523078486586201, 68.00113791807856956 ) ) ;
#9857=CARTESIAN_POINT ( 'NONE',  ( -6.139770520408369237, 215.5359834540460042, 45.95113791807857950 ) ) ;
#9858=CARTESIAN_POINT ( 'NONE',  ( -8.118202686958039038, 201.1607312380087080, 15.20113791807856884 ) ) ;
#9859=CARTESIAN_POINT ( 'NONE',  ( -2.426778023690262742, 214.6231898156240163, 4.101137918078565647 ) ) ;
#9862=CARTESIAN_POINT ( 'NONE',  ( 9.736236675707914401, 214.0148392665762458, 28.70113791807857240 ) ) ;
#9864=CARTESIAN_POINT ( 'NONE',  ( 10.00000000000000711, 206.9523078486586201, 71.00113791807858377 ) ) ;
#9865=CARTESIAN_POINT ( 'NONE',  ( 6.139770520408367460, 198.4640165459539389, 53.45113791807856529 ) ) ;
#9868=CARTESIAN_POINT ( 'NONE',  ( 7.456977232089471386, 196.8216656703012006, 16.44886208192143684 ) ) ;
#9869=CARTESIAN_POINT ( 'NONE',  ( -9.984503880673420539, 203.7031108863293980, 14.34886208192143542 ) ) ;
#9873=CARTESIAN_POINT ( 'NONE',  ( -7.375838497908182134, 217.2372850707499765, 54.95113791807855819 ) ) ;
#9874=CARTESIAN_POINT ( 'NONE',  ( 6.444103211791042618, 202.2591342207267644, 74.30113791807858092 ) ) ;
#9875=CARTESIAN_POINT ( 'NONE',  ( 10.01549611932659545, 203.7984951890123853, 40.14886208192143613 ) ) ;
#9885=CARTESIAN_POINT ( 'NONE',  ( -4.984841277089726574, 200.2242689037092305, 30.05113791807857027 ) ) ;
#9887=CARTESIAN_POINT ( 'NONE',  ( 6.220909254589681581, 198.5229672870052582, 10.44886208192143506 ) ) ;
#9890=CARTESIAN_POINT ( 'NONE',  ( -8.000000000000008882, 207.0476921513413515, 63.50113791807856956 ) ) ;
#9892=VECTOR ( 'NONE', #8882, 1000.000000000000227 ) ;
#9895=CARTESIAN_POINT ( 'NONE',  ( -3.044812012439970683, 197.4746971517856196, 100.8988620819214361 ) ) ;
#9897=CARTESIAN_POINT ( 'NONE',  ( -9.984503880673473830, 210.2968891136704315, 42.65113791807856813 ) ) ;
#9899=CARTESIAN_POINT ( 'NONE',  ( -9.984503880673473830, 210.2968891136704315, 18.65113791807856813 ) ) ;
#9906=CARTESIAN_POINT ( 'NONE',  ( 9.680171189290831535, 199.9079932115568852, 2.301137918078565825 ) ) ;
#9909=CARTESIAN_POINT ( 'NONE',  ( -10.01549611932653860, 203.7984951890123284, 45.35113791807857808 ) ) ;
#9915=CARTESIAN_POINT ( 'NONE',  ( 11.98450388067348271, 203.0532714938637753, 26.15113791807857169 ) ) ;
#9917=CARTESIAN_POINT ( 'NONE',  ( 10.00000000000000711, 207.0476921513415220, 12.99886208192143400 ) ) ;
#9920=CARTESIAN_POINT ( 'NONE',  ( 3.135527875058820690, 216.4958274776887492, 7.401137918078566358 ) ) ;
#9921=CARTESIAN_POINT ( 'NONE',  ( 10.00000000000000711, 206.9523078486586201, 62.00113791807856956 ) ) ;
#9923=CARTESIAN_POINT ( 'NONE',  ( 8.000000000000008882, 207.0476921513415220, 18.99886208192143400 ) ) ;
#9928=CARTESIAN_POINT ( 'NONE',  ( -4.903702542908602524, 213.8346818373418898, 6.951137918078566180 ) ) ;
#9931=CARTESIAN_POINT ( 'NONE',  ( -0.05014649552828442242, 219.6175466908591716, 93.24886208192143044 ) ) ;
#9938=CARTESIAN_POINT ( 'NONE',  ( 3.044812012439969795, 216.5253028482143520, 69.39886208192143613 ) ) ;
#9941=CARTESIAN_POINT ( 'NONE',  ( 6.139770520408368348, 198.4640165459539674, -0.5488620819214343749 ) ) ;
#9944=CARTESIAN_POINT ( 'NONE',  ( 6.139770520408368348, 198.4640165459539674, 92.45113791807857240 ) ) ;
#9946=CARTESIAN_POINT ( 'NONE',  ( -3.135527875058821579, 197.5041725223112223, 71.90113791807857524 ) ) ;
#9949=CARTESIAN_POINT ( 'NONE',  ( -7.375838497908014268, 196.7627149292498530, 89.04886208192142760 ) ) ;
#9951=CARTESIAN_POINT ( 'NONE',  ( 10.01549611932653860, 210.2015048109876716, 34.85113791807857098 ) ) ;
#9956=CARTESIAN_POINT ( 'NONE',  ( -0.05014649552807705357, 194.3824533091408000, 98.75113791807856956 ) ) ;
#9961=CARTESIAN_POINT ( 'NONE',  ( -6.139770520408224463, 198.4640165459539105, 83.04886208192144181 ) ) ;
#9962=CARTESIAN_POINT ( 'NONE',  ( -9.680171189290716072, 199.9079932115567146, 23.19886208192143684 ) ) ;
#9964=CARTESIAN_POINT ( 'NONE',  ( -8.062137200540920645, 212.9164362838581894, 33.80113791807857382 ) ) ;
#9966=CARTESIAN_POINT ( 'NONE',  ( -9.984503880673420539, 203.7031108863293980, 98.34886208192143897 ) ) ;
#9972=CARTESIAN_POINT ( 'NONE',  ( 8.015496119326595448, 204.4483345814782638, 79.14886208192143613 ) ) ;
#9978=CIRCLE ( 'NONE', #29012, 1.000000000000000888 ) ;
#9982=CARTESIAN_POINT ( 'NONE',  ( 8.000000000000008882, 206.9523078486586485, 77.00113791807858377 ) ) ;
#9983=EDGE_CURVE ( 'NONE', #14862, #11826, #12944, .T. ) ;
#9987=CARTESIAN_POINT ( 'NONE',  ( -7.984503880673422316, 204.3529502787951628, 65.34886208192142476 ) ) ;
#9990=CARTESIAN_POINT ( 'NONE',  ( -3.044812012440131443, 216.5253028482142952, 4.101137918078565647 ) ) ;
#9996=CARTESIAN_POINT ( 'NONE',  ( 9.680171189290831535, 199.9079932115568852, 71.30113791807856671 ) ) ;
#10000=CARTESIAN_POINT ( 'NONE',  ( 0.05014649552807549926, 219.6175466908591716, 7.251137918078565114 ) ) ;
#10001=CARTESIAN_POINT ( 'NONE',  ( -0.05014649552810635652, 196.4853777576173002, 83.75113791807856956 ) ) ;
#10002=CARTESIAN_POINT ( 'NONE',  ( -9.680171189290716072, 199.9079932115567146, 41.19886208192144039 ) ) ;
#10003=CARTESIAN_POINT ( 'NONE',  ( 10.00000000000000711, 207.0476921513415220, 60.99886208192143755 ) ) ;
#10006=CARTESIAN_POINT ( 'NONE',  ( -9.680171189290831535, 214.0920067884431148, 96.80113791807858092 ) ) ;
#10008=CARTESIAN_POINT ( 'NONE',  ( 3.135527875058820690, 216.4958274776887492, 1.401137918078565914 ) ) ;
#10010=CARTESIAN_POINT ( 'NONE',  ( 0.05014649552828275708, 196.4853777576173002, 73.74886208192144466 ) ) ;
#10014=CARTESIAN_POINT ( 'NONE',  ( -3.662846001189865142, 195.5725841191952838, 67.89886208192143613 ) ) ;
#10015=CARTESIAN_POINT ( 'NONE',  ( 3.135527875058820690, 216.4958274776887492, 91.40113791807857524 ) ) ;
#10018=CARTESIAN_POINT ( 'NONE',  ( -0.05014649552828365914, 215.4116977939061144, 51.24886208192144466 ) ) ;
#10028=CARTESIAN_POINT ( 'NONE',  ( 0.05014649552828275708, 196.4853777576173002, 49.74886208192141623 ) ) ;
#10034=CARTESIAN_POINT ( 'NONE',  ( 2.517493886309087436, 199.4062855549015865, 22.59886208192143542 ) ) ;
#10036=CARTESIAN_POINT ( 'NONE',  ( 6.139770520408368348, 198.4640165459539674, 71.45113791807857240 ) ) ;
#10038=ADVANCED_FACE ( 'NONE', ( #12607 ), #10763, .T. ) ;
#10039=CARTESIAN_POINT ( 'NONE',  ( 8.062137200540920645, 201.0835637161417822, 59.30113791807857382 ) ) ;
#10041=CARTESIAN_POINT ( 'NONE',  ( -8.062137200540920645, 212.9164362838581894, 30.80113791807856671 ) ) ;
#10042=CARTESIAN_POINT ( 'NONE',  ( -6.444103211791042618, 211.7408657792732356, 0.8011379180785661580 ) ) ;
#10046=CARTESIAN_POINT ( 'NONE',  ( -7.375838497908182134, 217.2372850707499765, 33.95113791807856529 ) ) ;
#10048=CARTESIAN_POINT ( 'NONE',  ( 3.135527875058820690, 216.4958274776887492, 82.40113791807857524 ) ) ;
#10049=CARTESIAN_POINT ( 'NONE',  ( -8.118202686958039038, 201.1607312380087080, 48.20113791807857950 ) ) ;
#10051=CARTESIAN_POINT ( 'NONE',  ( -11.98450388067341876, 203.0532714938636047, 11.34886208192143542 ) ) ;
#10052=CARTESIAN_POINT ( 'NONE',  ( -6.220909254589682469, 215.4770327129947134, 26.94886208192143329 ) ) ;
#10055=CARTESIAN_POINT ( 'NONE',  ( 11.98450388067348271, 203.0532714938637753, 59.15113791807857524 ) ) ;
#10056=CARTESIAN_POINT ( 'NONE',  ( 4.984841277089725686, 213.7757310962907411, 82.55113791807858092 ) ) ;
#10057=CARTESIAN_POINT ( 'NONE',  ( -6.139770520408224463, 198.4640165459539389, 41.04886208192142760 ) ) ;
#10060=CARTESIAN_POINT ( 'NONE',  ( 9.680171189290716072, 214.0920067884432854, 39.69886208192144039 ) ) ;
#10067=CARTESIAN_POINT ( 'NONE',  ( 0.05014649552807626948, 215.4116977939061144, 31.25113791807856956 ) ) ;
#10069=CARTESIAN_POINT ( 'NONE',  ( -10.01549611932659722, 210.2015048109875011, 17.64886208192143613 ) ) ;
#10072=CARTESIAN_POINT ( 'NONE',  ( 6.444103211791042618, 202.2591342207267644, 56.30113791807857382 ) ) ;
#10075=CARTESIAN_POINT ( 'NONE',  ( -6.220909254589682469, 215.4770327129946850, 101.9488620819214333 ) ) ;
#10077=CARTESIAN_POINT ( 'NONE',  ( 3.135527875058820690, 216.4958274776887492, 37.40113791807857524 ) ) ;
#10079=CARTESIAN_POINT ( 'NONE',  ( 3.044812012440130555, 197.4746971517856764, 26.60113791807856742 ) ) ;
#10086=CARTESIAN_POINT ( 'NONE',  ( -7.375838497908182134, 217.2372850707499765, 0.9511379180785655141 ) ) ;
#10089=CARTESIAN_POINT ( 'NONE',  ( -6.220909254589537696, 198.5229672870051161, 45.05113791807855961 ) ) ;
#10095=CARTESIAN_POINT ( 'NONE',  ( -11.98450388067348804, 210.9467285061362247, 24.65113791807857169 ) ) ;
#10097=CARTESIAN_POINT ( 'NONE',  ( -6.220909254589682469, 215.4770327129946850, 8.948862081921435063 ) ) ;
#10100=CARTESIAN_POINT ( 'NONE',  ( 6.139770520408368348, 198.4640165459539674, 11.45113791807856707 ) ) ;
#10101=CARTESIAN_POINT ( 'NONE',  ( 9.984503880673470277, 203.7031108863295401, 68.15113791807857524 ) ) ;
#10103=CARTESIAN_POINT ( 'NONE',  ( -6.500168698208244500, 211.6636982574061676, 23.79886208192143826 ) ) ;
#10106=CARTESIAN_POINT ( 'NONE',  ( 2.426778023690261410, 199.3768101843759837, -0.3988620819214340751 ) ) ;
#10107=CARTESIAN_POINT ( 'NONE',  ( -12.00000000000000711, 206.9523078486584780, 92.49886208192144466 ) ) ;
#10109=ORIENTED_EDGE ( 'NONE', *, *, #27467, .T. ) ;
#10112=CARTESIAN_POINT ( 'NONE',  ( 6.220909254589536808, 215.4770327129947702, 4.551137918078564937 ) ) ;
#10113=CARTESIAN_POINT ( 'NONE',  ( -0.05014649552828403384, 217.5146222423826714, 72.24886208192140202 ) ) ;
#10116=CARTESIAN_POINT ( 'NONE',  ( 6.139770520408368348, 198.4640165459539674, 8.451137918078565292 ) ) ;
#10119=CARTESIAN_POINT ( 'NONE',  ( -8.062137200540920645, 212.9164362838581894, 96.80113791807858092 ) ) ;
#10121=CARTESIAN_POINT ( 'NONE',  ( -9.984503880673473830, 210.2968891136704315, 78.65113791807854682 ) ) ;
#10124=CARTESIAN_POINT ( 'NONE',  ( 0.05014649552828288198, 194.3824533091408000, 82.74886208192144466 ) ) ;
#10130=CARTESIAN_POINT ( 'NONE',  ( -12.00000000000000711, 207.0476921513413515, 99.50113791807856956 ) ) ;
#10133=CARTESIAN_POINT ( 'NONE',  ( 10.01549611932659367, 203.7984951890124421, 85.14886208192143613 ) ) ;
#10134=CARTESIAN_POINT ( 'NONE',  ( -12.00000000000000711, 206.9523078486584780, 26.49886208192143400 ) ) ;
#10136=CARTESIAN_POINT ( 'NONE',  ( -9.984503880673473830, 210.2968891136704315, 42.65113791807856813 ) ) ;
#10138=CARTESIAN_POINT ( 'NONE',  ( -8.062137200540822946, 201.0835637161416400, 101.1988620819214475 ) ) ;
#10142=CARTESIAN_POINT ( 'NONE',  ( -0.05014649552828365914, 215.4116977939061144, 81.24886208192143044 ) ) ;
#10147=CARTESIAN_POINT ( 'NONE',  ( 4.984841277089725686, 213.7757310962907411, 64.55113791807856671 ) ) ;
#10150=CARTESIAN_POINT ( 'NONE',  ( -0.05014649552807731031, 198.5883022060938572, 83.75113791807856956 ) ) ;
#10153=CARTESIAN_POINT ( 'NONE',  ( -2.517493886309087880, 214.5937144450984135, 60.09886208192145318 ) ) ;
#10157=CARTESIAN_POINT ( 'NONE',  ( -10.00000000000000711, 207.0476921513413515, 0.5011379180785656695 ) ) ;
#10162=CARTESIAN_POINT ( 'NONE',  ( -9.680171189290831535, 214.0920067884431148, 63.80113791807858092 ) ) ;
#10164=CARTESIAN_POINT ( 'NONE',  ( -12.01549611932652972, 203.1486557965464499, 6.351137918078565647 ) ) ;
#10166=CARTESIAN_POINT ( 'NONE',  ( -3.135527875058821579, 197.5041725223112223, 83.90113791807857524 ) ) ;
#10169=CARTESIAN_POINT ( 'NONE',  ( 9.736236675708031640, 199.9851607334238963, 55.29886208192143471 ) ) ;
#10170=CARTESIAN_POINT ( 'NONE',  ( -8.118202686958138514, 212.8392687619910930, 59.79886208192143471 ) ) ;
#10172=CARTESIAN_POINT ( 'NONE',  ( 11.98450388067348271, 203.0532714938637753, 98.15113791807856103 ) ) ;
#10174=CARTESIAN_POINT ( 'NONE',  ( 3.044812012440130555, 197.4746971517856764, 2.601137918078566091 ) ) ;
#10175=CARTESIAN_POINT ( 'NONE',  ( -6.139770520408224463, 198.4640165459539389, 71.04886208192139918 ) ) ;
#10178=CARTESIAN_POINT ( 'NONE',  ( 9.736236675708031640, 199.9851607334238963, 82.29886208192144181 ) ) ;
#10179=CARTESIAN_POINT ( 'NONE',  ( -6.220909254589537696, 198.5229672870051161, 93.05113791807853829 ) ) ;
#10182=CARTESIAN_POINT ( 'NONE',  ( 6.500168698208244500, 202.3363017425938324, 49.29886208192144892 ) ) ;
#10193=CARTESIAN_POINT ( 'NONE',  ( 6.220909254589681581, 198.5229672870052582, 49.44886208192144039 ) ) ;
#10199=CARTESIAN_POINT ( 'NONE',  ( -6.500168698208244500, 211.6636982574061676, 35.79886208192144181 ) ) ;
#10200=CARTESIAN_POINT ( 'NONE',  ( -3.044812012440131443, 216.5253028482142952, 73.10113791807857808 ) ) ;
#10202=CARTESIAN_POINT ( 'NONE',  ( 3.044812012440130555, 197.4746971517856764, 56.60113791807857098 ) ) ;
#10203=CARTESIAN_POINT ( 'NONE',  ( -9.984503880673473830, 210.2968891136704315, 27.65113791807855748 ) ) ;
#10204=CARTESIAN_POINT ( 'NONE',  ( -8.015496119326531499, 204.4483345814780364, 18.35113791807856387 ) ) ;
#10208=CARTESIAN_POINT ( 'NONE',  ( -11.98450388067348804, 210.9467285061362247, 42.65113791807856813 ) ) ;
#10211=CARTESIAN_POINT ( 'NONE',  ( 0.05014649552810505201, 217.5146222423826714, 88.25113791807858377 ) ) ;
#10212=CARTESIAN_POINT ( 'NONE',  ( -6.220909254589537696, 198.5229672870051445, 63.05113791807858092 ) ) ;
#10215=CARTESIAN_POINT ( 'NONE',  ( 7.456977232089471386, 196.8216656703012006, 19.44886208192143329 ) ) ;
#10217=CARTESIAN_POINT ( 'NONE',  ( 9.984503880673420539, 210.2968891136705736, 30.84886208192143187 ) ) ;
#10220=CARTESIAN_POINT ( 'NONE',  ( -7.456977232089304408, 196.8216656703010301, 72.05113791807858092 ) ) ;
#10221=CARTESIAN_POINT ( 'NONE',  ( 2.426778023690261410, 199.3768101843759837, 74.60113791807854966 ) ) ;
#10223=CARTESIAN_POINT ( 'NONE',  ( 6.139770520408223575, 215.5359834540460611, 42.54886208192142050 ) ) ;
#10228=CARTESIAN_POINT ( 'NONE',  ( -7.456977232089471386, 217.1783343296987709, 47.94886208192143329 ) ) ;
#10235=CARTESIAN_POINT ( 'NONE',  ( -4.903702542908602524, 213.8346818373418898, 39.95113791807856529 ) ) ;
#10241=CARTESIAN_POINT ( 'NONE',  ( 8.118202686958138514, 201.1607312380088501, 19.29886208192143471 ) ) ;
#10248=CARTESIAN_POINT ( 'NONE',  ( -4.903702542908436435, 200.1653181626580249, 2.048862081921434708 ) ) ;
#10249=CARTESIAN_POINT ( 'NONE',  ( -10.01549611932653860, 203.7984951890123284, 39.35113791807857098 ) ) ;
#10251=CARTESIAN_POINT ( 'NONE',  ( 8.062137200540920645, 201.0835637161417822, 26.30113791807856671 ) ) ;
#10252=CARTESIAN_POINT ( 'NONE',  ( -6.220909254589682469, 215.4770327129947134, 101.9488620819214617 ) ) ;
#10254=CARTESIAN_POINT ( 'NONE',  ( 4.984841277089891776, 200.2242689037093726, 85.44886208192144750 ) ) ;
#10258=CARTESIAN_POINT ( 'NONE',  ( -0.05014649552807705357, 194.3824533091408000, 8.751137918078567779 ) ) ;
#10261=CARTESIAN_POINT ( 'NONE',  ( 8.062137200540920645, 201.0835637161417822, 56.30113791807857382 ) ) ;
#10269=CARTESIAN_POINT ( 'NONE',  ( 9.680171189290831535, 199.9079932115568852, 41.30113791807857382 ) ) ;
#10272=CARTESIAN_POINT ( 'NONE',  ( -6.220909254589682469, 215.4770327129946850, 14.94886208192143151 ) ) ;
#10276=CARTESIAN_POINT ( 'NONE',  ( 3.135527875058820690, 216.4958274776887492, 10.40113791807856636 ) ) ;
#10277=CARTESIAN_POINT ( 'NONE',  ( -6.139770520408369237, 215.5359834540460042, 72.95113791807854398 ) ) ;
#10279=CARTESIAN_POINT ( 'NONE',  ( -0.05014649552828365914, 215.4116977939061144, 36.24886208192143755 ) ) ;
#10283=CARTESIAN_POINT ( 'NONE',  ( 4.984841277089725686, 213.7757310962907411, 13.55113791807856849 ) ) ;
#10284=CARTESIAN_POINT ( 'NONE',  ( 3.753561863808876797, 195.6020594897209719, 100.5988620819214532 ) ) ;
#10289=CARTESIAN_POINT ( 'NONE',  ( 3.135527875058820690, 216.4958274776887492, 7.401137918078566358 ) ) ;
#10290=CARTESIAN_POINT ( 'NONE',  ( -3.044812012439970683, 197.4746971517856196, 67.89886208192143613 ) ) ;
#10292=CARTESIAN_POINT ( 'NONE',  ( 8.062137200540920645, 201.0835637161417822, 11.30113791807856671 ) ) ;
#10298=CARTESIAN_POINT ( 'NONE',  ( -0.05014649552810635652, 196.4853777576173002, 95.75113791807856956 ) ) ;
#10300=CARTESIAN_POINT ( 'NONE',  ( 9.984503880673470277, 203.7031108863295401, 74.15113791807854682 ) ) ;
#10303=CARTESIAN_POINT ( 'NONE',  ( 12.01549611932659367, 203.1486557965466773, 100.1488620819214646 ) ) ;
#10308=CARTESIAN_POINT ( 'NONE',  ( 9.680171189290831535, 199.9079932115568852, 95.30113791807858092 ) ) ;
#10311=CARTESIAN_POINT ( 'NONE',  ( -6.139770520408224463, 198.4640165459539105, 86.04886208192144181 ) ) ;
#10312=CARTESIAN_POINT ( 'NONE',  ( 0.05014649552828288198, 194.3824533091408000, 19.74886208192143400 ) ) ;
#10315=CARTESIAN_POINT ( 'NONE',  ( 10.00000000000000711, 206.9523078486586201, 44.00113791807857666 ) ) ;
#10317=CARTESIAN_POINT ( 'NONE',  ( 7.984503880673422316, 209.6470497212048372, 3.848862081921434530 ) ) ;
#10321=CARTESIAN_POINT ( 'NONE',  ( 8.000000000000008882, 207.0476921513415220, 81.99886208192144466 ) ) ;
#10327=CARTESIAN_POINT ( 'NONE',  ( -4.903702542908602524, 213.8346818373418898, 57.95113791807855819 ) ) ;
#10330=CARTESIAN_POINT ( 'NONE',  ( 2.426778023690261410, 199.3768101843759837, 86.60113791807857808 ) ) ;
#10333=CARTESIAN_POINT ( 'NONE',  ( 6.444103211790928043, 211.7408657792734061, 60.69886208192144750 ) ) ;
#10337=CARTESIAN_POINT ( 'NONE',  ( -8.062137200540920645, 212.9164362838581894, 3.801137918078565825 ) ) ;
#10341=CARTESIAN_POINT ( 'NONE',  ( -3.662846001190052991, 218.4274158808045740, 64.10113791807857808 ) ) ;
#10344=CARTESIAN_POINT ( 'NONE',  ( -12.01549611932652972, 203.1486557965464499, 12.35113791807856565 ) ) ;
#10345=CARTESIAN_POINT ( 'NONE',  ( -6.139770520408368348, 215.5359834540460042, 84.95113791807858661 ) ) ;
#10346=CARTESIAN_POINT ( 'NONE',  ( -12.00000000000000711, 206.9523078486584780, 53.49886208192144466 ) ) ;
#10347=CARTESIAN_POINT ( 'NONE',  ( 8.118202686958138514, 201.1607312380088501, 58.29886208192143471 ) ) ;
#10348=CARTESIAN_POINT ( 'NONE',  ( 9.736236675707914401, 214.0148392665762458, 94.70113791807858661 ) ) ;
#10350=CARTESIAN_POINT ( 'NONE',  ( -8.118202686958039038, 201.1607312380087080, 18.20113791807856884 ) ) ;
#10351=CARTESIAN_POINT ( 'NONE',  ( 10.00000000000000711, 207.0476921513415220, 72.99886208192144466 ) ) ;
#10353=CARTESIAN_POINT ( 'NONE',  ( -0.05014649552828442242, 219.6175466908591716, 78.24886208192144466 ) ) ;
#10354=CARTESIAN_POINT ( 'NONE',  ( -9.898309971686792608, 228.3698647632124334, 103.4854814124440452 ) ) ;
#10357=CARTESIAN_POINT ( 'NONE',  ( -2.517493886309087880, 214.5937144450984135, 51.09886208192143897 ) ) ;
#10365=CARTESIAN_POINT ( 'NONE',  ( 6.139770520408223575, 215.5359834540460611, 54.54886208192144181 ) ) ;
#10370=CARTESIAN_POINT ( 'NONE',  ( -2.517493886309087880, 214.5937144450984135, 30.09886208192144252 ) ) ;
#10371=CARTESIAN_POINT ( 'NONE',  ( -8.118202686958039038, 201.1607312380087080, 69.20113791807858661 ) ) ;
#10373=CARTESIAN_POINT ( 'NONE',  ( -10.00000000000000711, 207.0476921513413515, 54.50113791807857666 ) ) ;
#10374=CARTESIAN_POINT ( 'NONE',  ( 10.01549611932653860, 210.2015048109876716, 31.85113791807857453 ) ) ;
#10375=CARTESIAN_POINT ( 'NONE',  ( -8.000000000000008882, 207.0476921513413515, 12.50113791807856600 ) ) ;
#10376=CARTESIAN_POINT ( 'NONE',  ( -10.00000000000000178, 207.7681335166370502, 108.3800599224786367 ) ) ;
#10379=CARTESIAN_POINT ( 'NONE',  ( -0.05014649552807705357, 194.3824533091408000, 41.75113791807856245 ) ) ;
#10382=CARTESIAN_POINT ( 'NONE',  ( -0.05014649552810635652, 196.4853777576173002, 80.75113791807854113 ) ) ;
#10383=CARTESIAN_POINT ( 'NONE',  ( 3.044812012440130555, 197.4746971517856764, 59.60113791807857808 ) ) ;
#10385=CARTESIAN_POINT ( 'NONE',  ( -11.98450388067341876, 203.0532714938636047, 23.34886208192143542 ) ) ;
#10386=CARTESIAN_POINT ( 'NONE',  ( 9.984503880673420539, 210.2968891136705736, 24.84886208192143897 ) ) ;
#10388=CARTESIAN_POINT ( 'NONE',  ( -9.736236675707914401, 199.9851607334237542, 66.20113791807857240 ) ) ;
#10389=CARTESIAN_POINT ( 'NONE',  ( 0.05014649552807626948, 215.4116977939061144, 88.25113791807856956 ) ) ;
#10391=CARTESIAN_POINT ( 'NONE',  ( -9.984503880673420539, 203.7031108863293980, 44.34886208192142476 ) ) ;
#10394=CARTESIAN_POINT ( 'NONE',  ( 3.753561863808876797, 195.6020594897209719, 49.59886208192143897 ) ) ;
#10402=CARTESIAN_POINT ( 'NONE',  ( -6.500168698208129925, 202.3363017425936050, 45.20113791807857240 ) ) ;
#10403=CARTESIAN_POINT ( 'NONE',  ( -10.01549611932659722, 210.2015048109875011, 23.64886208192142902 ) ) ;
#10409=CARTESIAN_POINT ( 'NONE',  ( 4.903702542908435547, 213.8346818373419751, 3.548862081921434264 ) ) ;
#10410=CARTESIAN_POINT ( 'NONE',  ( 8.062137200540920645, 201.0835637161417822, 41.30113791807857382 ) ) ;
#10413=CARTESIAN_POINT ( 'NONE',  ( -10.00000000000000711, 207.0476921513413515, 24.50113791807856600 ) ) ;
#10414=CARTESIAN_POINT ( 'NONE',  ( -3.044812012439970683, 197.4746971517856196, 100.8988620819214361 ) ) ;
#10417=CARTESIAN_POINT ( 'NONE',  ( 6.444103211790928043, 211.7408657792734061, 96.69886208192144750 ) ) ;
#10421=CARTESIAN_POINT ( 'NONE',  ( 3.662846001190051659, 195.5725841191953691, 8.601137918078565647 ) ) ;
#10425=CARTESIAN_POINT ( 'NONE',  ( 0.05014649552810505201, 217.5146222423826714, 61.25113791807856245 ) ) ;
#10431=CARTESIAN_POINT ( 'NONE',  ( -9.736236675707914401, 199.9851607334237542, 42.20113791807857240 ) ) ;
#10434=CARTESIAN_POINT ( 'NONE',  ( -6.139770520408224463, 198.4640165459539389, 11.04886208192143648 ) ) ;
#10437=CARTESIAN_POINT ( 'NONE',  ( 0.05014649552810505201, 217.5146222423826714, 7.251137918078566003 ) ) ;
#10438=CARTESIAN_POINT ( 'NONE',  ( 3.135527875058820690, 216.4958274776887492, 70.40113791807857524 ) ) ;
#10440=CARTESIAN_POINT ( 'NONE',  ( 2.517493886309087436, 199.4062855549015865, 31.59886208192144252 ) ) ;
#10444=CARTESIAN_POINT ( 'NONE',  ( 8.015496119326531499, 209.5516654185219636, 13.85113791807856742 ) ) ;
#10445=CARTESIAN_POINT ( 'NONE',  ( 9.680171189290716072, 214.0920067884432854, 96.69886208192144750 ) ) ;
#10450=CARTESIAN_POINT ( 'NONE',  ( -9.984503880673473830, 210.2968891136704315, 9.651137918078568134 ) ) ;
#10451=CARTESIAN_POINT ( 'NONE',  ( 3.135527875058981895, 197.5041725223112792, 79.59886208192143897 ) ) ;
#10454=CARTESIAN_POINT ( 'NONE',  ( -9.984503880673473830, 210.2968891136704315, 12.65113791807856281 ) ) ;
#10458=CARTESIAN_POINT ( 'NONE',  ( 8.062137200540920645, 201.0835637161417822, 101.3011379180785809 ) ) ;
#10461=CARTESIAN_POINT ( 'NONE',  ( -3.044812012440131443, 216.5253028482142952, 88.10113791807857808 ) ) ;
#10465=CARTESIAN_POINT ( 'NONE',  ( 0.05014649552828288198, 194.3824533091408000, 100.7488620819214304 ) ) ;
#10471=CARTESIAN_POINT ( 'NONE',  ( 12.00000000000000711, 206.9523078486586485, 101.0011379180785696 ) ) ;
#10474=CARTESIAN_POINT ( 'NONE',  ( 8.062137200540822946, 212.9164362838583315, 84.69886208192144750 ) ) ;
#10476=CARTESIAN_POINT ( 'NONE',  ( -3.753561863808878130, 218.3979405102790281, 24.09886208192143897 ) ) ;
#10478=CARTESIAN_POINT ( 'NONE',  ( 3.044812012440130555, 197.4746971517856764, 44.60113791807857098 ) ) ;
#10480=CARTESIAN_POINT ( 'NONE',  ( -6.500168698208244500, 211.6636982574061676, 2.798862081921434708 ) ) ;
#10483=CARTESIAN_POINT ( 'NONE',  ( 0.05014649552828262524, 198.5883022060938572, 91.74886208192144466 ) ) ;
#10485=CARTESIAN_POINT ( 'NONE',  ( 4.903702542908601636, 200.1653181626581102, 35.45113791807857240 ) ) ;
#10492=CARTESIAN_POINT ( 'NONE',  ( -4.984841277089726574, 200.2242689037092305, 90.05113791807858092 ) ) ;
#10497=CARTESIAN_POINT ( 'NONE',  ( 2.517493886309087436, 199.4062855549015865, 67.59886208192143897 ) ) ;
#10502=CARTESIAN_POINT ( 'NONE',  ( 8.118202686958039038, 212.8392687619912635, 4.701137918078565292 ) ) ;
#10506=CARTESIAN_POINT ( 'NONE',  ( -7.456977232089304408, 196.8216656703010301, 66.05113791807858092 ) ) ;
#10508=CARTESIAN_POINT ( 'NONE',  ( -7.456977232089304408, 196.8216656703010301, 9.051137918078564937 ) ) ;
#10509=CARTESIAN_POINT ( 'NONE',  ( 10.00000000000000711, 206.9523078486586201, 89.00113791807858377 ) ) ;
#10510=CARTESIAN_POINT ( 'NONE',  ( -1.474514954580286030E-14, 206.9977241638431167, -6.000000000000014211 ) ) ;
#10511=CARTESIAN_POINT ( 'NONE',  ( 12.00000000000000711, 207.0476921513415220, 51.99886208192143044 ) ) ;
#10512=CARTESIAN_POINT ( 'NONE',  ( 0.05014649552828275014, 196.4853777576173002, 61.74886208192143755 ) ) ;
#10513=CARTESIAN_POINT ( 'NONE',  ( -12.01549611932652972, 203.1486557965464499, 96.35113791807857808 ) ) ;
#10515=CARTESIAN_POINT ( 'NONE',  ( 8.118202686958039038, 212.8392687619912635, 10.70113791807856529 ) ) ;
#10516=CARTESIAN_POINT ( 'NONE',  ( -10.01549611932659722, 210.2015048109875011, 80.64886208192143613 ) ) ;
#10518=CARTESIAN_POINT ( 'NONE',  ( -9.680171189290716072, 199.9079932115567146, 77.19886208192143329 ) ) ;
#10519=CARTESIAN_POINT ( 'NONE',  ( 0.05014649552810505201, 217.5146222423826714, 97.25113791807854113 ) ) ;
#10520=CIRCLE ( 'NONE', #20275, 1.000000000000000888 ) ;
#10523=CARTESIAN_POINT ( 'NONE',  ( -7.984503880673422316, 204.3529502787951628, 65.34886208192142476 ) ) ;
#10531=CARTESIAN_POINT ( 'NONE',  ( 3.135527875058981895, 197.5041725223112792, 55.59886208192143187 ) ) ;
#10537=CARTESIAN_POINT ( 'NONE',  ( 0.05014649552828262524, 198.5883022060938572, 31.74886208192143755 ) ) ;
#10538=CARTESIAN_POINT ( 'NONE',  ( 8.118202686958039038, 212.8392687619912635, 70.70113791807857240 ) ) ;
#10540=CARTESIAN_POINT ( 'NONE',  ( -3.135527875058821579, 197.5041725223112223, 59.90113791807856813 ) ) ;
#10541=CARTESIAN_POINT ( 'NONE',  ( 9.984503880673470277, 203.7031108863295401, 23.15113791807856813 ) ) ;
#10542=CARTESIAN_POINT ( 'NONE',  ( -8.015496119326531499, 204.4483345814780364, 12.35113791807856565 ) ) ;
#10546=CARTESIAN_POINT ( 'NONE',  ( 3.753561863808689836, 218.3979405102790565, 40.40113791807857524 ) ) ;
#10549=CARTESIAN_POINT ( 'NONE',  ( -8.118202686958039038, 201.1607312380087080, 84.20113791807858661 ) ) ;
#10551=CARTESIAN_POINT ( 'NONE',  ( -10.01549611932653860, 203.7984951890123000, 57.35113791807857098 ) ) ;
#10553=CARTESIAN_POINT ( 'NONE',  ( 9.736236675708031640, 199.9851607334238963, 25.29886208192143826 ) ) ;
#10554=CARTESIAN_POINT ( 'NONE',  ( -6.139770520408224463, 198.4640165459539105, 29.04886208192144181 ) ) ;
#10556=CARTESIAN_POINT ( 'NONE',  ( 7.456977232089302632, 217.1783343296989131, 70.55113791807856671 ) ) ;
#10557=CARTESIAN_POINT ( 'NONE',  ( 4.903702542908601636, 200.1653181626581102, 89.45113791807857240 ) ) ;
#10558=CARTESIAN_POINT ( 'NONE',  ( -10.01549611932659722, 210.2015048109875011, 50.64886208192143613 ) ) ;
#10561=CARTESIAN_POINT ( 'NONE',  ( 7.375838497908012492, 217.2372850707501186, 51.54886208192144181 ) ) ;
#10566=CARTESIAN_POINT ( 'NONE',  ( 7.984503880673485376, 204.3529502787953902, 38.15113791807856813 ) ) ;
#10569=CARTESIAN_POINT ( 'NONE',  ( 8.118202686958138514, 201.1607312380088501, 25.29886208192143826 ) ) ;
#10575=CARTESIAN_POINT ( 'NONE',  ( 4.903702542908435547, 213.8346818373419751, 6.548862081921434708 ) ) ;
#10577=CARTESIAN_POINT ( 'NONE',  ( -3.135527875058821579, 197.5041725223112223, 44.90113791807857524 ) ) ;
#10579=CARTESIAN_POINT ( 'NONE',  ( 0.05014649552810505201, 217.5146222423826714, 31.25113791807857311 ) ) ;
#10580=CARTESIAN_POINT ( 'NONE',  ( -9.945352646237287431, 205.9548993908332193, 104.4520571433695579 ) ) ;
#10582=CARTESIAN_POINT ( 'NONE',  ( 7.984503880673422316, 209.6470497212048372, 90.84886208192142476 ) ) ;
#10586=CARTESIAN_POINT ( 'NONE',  ( -3.662846001190052991, 218.4274158808045740, 7.101137918078566535 ) ) ;
#10589=CARTESIAN_POINT ( 'NONE',  ( -0.05014649552810635652, 196.4853777576173002, 56.75113791807855534 ) ) ;
#10591=CARTESIAN_POINT ( 'NONE',  ( 6.139770520408367460, 198.4640165459539389, 26.45113791807856884 ) ) ;
#10598=CARTESIAN_POINT ( 'NONE',  ( -3.753561863808691168, 195.6020594897209435, 41.90113791807856813 ) ) ;
#10601=CARTESIAN_POINT ( 'NONE',  ( 10.00000000000000711, 207.0476921513415220, 18.99886208192143755 ) ) ;
#10603=ORIENTED_EDGE ( 'NONE', *, *, #6042, .T. ) ;
#10605=CARTESIAN_POINT ( 'NONE',  ( 8.062137200540920645, 201.0835637161417822, 68.30113791807856671 ) ) ;
#10609=CARTESIAN_POINT ( 'NONE',  ( 7.984503880673485376, 204.3529502787953902, 17.15113791807856458 ) ) ;
#10611=CARTESIAN_POINT ( 'NONE',  ( 9.736236675708031640, 199.9851607334238963, 97.29886208192142760 ) ) ;
#10616=CARTESIAN_POINT ( 'NONE',  ( -9.984503880673473830, 210.2968891136704315, 12.65113791807856281 ) ) ;
#10617=CARTESIAN_POINT ( 'NONE',  ( 8.118202686958138514, 201.1607312380088501, 82.29886208192144181 ) ) ;
#10621=CARTESIAN_POINT ( 'NONE',  ( -3.135527875058821579, 197.5041725223112223, 11.90113791807856636 ) ) ;
#10626=CARTESIAN_POINT ( 'NONE',  ( -10.00000000000000711, 207.0476921513413515, 84.50113791807856956 ) ) ;
#10629=CARTESIAN_POINT ( 'NONE',  ( -3.753561863808878130, 218.3979405102790281, 93.09886208192145318 ) ) ;
#10634=CARTESIAN_POINT ( 'NONE',  ( -9.736236675707914401, 199.9851607334237542, 93.20113791807858661 ) ) ;
#10637=CARTESIAN_POINT ( 'NONE',  ( 6.139770520408223575, 215.5359834540460611, 96.54886208192142760 ) ) ;
#10638=CARTESIAN_POINT ( 'NONE',  ( 3.753561863808876797, 195.6020594897209719, 19.59886208192143897 ) ) ;
#10640=CARTESIAN_POINT ( 'NONE',  ( -8.118202686958039038, 201.1607312380087080, 42.20113791807857240 ) ) ;
#10642=CARTESIAN_POINT ( 'NONE',  ( -8.015496119326597224, 209.5516654185217362, 8.648862081921436129 ) ) ;
#10647=CARTESIAN_POINT ( 'NONE',  ( -4.903702542908436435, 200.1653181626580249, 86.04886208192145602 ) ) ;
#10649=CARTESIAN_POINT ( 'NONE',  ( -6.444103211791042618, 211.7408657792732356, 27.80113791807857027 ) ) ;
#10657=CARTESIAN_POINT ( 'NONE',  ( 4.903702542908601636, 200.1653181626581102, 92.45113791807857240 ) ) ;
#10660=CARTESIAN_POINT ( 'NONE',  ( 8.015496119326595448, 204.4483345814782638, 64.14886208192143613 ) ) ;
#10663=CARTESIAN_POINT ( 'NONE',  ( -9.984503880673475606, 210.2968891136704315, 0.6511379180785656917 ) ) ;
#10667=CARTESIAN_POINT ( 'NONE',  ( 3.753561863808689836, 218.3979405102790565, 70.40113791807856103 ) ) ;
#10669=CARTESIAN_POINT ( 'NONE',  ( 3.135527875058820690, 216.4958274776887492, 85.40113791807857524 ) ) ;
#10671=CARTESIAN_POINT ( 'NONE',  ( 0.05014649552828288198, 194.3824533091408000, 49.74886208192143044 ) ) ;
#10672=CARTESIAN_POINT ( 'NONE',  ( -3.044812012439970683, 197.4746971517856196, 58.89886208192143613 ) ) ;
#10673=CARTESIAN_POINT ( 'NONE',  ( 12.01549611932652972, 210.8513442034534933, 94.85113791807856387 ) ) ;
#10675=CARTESIAN_POINT ( 'NONE',  ( -0.05014649552810635652, 196.4853777576173002, 11.75113791807856778 ) ) ;
#10676=CARTESIAN_POINT ( 'NONE',  ( 3.044812012439969795, 216.5253028482143520, 78.39886208192143613 ) ) ;
#10680=CARTESIAN_POINT ( 'NONE',  ( -2.426778023690076225, 199.3768101843759553, 61.89886208192143613 ) ) ;
#10684=CYLINDRICAL_SURFACE ( 'NONE', #32260, 1.000000000000000000 ) ;
#10687=CARTESIAN_POINT ( 'NONE',  ( 7.984503880673485376, 204.3529502787953902, 56.15113791807857524 ) ) ;
#10689=CARTESIAN_POINT ( 'NONE',  ( 10.00000000000000711, 207.0476921513415220, 54.99886208192143755 ) ) ;
#10690=AXIS2_PLACEMENT_3D ( 'NONE', #28518, #14880, #17609 ) ;
#10695=CARTESIAN_POINT ( 'NONE',  ( -4.984841277089891776, 213.7757310962905990, 32.94886208192144039 ) ) ;
#10696=CARTESIAN_POINT ( 'NONE',  ( -0.05014649552810635652, 196.4853777576173002, 83.75113791807856956 ) ) ;
#10698=CARTESIAN_POINT ( 'NONE',  ( 10.01549611932653860, 210.2015048109876716, 52.85113791807854966 ) ) ;
#10700=CARTESIAN_POINT ( 'NONE',  ( -8.118202686958039038, 201.1607312380087080, 27.20113791807856884 ) ) ;
#10701=CARTESIAN_POINT ( 'NONE',  ( -2.517493886308901807, 199.4062855549015012, 14.90113791807856636 ) ) ;
#10705=CARTESIAN_POINT ( 'NONE',  ( -12.00000000000000711, 207.0476921513413515, 39.50113791807856245 ) ) ;
#10707=CARTESIAN_POINT ( 'NONE',  ( 8.062137200540920645, 201.0835637161417822, 86.30113791807856671 ) ) ;
#10708=CARTESIAN_POINT ( 'NONE',  ( -3.135527875058821579, 197.5041725223112223, 59.90113791807856813 ) ) ;
#10709=CARTESIAN_POINT ( 'NONE',  ( -0.05014649552828442242, 219.6175466908591716, 21.24886208192143755 ) ) ;
#10710=CARTESIAN_POINT ( 'NONE',  ( 0.05014649552828275014, 196.4853777576173002, 25.74886208192143400 ) ) ;
#10712=CARTESIAN_POINT ( 'NONE',  ( 9.680171189290831535, 199.9079932115568852, 71.30113791807856671 ) ) ;
#10713=CARTESIAN_POINT ( 'NONE',  ( 4.903702542908601636, 200.1653181626581102, 92.45113791807857240 ) ) ;
#10714=CARTESIAN_POINT ( 'NONE',  ( -6.220909254589682469, 215.4770327129946850, 53.94886208192144039 ) ) ;
#10717=CARTESIAN_POINT ( 'NONE',  ( 3.753561863808876797, 195.6020594897209719, 55.59886208192143897 ) ) ;
#10724=CARTESIAN_POINT ( 'NONE',  ( -8.015496119326531499, 204.4483345814780364, 45.35113791807857098 ) ) ;
#10727=CARTESIAN_POINT ( 'NONE',  ( -8.118202686958138514, 212.8392687619910930, 20.79886208192143471 ) ) ;
#10732=CARTESIAN_POINT ( 'NONE',  ( 4.903702542908435547, 213.8346818373419751, 9.548862081921432932 ) ) ;
#10734=CARTESIAN_POINT ( 'NONE',  ( 10.00000000000000711, 206.9523078486586201, 47.00113791807856956 ) ) ;
#10736=CARTESIAN_POINT ( 'NONE',  ( -3.135527875058821579, 197.5041725223112223, 26.90113791807856813 ) ) ;
#10741=CARTESIAN_POINT ( 'NONE',  ( 8.000000000000008882, 207.0476921513415220, 93.99886208192144466 ) ) ;
#10745=CARTESIAN_POINT ( 'NONE',  ( -12.00000000000000711, 207.0476921513413515, 6.501137918078566891 ) ) ;
#10748=CARTESIAN_POINT ( 'NONE',  ( -10.00000000000000711, 207.0476921513413515, 54.50113791807857666 ) ) ;
#10749=CARTESIAN_POINT ( 'NONE',  ( -6.220909254589537696, 198.5229672870051445, 33.05113791807857382 ) ) ;
#10756=CARTESIAN_POINT ( 'NONE',  ( -7.375838497908182134, 217.2372850707499765, 42.95113791807857240 ) ) ;
#10758=CARTESIAN_POINT ( 'NONE',  ( -0.05014649552828403384, 217.5146222423826714, 18.24886208192143755 ) ) ;
#10762=CARTESIAN_POINT ( 'NONE',  ( -8.062137200540920645, 212.9164362838581894, 72.80113791807856671 ) ) ;
#10763=TOROIDAL_SURFACE ( 'NONE', #27620, 1.000000000000059064, 1.000000000000000222 ) ;
#10770=CARTESIAN_POINT ( 'NONE',  ( -0.05014649552807731031, 198.5883022060938572, 11.75113791807856600 ) ) ;
#10772=CARTESIAN_POINT ( 'NONE',  ( -12.01549611932659722, 210.8513442034533227, 101.6488620819214361 ) ) ;
#10778=CARTESIAN_POINT ( 'NONE',  ( 10.01549611932653860, 210.2015048109876716, 4.851137918078563871 ) ) ;
#10779=CARTESIAN_POINT ( 'NONE',  ( 8.062137200540822946, 212.9164362838583315, 78.69886208192143329 ) ) ;
#10782=CARTESIAN_POINT ( 'NONE',  ( 9.984503880673470277, 203.7031108863295401, 11.15113791807856636 ) ) ;
#10786=CARTESIAN_POINT ( 'NONE',  ( 6.139770520408368348, 198.4640165459539674, 98.45113791807854398 ) ) ;
#10788=CARTESIAN_POINT ( 'NONE',  ( 8.062137200540920645, 201.0835637161417822, 89.30113791807858092 ) ) ;
#10792=CARTESIAN_POINT ( 'NONE',  ( -7.375838497908014268, 196.7627149292498530, 95.04886208192144181 ) ) ;
#10798=EDGE_CURVE ( 'NONE', #25814, #24261, #13897, .T. ) ;
#10803=CARTESIAN_POINT ( 'NONE',  ( -9.984503880673420539, 203.7031108863293980, 95.34886208192143897 ) ) ;
#10804=CARTESIAN_POINT ( 'NONE',  ( 7.375838497908012492, 217.2372850707501186, 33.54886208192143471 ) ) ;
#10806=CARTESIAN_POINT ( 'NONE',  ( 8.118202686958039038, 212.8392687619912635, 40.70113791807857240 ) ) ;
#10807=ADVANCED_FACE ( 'NONE', ( #29578 ), #6231, .F. ) ;
#10809=CARTESIAN_POINT ( 'NONE',  ( 3.135527875058981895, 197.5041725223112792, 103.5988620819214390 ) ) ;
#10812=CARTESIAN_POINT ( 'NONE',  ( 2.426778023690075337, 214.6231898156240447, 93.39886208192143613 ) ) ;
#10815=CARTESIAN_POINT ( 'NONE',  ( 7.984503880673485376, 204.3529502787953902, 29.15113791807857169 ) ) ;
#10821=CARTESIAN_POINT ( 'NONE',  ( -4.984841277089726574, 200.2242689037092305, 84.05113791807858092 ) ) ;
#10825=CARTESIAN_POINT ( 'NONE',  ( 2.517493886309087436, 199.4062855549015865, 73.59886208192142476 ) ) ;
#10829=CARTESIAN_POINT ( 'NONE',  ( -6.139770520408368348, 215.5359834540460042, 12.95113791807856174 ) ) ;
#10834=CARTESIAN_POINT ( 'NONE',  ( -9.736236675707914401, 199.9851607334237542, 81.20113791807858661 ) ) ;
#10838=CARTESIAN_POINT ( 'NONE',  ( -8.062137200540920645, 212.9164362838581894, 96.80113791807858092 ) ) ;
#10842=CARTESIAN_POINT ( 'NONE',  ( 12.01549611932659367, 203.1486557965466773, 49.14886208192143613 ) ) ;
#10843=CARTESIAN_POINT ( 'NONE',  ( -10.00000000000000711, 206.9523078486584495, 71.49886208192144466 ) ) ;
#10844=CARTESIAN_POINT ( 'NONE',  ( -11.94915498584342295, 219.8409957184640291, 102.9933096652613642 ) ) ;
#10846=CARTESIAN_POINT ( 'NONE',  ( -8.062137200540920645, 212.9164362838581894, 12.80113791807856671 ) ) ;
#10848=CARTESIAN_POINT ( 'NONE',  ( 10.00000000000000711, 207.0476921513415220, 81.99886208192143044 ) ) ;
#10850=CARTESIAN_POINT ( 'NONE',  ( -8.062137200540920645, 212.9164362838581894, 99.80113791807858092 ) ) ;
#10853=CARTESIAN_POINT ( 'NONE',  ( 0.05014649552828262524, 198.5883022060938572, 58.74886208192143755 ) ) ;
#10858=CIRCLE ( 'NONE', #520, 0.9999999999999968914 ) ;
#10860=CARTESIAN_POINT ( 'NONE',  ( -6.444103211791042618, 211.7408657792732356, 54.80113791807857382 ) ) ;
#10862=DIRECTION ( 'NONE',  ( -5.782411586589351722E-16, 0.000000000000000000, -1.000000000000000000 ) ) ;
#10864=CARTESIAN_POINT ( 'NONE',  ( 6.500168698208244500, 202.3363017425938324, 34.29886208192144181 ) ) ;
#10865=CARTESIAN_POINT ( 'NONE',  ( -9.984503880673473830, 210.2968891136704315, 84.65113791807857524 ) ) ;
#10867=CARTESIAN_POINT ( 'NONE',  ( 8.118202686958039038, 212.8392687619912635, 61.70113791807857240 ) ) ;
#10870=CARTESIAN_POINT ( 'NONE',  ( 6.444103211791042618, 202.2591342207267644, 11.30113791807856671 ) ) ;
#10874=CARTESIAN_POINT ( 'NONE',  ( -7.375838497908182134, 217.2372850707499765, 42.95113791807857240 ) ) ;
#10876=CARTESIAN_POINT ( 'NONE',  ( -0.05014649552810635652, 196.4853777576173002, 98.75113791807854113 ) ) ;
#10878=CARTESIAN_POINT ( 'NONE',  ( 9.984503880673473830, 203.7031108863295401, 62.15113791807857524 ) ) ;
#10879=CARTESIAN_POINT ( 'NONE',  ( 7.375838497908012492, 217.2372850707501186, 18.54886208192143116 ) ) ;
#10880=CARTESIAN_POINT ( 'NONE',  ( 6.139770520408223575, 215.5359834540460611, 42.54886208192142760 ) ) ;
#10882=CARTESIAN_POINT ( 'NONE',  ( 7.375838497908181246, 196.7627149292499666, 71.45113791807854398 ) ) ;
#10884=CARTESIAN_POINT ( 'NONE',  ( 6.444103211791042618, 202.2591342207267644, 92.30113791807858092 ) ) ;
#10885=CARTESIAN_POINT ( 'NONE',  ( 0.05014649552828275708, 196.4853777576173002, 49.74886208192141623 ) ) ;
#10888=CARTESIAN_POINT ( 'NONE',  ( -9.680171189290716072, 199.9079932115567146, 50.19886208192144039 ) ) ;
#10894=CARTESIAN_POINT ( 'NONE',  ( -2.517493886308901807, 199.4062855549015012, 41.90113791807856813 ) ) ;
#10895=CARTESIAN_POINT ( 'NONE',  ( 8.062137200540822946, 212.9164362838583315, 24.69886208192143684 ) ) ;
#10901=CARTESIAN_POINT ( 'NONE',  ( 4.984841277089891776, 200.2242689037093726, 7.448862081921436840 ) ) ;
#10902=CARTESIAN_POINT ( 'NONE',  ( 6.139770520408368348, 198.4640165459539674, 50.45113791807857240 ) ) ;
#10904=( BOUNDED_CURVE ( )  B_SPLINE_CURVE ( 2, ( #23099, #15760, #22925, #12873, #269, #28382, #20376, #15590, #7431, #33488, #10157, #10663, #2662, #21039, #8109, #20540, #23266, #4869, #15430, #28034, #20708, #2317, #4695, #33320, #15257, #33661, #7607, #18162, #20881, #17812, #15085, #30942, #10337, #31109, #9990, #28556, #23435, #99, #10502, #31279, #18321, #28716, #5372, #26155, #2821, #13205, #25479, #23604, #5697, #18990, #8594, #759, #11490, #21204, #3307, #31762, #11321, #13535, #16086, #923, #13869, #29209, #21705, #31599, #6199, #21533, #2986, #1099, #18492, #29044, #11158, #14038, #3148, #26814, #21868, #23929, #8428, #16417, #3644, #592, #10987, #26479, #5860, #32262, #18654, #6025, #24435, #31923, #21366, #18814, #3477, #26644, #28875, #10829, #29380, #13691, #16258, #24254, #8264, #32096, #29545, #8758, #5531, #24092, #19147, #15922, #16587, #26979, #26320, #13366, #23762, #427, #14710, #6544, #9602, #22556, #24774, #24943, #32601, #1600, #6371, #9439, #11991, #12330, #27659, #8930, #17108, #1763, #30225, #19829, #14543, #25103, #27822, #32941, #1430, #6880, #27492, #16762, #4492, #22727, #1267, #25277, #3987, #14207, #22044, #9094, #24604, #14884, #12164, #17269, #11660, #32427, #1941, #27160, #27321, #4326, #14384, #30396, #3816, #6717, #19320, #29709, #7057, #11825, #19490, #22212, #29890, #19996, #16926, #17439, #9266, #19659, #30049, #4147, #22376, #32765, #26409, #30738, #33115, #17614, #20339, #16175, #12665, #10591, #7397, #31361, #13456, #23849, #524, #193, #13620, #21293, #13296, #17778, #25615, #18747, #3068, #28001, #5626, #2281, #15226, #10916, #8030, #28178, #4667, #31687, #3234, #4836, #23525, #31528, #29132, #20967, #18415, #16017, #28808, #8357, #5780, #5464, #15850, #26241, #2911, #33284, #348, #23688, #9780, #18582, #20164, #10749, #26564, #21129, #8197, #28967, #30561, #7223, #15051, #25446, #2121, #12503, #22892, #9951, #27410, #11739, #6630, #19073, #29300, #3397, #24186, #5951, #29972, #29806, #24520, #16341, #26735, #17016, #31848, #8682, #32351, #29462, #22126, #18905, #21790, #4070, #11083, #32516, #6114, #8511, #16510, #13791, #1352, #848, #21962, #6466, #11238, #24693, #21624, #9015, #32018, #16849, #26909, #24017, #3567, #16677, #681, #13957, #1018, #24350, #32182, #3896, #14292, #9189, #11413, #21464, #19579, #3738, #8842, #19242, #29637, #27242, #6284, #27074, #14127, #1177, #11573, #19404, #22465, #19744, #4746, #32856, #25187, #7484, #14633, #2029, #33375, #7140, #17360, #9519, #12416, #22632, #14458, #6798, #30478, #2200, #17524, #32681, #30819, #24854, #25030, #27913, #10049, #19906, #22811, #1517, #12582, #30305, #22300, #6972, #4235, #25532, #27568, #33202, #30652, #9689, #1682, #1855, #20426, #4583, #15137, #22975, #12075, #17869, #14970, #28265, #27746, #12245, #4409, #33020, #28084, #11914, #9348, #14794, #30140, #25358, #20083, #9865, #17185, #17696, #20248, #7319, #31153, #20755, #13548, #21253, #13092, #25873, #5422, #28766, #20930, #31646, #7654, #23482, #18209, #31323, #7820, #12922, #26200, #148, #4920, #30998, #7989, #10551, #28600, #15807, #18037, #18374, #15976, #2715, #15642, #2540, #2868, #5251, #8313, #26044, #13254, #23808, #10383, #23650, #10708, #23318, #5582, #18540, #309, #21087, #31490, #8158, #2370, #28922, #26369, #3029, #13414, #480, #18706, #10878, #15306, #25698, #12759, #23150, #33538, #10212, #20596, #28431, #5087, #15482, #24649, #32473, #21420, #13585, #11703, #808, #3523, #14250, #8801, #1315, #1140, #29597, #11037, #31806, #22088, #3196, #13746, #3692, #24142, #16804, #23978, #26866, #9141, #29093, #29758, #13916, #3355, #639, #19364, #11370, #5741, #8471, #24301, #8641, #21915, #11198, #26693, #11533, #24478, #32311, #6071, #8977, #18860, #27201, #32139, #29257, #16133, #26525, #5908, #16466, #21577, #27030, #19033, #16304, #31970, #29422, #3857, #970, #21750, #19198, #6247, #6423, #16634, #14083, #1983, #25318, #12374, #22770, #19699, #17145, #19867, #30607, #22420, #12543, #28042, #22934, #32644, #33163, #27708, #9826, #20207, #30440, #16969, #4703, #33329, #14421, #7272, #17654, #15093, #2160, #24990, #4369, #25488, #32979, #9644, #27365, #19538, #29932, #4032, #6586, #24814, #1477, #27865, #9307, #30093, #25143, #11872, #20040, #22257, #6760, #7100, #27531, #14592, #1641, #4193, #4539, #12032, #32811, #9477, #14751, #30263, #6925, #17317, #12205, #1809, #22592, #17480, #14930, #2670, #23273, #23442, #2827, #12714, #10001, #10166, #15597, #2497, #17819, #28564, #20548, #13052, #10345, #20888, #33670, #10669, #31449, #20385, #28220, #17999, #2993, #23108, #5212, #20716, #13211, #5047, #7615, #26161, #5379, #23610, #31116, #274, #33496, #8117, #107, #4878, #26327, #30777, #30953, #10509, #28390, #7947, #7778, #13372, #15439, #25835, #18498, #28883, #12880, #25999, #15266, #21047, #25658, #18169, #5539, #15766, #15929, #23769, #31286, #18329, #28723, #7439, #2326, #27166, #8936, #3821, #13544, #3649, #8599, #14044, #24440, #11327, #31605, #19326, #14213, #29051, #1104, #6205, #21875, #16767, #5867, #18996, #29714, #13875, #24259, #8273, #32269, #6377, #18660, #26986, #11497, #10838, #8765, #23937, #10994, #6033, #5704, #929, #436, #21212, #18821, #16092, #26652, #599, #26486, #21373, #32102, #16593, #31768, #3155, #8435, #19155, #29215, #16265, #3315, #13699, #24097, #26820, #765, #11163, #21538, #31928, #29385, #16424, #3483, #21712, #29551, #9444, #24781, #27665, #24949, #1769 ),
 .UNSPECIFIED., .F., .F. ) 
 B_SPLINE_CURVE_WITH_KNOTS ( ( 3, 2, 2, 2, 2, 2, 2, 2, 2, 2, 2, 2, 2, 2, 2, 2, 2, 2, 2, 2, 2, 2, 2, 2, 2, 2, 2, 2, 2, 2, 2, 2, 2, 2, 2, 2, 2, 2, 2, 2, 2, 2, 2, 2, 2, 2, 2, 2, 2, 2, 2, 2, 2, 2, 2, 2, 2, 2, 2, 2, 2, 2, 2, 2, 2, 2, 2, 2, 2, 2, 2, 2, 2, 2, 2, 2, 2, 2, 2, 2, 2, 2, 2, 2, 2, 2, 2, 2, 2, 2, 2, 2, 2, 2, 2, 2, 2, 2, 2, 2, 2, 2, 2, 2, 2, 2, 2, 2, 2, 2, 2, 2, 2, 2, 2, 2, 2, 2, 2, 2, 2, 2, 2, 2, 2, 2, 2, 2, 2, 2, 2, 2, 2, 2, 2, 2, 2, 2, 2, 2, 2, 2, 2, 2, 2, 2, 2, 2, 2, 2, 2, 2, 2, 2, 2, 2, 2, 2, 2, 2, 2, 2, 2, 2, 2, 2, 2, 2, 2, 2, 2, 2, 2, 2, 2, 2, 2, 2, 2, 2, 2, 2, 2, 2, 2, 2, 2, 2, 2, 2, 2, 2, 2, 2, 2, 2, 2, 2, 2, 2, 2, 2, 2, 2, 2, 2, 2, 2, 2, 2, 2, 2, 2, 2, 2, 2, 2, 2, 2, 2, 2, 2, 2, 2, 2, 2, 2, 2, 2, 2, 2, 2, 2, 2, 2, 2, 2, 2, 2, 2, 2, 2, 2, 2, 2, 2, 2, 2, 2, 2, 2, 2, 2, 2, 2, 2, 2, 2, 2, 2, 2, 2, 2, 2, 2, 2, 2, 2, 2, 2, 2, 2, 2, 2, 2, 2, 2, 2, 2, 2, 2, 2, 2, 2, 2, 2, 2, 2, 2, 2, 2, 2, 2, 2, 2, 2, 2, 2, 2, 2, 2, 2, 2, 2, 2, 2, 2, 2, 2, 2, 2, 2, 2, 2, 2, 2, 2, 2, 2, 2, 2, 2, 2, 2, 2, 2, 2, 2, 2, 2, 2, 2, 2, 2, 2, 2, 2, 2, 2, 2, 2, 2, 2, 2, 2, 2, 3 ),
 ( 0.000000000000000000, 0.002857142857142857140, 0.005714285714285714281, 0.008571428571428571855, 0.01142857142857142856, 0.01428571428571428527, 0.01714285714285714371, 0.02000000000000000042, 0.02285714285714285712, 0.02571428571428571383, 0.02857142857142857054, 0.03142857142857143071, 0.03428571428571428742, 0.03714285714285714413, 0.04000000000000000083, 0.04285714285714285754, 0.04571428571428571425, 0.04857142857142857095, 0.05142857142857142766, 0.05428571428571428437, 0.05714285714285714107, 0.05999999999999999778, 0.06285714285714286143, 0.06571428571428571119, 0.06857142857142857484, 0.07142857142857142461, 0.07428571428571428825, 0.07714285714285713802, 0.08000000000000000167, 0.08285714285714285143, 0.08571428571428571508, 0.08857142857142856485, 0.09142857142857142849, 0.09428571428571429214, 0.09714285714285714191, 0.1000000000000000056, 0.1028571428571428553, 0.1057142857142857190, 0.1085714285714285687, 0.1114285714285714324, 0.1142857142857142821, 0.1171428571428571458, 0.1199999999999999956, 0.1228571428571428592, 0.1257142857142857229, 0.1285714285714285587, 0.1314285714285714224, 0.1342857142857142860, 0.1371428571428571497, 0.1400000000000000133, 0.1428571428571428492, 0.1457142857142857129, 0.1485714285714285765, 0.1514285714285714401, 0.1542857142857142760, 0.1571428571428571397, 0.1600000000000000033, 0.1628571428571428670, 0.1657142857142857029, 0.1685714285714285665, 0.1714285714285714302, 0.1742857142857142938, 0.1771428571428571297, 0.1799999999999999933, 0.1828571428571428570, 0.1857142857142857206, 0.1885714285714285843, 0.1914285714285714202, 0.1942857142857142838, 0.1971428571428571475, 0.2000000000000000111, 0.2028571428571428470, 0.2057142857142857106, 0.2085714285714285743, 0.2114285714285714379, 0.2142857142857142738, 0.2171428571428571375, 0.2200000000000000011, 0.2228571428571428648, 0.2257142857142857006, 0.2285714285714285643, 0.2314285714285714279, 0.2342857142857142916, 0.2371428571428571552, 0.2399999999999999911, 0.2428571428571428548, 0.2457142857142857184, 0.2485714285714285821, 0.2514285714285714457, 0.2542857142857142816, 0.2571428571428571175, 0.2600000000000000089, 0.2628571428571428448, 0.2657142857142857362, 0.2685714285714285721, 0.2714285714285714080, 0.2742857142857142994, 0.2771428571428571352, 0.2800000000000000266, 0.2828571428571428625, 0.2857142857142856984, 0.2885714285714285898, 0.2914285714285714257, 0.2942857142857142616, 0.2971428571428571530, 0.2999999999999999889, 0.3028571428571428803, 0.3057142857142857162, 0.3085714285714285521, 0.3114285714285714435, 0.3142857142857142794, 0.3171428571428571153, 0.3200000000000000067, 0.3228571428571428426, 0.3257142857142857340, 0.3285714285714285698, 0.3314285714285714057, 0.3342857142857142971, 0.3371428571428571330, 0.3400000000000000244, 0.3428571428571428603, 0.3457142857142856962, 0.3485714285714285876, 0.3514285714285714235, 0.3542857142857142594, 0.3571428571428571508, 0.3599999999999999867, 0.3628571428571428781, 0.3657142857142857140, 0.3685714285714285499, 0.3714285714285714413, 0.3742857142857142771, 0.3771428571428571686, 0.3800000000000000044, 0.3828571428571428403, 0.3857142857142857317, 0.3885714285714285676, 0.3914285714285714035, 0.3942857142857142949, 0.3971428571428571308, 0.4000000000000000222, 0.4028571428571428581, 0.4057142857142856940, 0.4085714285714285854, 0.4114285714285714213, 0.4142857142857143127, 0.4171428571428571486, 0.4199999999999999845, 0.4228571428571428759, 0.4257142857142857117, 0.4285714285714285476, 0.4314285714285714390, 0.4342857142857142749, 0.4371428571428571663, 0.4400000000000000022, 0.4428571428571428381, 0.4457142857142857295, 0.4485714285714285654, 0.4514285714285714013, 0.4542857142857142927, 0.4571428571428571286, 0.4600000000000000200, 0.4628571428571428559, 0.4657142857142856918, 0.4685714285714285832, 0.4714285714285714191, 0.4742857142857143105, 0.4771428571428571463, 0.4799999999999999822, 0.4828571428571428736, 0.4857142857142857095, 0.4885714285714285454, 0.4914285714285714368, 0.4942857142857142727, 0.4971428571428571641, 0.5000000000000000000, 0.5028571428571428914, 0.5057142857142856718, 0.5085714285714285632, 0.5114285714285714546, 0.5142857142857142350, 0.5171428571428571264, 0.5200000000000000178, 0.5228571428571429092, 0.5257142857142856895, 0.5285714285714285809, 0.5314285714285714723, 0.5342857142857142527, 0.5371428571428571441, 0.5400000000000000355, 0.5428571428571428159, 0.5457142857142857073, 0.5485714285714285987, 0.5514285714285713791, 0.5542857142857142705, 0.5571428571428571619, 0.5600000000000000533, 0.5628571428571428337, 0.5657142857142857251, 0.5685714285714286165, 0.5714285714285713969, 0.5742857142857142883, 0.5771428571428571797, 0.5799999999999999600, 0.5828571428571428514, 0.5857142857142857428, 0.5885714285714285232, 0.5914285714285714146, 0.5942857142857143060, 0.5971428571428571974, 0.5999999999999999778, 0.6028571428571428692, 0.6057142857142857606, 0.6085714285714285410, 0.6114285714285714324, 0.6142857142857143238, 0.6171428571428571042, 0.6199999999999999956, 0.6228571428571428870, 0.6257142857142856673, 0.6285714285714285587, 0.6314285714285714501, 0.6342857142857142305, 0.6371428571428571219, 0.6400000000000000133, 0.6428571428571429047, 0.6457142857142856851, 0.6485714285714285765, 0.6514285714285714679, 0.6542857142857142483, 0.6571428571428571397, 0.6600000000000000311, 0.6628571428571428115, 0.6657142857142857029, 0.6685714285714285943, 0.6714285714285713746, 0.6742857142857142660, 0.6771428571428571574, 0.6800000000000000488, 0.6828571428571428292, 0.6857142857142857206, 0.6885714285714286120, 0.6914285714285713924, 0.6942857142857142838, 0.6971428571428571752, 0.6999999999999999556, 0.7028571428571428470, 0.7057142857142857384, 0.7085714285714285188, 0.7114285714285714102, 0.7142857142857143016, 0.7171428571428571930, 0.7199999999999999734, 0.7228571428571428648, 0.7257142857142857562, 0.7285714285714285365, 0.7314285714285714279, 0.7342857142857143193, 0.7371428571428570997, 0.7399999999999999911, 0.7428571428571428825, 0.7457142857142856629, 0.7485714285714285543, 0.7514285714285714457, 0.7542857142857143371, 0.7571428571428571175, 0.7600000000000000089, 0.7628571428571429003, 0.7657142857142856807, 0.7685714285714285721, 0.7714285714285714635, 0.7742857142857142438, 0.7771428571428571352, 0.7800000000000000266, 0.7828571428571428070, 0.7857142857142856984, 0.7885714285714285898, 0.7914285714285714812, 0.7942857142857142616, 0.7971428571428571530, 0.8000000000000000444, 0.8028571428571428248, 0.8057142857142857162, 0.8085714285714286076, 0.8114285714285713880, 0.8142857142857142794, 0.8171428571428571708, 0.8199999999999999512, 0.8228571428571428426, 0.8257142857142857340, 0.8285714285714286254, 0.8314285714285714057, 0.8342857142857142971, 0.8371428571428571885, 0.8399999999999999689, 0.8428571428571428603, 0.8457142857142857517, 0.8485714285714285321, 0.8514285714285714235, 0.8542857142857143149, 0.8571428571428570953, 0.8599999999999999867, 0.8628571428571428781, 0.8657142857142857695, 0.8685714285714285499, 0.8714285714285714413, 0.8742857142857143327, 0.8771428571428571130, 0.8800000000000000044, 0.8828571428571428958, 0.8857142857142856762, 0.8885714285714285676, 0.8914285714285714590, 0.8942857142857142394, 0.8971428571428571308, 0.9000000000000000222, 0.9028571428571428026, 0.9057142857142856940, 0.9085714285714285854, 0.9114285714285714768, 0.9142857142857142572, 0.9171428571428571486, 0.9200000000000000400, 0.9228571428571428203, 0.9257142857142857117, 0.9285714285714286031, 0.9314285714285713835, 0.9342857142857142749, 0.9371428571428571663, 0.9399999999999999467, 0.9428571428571428381, 0.9457142857142857295, 0.9485714285714286209, 0.9514285714285714013, 0.9542857142857142927, 0.9571428571428571841, 0.9599999999999999645, 0.9628571428571428559, 0.9657142857142857473, 0.9685714285714285277, 0.9714285714285714191, 0.9742857142857143105, 0.9771428571428570908, 0.9799999999999999822, 0.9828571428571428736, 0.9857142857142857650, 0.9860665758260036551 ),
 .UNSPECIFIED. ) 
 CURVE ( )  GEOMETRIC_REPRESENTATION_ITEM ( )  RATIONAL_B_SPLINE_CURVE ( ( 1.000000000000000000, 0.9510565162951535312, 1.000000000000000000, 0.9510565162951535312, 1.000000000000000000, 0.9510565162951535312, 1.000000000000000000, 0.9510565162951535312, 1.000000000000000000, 0.9510565162951535312, 1.000000000000000000, 0.9510565162951535312, 1.000000000000000000, 0.9510565162951535312, 1.000000000000000000, 0.9510565162951535312, 1.000000000000000000, 0.9510565162951535312, 1.000000000000000000, 0.9510565162951535312, 1.000000000000000000, 0.9510565162951535312, 1.000000000000000000, 0.9510565162951535312, 1.000000000000000000, 0.9510565162951535312, 1.000000000000000000, 0.9510565162951535312, 1.000000000000000000, 0.9510565162951535312, 1.000000000000000000, 0.9510565162951535312, 1.000000000000000000, 0.9510565162951535312, 1.000000000000000000, 0.9510565162951535312, 1.000000000000000000, 0.9510565162951535312, 1.000000000000000000, 0.9510565162951535312, 1.000000000000000000, 0.9510565162951535312, 1.000000000000000000, 0.9510565162951535312, 1.000000000000000000, 0.9510565162951535312, 1.000000000000000000, 0.9510565162951535312, 1.000000000000000000, 0.9510565162951535312, 1.000000000000000000, 0.9510565162951535312, 1.000000000000000000, 0.9510565162951535312, 1.000000000000000000, 0.9510565162951535312, 1.000000000000000000, 0.9510565162951535312, 1.000000000000000000, 0.9510565162951535312, 1.000000000000000000, 0.9510565162951535312, 1.000000000000000000, 0.9510565162951535312, 1.000000000000000000, 0.9510565162951535312, 1.000000000000000000, 0.9510565162951535312, 1.000000000000000000, 0.9510565162951535312, 1.000000000000000000, 0.9510565162951535312, 1.000000000000000000, 0.9510565162951535312, 1.000000000000000000, 0.9510565162951535312, 1.000000000000000000, 0.9510565162951535312, 1.000000000000000000, 0.9510565162951535312, 1.000000000000000000, 0.9510565162951535312, 1.000000000000000000, 0.9510565162951535312, 1.000000000000000000, 0.9510565162951535312, 1.000000000000000000, 0.9510565162951535312, 1.000000000000000000, 0.9510565162951535312, 1.000000000000000000, 0.9510565162951535312, 1.000000000000000000, 0.9510565162951535312, 1.000000000000000000, 0.9510565162951535312, 1.000000000000000000, 0.9510565162951535312, 1.000000000000000000, 0.9510565162951535312, 1.000000000000000000, 0.9510565162951535312, 1.000000000000000000, 0.9510565162951535312, 1.000000000000000000, 0.9510565162951535312, 1.000000000000000000, 0.9510565162951535312, 1.000000000000000000, 0.9510565162951535312, 1.000000000000000000, 0.9510565162951535312, 1.000000000000000000, 0.9510565162951535312, 1.000000000000000000, 0.9510565162951535312, 1.000000000000000000, 0.9510565162951535312, 1.000000000000000000, 0.9510565162951535312, 1.000000000000000000, 0.9510565162951535312, 1.000000000000000000, 0.9510565162951535312, 1.000000000000000000, 0.9510565162951535312, 1.000000000000000000, 0.9510565162951535312, 1.000000000000000000, 0.9510565162951535312, 1.000000000000000000, 0.9510565162951535312, 1.000000000000000000, 0.9510565162951535312, 1.000000000000000000, 0.9510565162951535312, 1.000000000000000000, 0.9510565162951535312, 1.000000000000000000, 0.9510565162951535312, 1.000000000000000000, 0.9510565162951535312, 1.000000000000000000, 0.9510565162951535312, 1.000000000000000000, 0.9510565162951535312, 1.000000000000000000, 0.9510565162951535312, 1.000000000000000000, 0.9510565162951535312, 1.000000000000000000, 0.9510565162951535312, 1.000000000000000000, 0.9510565162951535312, 1.000000000000000000, 0.9510565162951535312, 1.000000000000000000, 0.9510565162951535312, 1.000000000000000000, 0.9510565162951535312, 1.000000000000000000, 0.9510565162951535312, 1.000000000000000000, 0.9510565162951535312, 1.000000000000000000, 0.9510565162951535312, 1.000000000000000000, 0.9510565162951535312, 1.000000000000000000, 0.9510565162951535312, 1.000000000000000000, 0.9510565162951535312, 1.000000000000000000, 0.9510565162951535312, 1.000000000000000000, 0.9510565162951535312, 1.000000000000000000, 0.9510565162951535312, 1.000000000000000000, 0.9510565162951535312, 1.000000000000000000, 0.9510565162951535312, 1.000000000000000000, 0.9510565162951535312, 1.000000000000000000, 0.9510565162951535312, 1.000000000000000000, 0.9510565162951535312, 1.000000000000000000, 0.9510565162951535312, 1.000000000000000000, 0.9510565162951535312, 1.000000000000000000, 0.9510565162951535312, 1.000000000000000000, 0.9510565162951535312, 1.000000000000000000, 0.9510565162951535312, 1.000000000000000000, 0.9510565162951535312, 1.000000000000000000, 0.9510565162951535312, 1.000000000000000000, 0.9510565162951535312, 1.000000000000000000, 0.9510565162951535312, 1.000000000000000000, 0.9510565162951535312, 1.000000000000000000, 0.9510565162951535312, 1.000000000000000000, 0.9510565162951535312, 1.000000000000000000, 0.9510565162951535312, 1.000000000000000000, 0.9510565162951535312, 1.000000000000000000, 0.9510565162951535312, 1.000000000000000000, 0.9510565162951535312, 1.000000000000000000, 0.9510565162951535312, 1.000000000000000000, 0.9510565162951535312, 1.000000000000000000, 0.9510565162951535312, 1.000000000000000000, 0.9510565162951535312, 1.000000000000000000, 0.9510565162951535312, 1.000000000000000000, 0.9510565162951535312, 1.000000000000000000, 0.9510565162951535312, 1.000000000000000000, 0.9510565162951535312, 1.000000000000000000, 0.9510565162951535312, 1.000000000000000000, 0.9510565162951535312, 1.000000000000000000, 0.9510565162951535312, 1.000000000000000000, 0.9510565162951535312, 1.000000000000000000, 0.9510565162951535312, 1.000000000000000000, 0.9510565162951535312, 1.000000000000000000, 0.9510565162951535312, 1.000000000000000000, 0.9510565162951535312, 1.000000000000000000, 0.9510565162951535312, 1.000000000000000000, 0.9510565162951535312, 1.000000000000000000, 0.9510565162951535312, 1.000000000000000000, 0.9510565162951535312, 1.000000000000000000, 0.9510565162951535312, 1.000000000000000000, 0.9510565162951535312, 1.000000000000000000, 0.9510565162951535312, 1.000000000000000000, 0.9510565162951535312, 1.000000000000000000, 0.9510565162951535312, 1.000000000000000000, 0.9510565162951535312, 1.000000000000000000, 0.9510565162951535312, 1.000000000000000000, 0.9510565162951535312, 1.000000000000000000, 0.9510565162951535312, 1.000000000000000000, 0.9510565162951535312, 1.000000000000000000, 0.9510565162951535312, 1.000000000000000000, 0.9510565162951535312, 1.000000000000000000, 0.9510565162951535312, 1.000000000000000000, 0.9510565162951535312, 1.000000000000000000, 0.9510565162951535312, 1.000000000000000000, 0.9510565162951535312, 1.000000000000000000, 0.9510565162951535312, 1.000000000000000000, 0.9510565162951535312, 1.000000000000000000, 0.9510565162951535312, 1.000000000000000000, 0.9510565162951535312, 1.000000000000000000, 0.9510565162951535312, 1.000000000000000000, 0.9510565162951535312, 1.000000000000000000, 0.9510565162951535312, 1.000000000000000000, 0.9510565162951535312, 1.000000000000000000, 0.9510565162951535312, 1.000000000000000000, 0.9510565162951535312, 1.000000000000000000, 0.9510565162951535312, 1.000000000000000000, 0.9510565162951535312, 1.000000000000000000, 0.9510565162951535312, 1.000000000000000000, 0.9510565162951535312, 1.000000000000000000, 0.9510565162951535312, 1.000000000000000000, 0.9510565162951535312, 1.000000000000000000, 0.9510565162951535312, 1.000000000000000000, 0.9510565162951535312, 1.000000000000000000, 0.9510565162951535312, 1.000000000000000000, 0.9510565162951535312, 1.000000000000000000, 0.9510565162951535312, 1.000000000000000000, 0.9510565162951535312, 1.000000000000000000, 0.9510565162951535312, 1.000000000000000000, 0.9510565162951535312, 1.000000000000000000, 0.9510565162951535312, 1.000000000000000000, 0.9510565162951535312, 1.000000000000000000, 0.9510565162951535312, 1.000000000000000000, 0.9510565162951535312, 1.000000000000000000, 0.9510565162951535312, 1.000000000000000000, 0.9510565162951535312, 1.000000000000000000, 0.9510565162951535312, 1.000000000000000000, 0.9510565162951535312, 1.000000000000000000, 0.9510565162951535312, 1.000000000000000000, 0.9510565162951535312, 1.000000000000000000, 0.9510565162951535312, 1.000000000000000000, 0.9510565162951535312, 1.000000000000000000, 0.9510565162951535312, 1.000000000000000000, 0.9510565162951535312, 1.000000000000000000, 0.9510565162951535312, 1.000000000000000000, 0.9510565162951535312, 1.000000000000000000, 0.9510565162951535312, 1.000000000000000000, 0.9510565162951535312, 1.000000000000000000, 0.9510565162951535312, 1.000000000000000000, 0.9510565162951535312, 1.000000000000000000, 0.9510565162951535312, 1.000000000000000000, 0.9510565162951535312, 1.000000000000000000, 0.9510565162951535312, 1.000000000000000000, 0.9510565162951535312, 1.000000000000000000, 0.9510565162951535312, 1.000000000000000000, 0.9510565162951535312, 1.000000000000000000, 0.9510565162951535312, 1.000000000000000000, 0.9510565162951535312, 1.000000000000000000, 0.9510565162951535312, 1.000000000000000000, 0.9510565162951535312, 1.000000000000000000, 0.9510565162951535312, 1.000000000000000000, 0.9510565162951535312, 1.000000000000000000, 0.9510565162951535312, 1.000000000000000000, 0.9510565162951535312, 1.000000000000000000, 0.9510565162951535312, 1.000000000000000000, 0.9510565162951535312, 1.000000000000000000, 0.9510565162951535312, 1.000000000000000000, 0.9510565162951535312, 1.000000000000000000, 0.9510565162951535312, 1.000000000000000000, 0.9510565162951535312, 1.000000000000000000, 0.9510565162951535312, 1.000000000000000000, 0.9510565162951535312, 1.000000000000000000, 0.9510565162951535312, 1.000000000000000000, 0.9510565162951535312, 1.000000000000000000, 0.9510565162951535312, 1.000000000000000000, 0.9510565162951535312, 1.000000000000000000, 0.9510565162951535312, 1.000000000000000000, 0.9510565162951535312, 1.000000000000000000, 0.9510565162951535312, 1.000000000000000000, 0.9510565162951535312, 1.000000000000000000, 0.9510565162951535312, 1.000000000000000000, 0.9510565162951535312, 1.000000000000000000, 0.9510565162951535312, 1.000000000000000000, 0.9510565162951535312, 1.000000000000000000, 0.9510565162951535312, 1.000000000000000000, 0.9510565162951535312, 1.000000000000000000, 0.9510565162951535312, 1.000000000000000000, 0.9510565162951535312, 1.000000000000000000, 0.9510565162951535312, 1.000000000000000000, 0.9510565162951535312, 1.000000000000000000, 0.9510565162951535312, 1.000000000000000000, 0.9510565162951535312, 1.000000000000000000, 0.9510565162951535312, 1.000000000000000000, 0.9510565162951535312, 1.000000000000000000, 0.9510565162951535312, 1.000000000000000000, 0.9510565162951535312, 1.000000000000000000, 0.9510565162951535312, 1.000000000000000000, 0.9510565162951535312, 1.000000000000000000, 0.9510565162951535312, 1.000000000000000000, 0.9510565162951535312, 1.000000000000000000, 0.9510565162951535312, 1.000000000000000000, 0.9510565162951535312, 1.000000000000000000, 0.9510565162951535312, 1.000000000000000000, 0.9510565162951535312, 1.000000000000000000, 0.9510565162951535312, 1.000000000000000000, 0.9510565162951535312, 1.000000000000000000, 0.9510565162951535312, 1.000000000000000000, 0.9510565162951535312, 1.000000000000000000, 0.9510565162951535312, 1.000000000000000000, 0.9510565162951535312, 1.000000000000000000, 0.9510565162951535312, 1.000000000000000000, 0.9510565162951535312, 1.000000000000000000, 0.9510565162951535312, 1.000000000000000000, 0.9510565162951535312, 1.000000000000000000, 0.9510565162951535312, 1.000000000000000000, 0.9510565162951535312, 1.000000000000000000, 0.9510565162951535312, 1.000000000000000000, 0.9510565162951535312, 1.000000000000000000, 0.9510565162951535312, 1.000000000000000000, 0.9510565162951535312, 1.000000000000000000, 0.9510565162951535312, 1.000000000000000000, 0.9510565162951535312, 1.000000000000000000, 0.9510565162951535312, 1.000000000000000000, 0.9510565162951535312, 1.000000000000000000, 0.9510565162951535312, 1.000000000000000000, 0.9510565162951535312, 1.000000000000000000, 0.9510565162951535312, 1.000000000000000000, 0.9510565162951535312, 1.000000000000000000, 0.9510565162951535312, 1.000000000000000000, 0.9510565162951535312, 1.000000000000000000, 0.9510565162951535312, 1.000000000000000000, 0.9510565162951535312, 1.000000000000000000, 0.9510565162951535312, 1.000000000000000000, 0.9510565162951535312, 1.000000000000000000, 0.9510565162951535312, 1.000000000000000000, 0.9510565162951535312, 1.000000000000000000, 0.9510565162951535312, 1.000000000000000000, 0.9510565162951535312, 1.000000000000000000, 0.9510565162951535312, 1.000000000000000000, 0.9510565162951535312, 1.000000000000000000, 0.9510565162951535312, 1.000000000000000000, 0.9510565162951535312, 1.000000000000000000, 0.9510565162951535312, 1.000000000000000000, 0.9510565162951535312, 1.000000000000000000, 0.9510565162951535312, 1.000000000000000000, 0.9510565162951535312, 1.000000000000000000, 0.9510565162951535312, 1.000000000000000000, 0.9510565162951535312, 1.000000000000000000, 0.9510565162951535312, 1.000000000000000000, 0.9510565162951535312, 1.000000000000000000, 0.9510565162951535312, 1.000000000000000000, 0.9510565162951535312, 1.000000000000000000, 0.9510565162951535312, 1.000000000000000000, 0.9510565162951535312, 1.000000000000000000, 0.9510565162951535312, 1.000000000000000000, 0.9510565162951535312, 1.000000000000000000, 0.9510565162951535312, 1.000000000000000000, 0.9510565162951535312, 1.000000000000000000, 0.9510565162951535312, 1.000000000000000000, 0.9510565162951535312, 1.000000000000000000, 0.9510565162951535312, 1.000000000000000000, 0.9510565162951535312, 1.000000000000000000, 0.9510565162951535312, 1.000000000000000000, 0.9510565162951535312, 1.000000000000000000, 0.9510565162951535312, 1.000000000000000000, 0.9510565162951535312, 1.000000000000000000, 0.9510565162951535312, 1.000000000000000000, 0.9510565162951535312, 1.000000000000000000, 0.9510565162951535312, 1.000000000000000000, 0.9510565162951535312, 1.000000000000000000, 0.9510565162951535312, 1.000000000000000000, 0.9510565162951535312, 1.000000000000000000, 0.9510565162951535312, 1.000000000000000000, 0.9510565162951535312, 1.000000000000000000, 0.9510565162951535312, 1.000000000000000000, 0.9510565162951535312, 1.000000000000000000, 0.9510565162951535312, 1.000000000000000000, 0.9510565162951535312, 1.000000000000000000, 0.9510565162951535312, 1.000000000000000000, 0.9510565162951535312, 1.000000000000000000, 0.9510565162951535312, 1.000000000000000000, 0.9510565162951535312, 1.000000000000000000, 0.9510565162951535312, 1.000000000000000000, 0.9510565162951535312, 1.000000000000000000, 0.9510565162951535312, 1.000000000000000000, 0.9510565162951535312, 1.000000000000000000, 0.9510565162951535312, 1.000000000000000000, 0.9510565162951535312, 1.000000000000000000, 0.9510565162951535312, 1.000000000000000000, 0.9510565162951535312, 1.000000000000000000, 0.9510565162951535312, 1.000000000000000000, 0.9510565162951535312, 1.000000000000000000, 0.9510565162951535312, 1.000000000000000000, 0.9510565162951535312, 1.000000000000000000, 0.9510565162951535312, 1.000000000000000000, 0.9510565162951535312, 1.000000000000000000, 0.9510565162951535312, 1.000000000000000000, 0.9510565162951535312, 1.000000000000000000, 0.9510565162951535312, 1.000000000000000000, 0.9510565162951535312, 1.000000000000000000, 0.9510565162951535312, 1.000000000000000000, 0.9510565162951535312, 1.000000000000000000, 0.9510565162951535312, 1.000000000000000000, 0.9510565162951535312, 1.000000000000000000, 0.9510565162951535312, 1.000000000000000000, 1.000000000000000000, 1.000000000000000000 ) ) 
 REPRESENTATION_ITEM ( '' )  );
#10905=CARTESIAN_POINT ( 'NONE',  ( -10.00000000000000711, 207.0476921513413515, 39.50113791807856956 ) ) ;
#10908=CARTESIAN_POINT ( 'NONE',  ( 6.444103211790928043, 211.7408657792734061, 90.69886208192143329 ) ) ;
#10912=CARTESIAN_POINT ( 'NONE',  ( -0.05014649552807705357, 194.3824533091408000, 5.751137918078564226 ) ) ;
#10915=CARTESIAN_POINT ( 'NONE',  ( -10.00000000000000711, 207.0476921513413515, 57.50113791807856956 ) ) ;
#10916=CARTESIAN_POINT ( 'NONE',  ( 9.984503880673473830, 203.7031108863295401, 29.15113791807856458 ) ) ;
#10923=CARTESIAN_POINT ( 'NONE',  ( 9.680171189290831535, 199.9079932115568852, 38.30113791807856671 ) ) ;
#10924=DIRECTION ( 'NONE',  ( -0.5526942671207061286, -0.1536855300543007730, -0.8190908404712107238 ) ) ;
#10926=CARTESIAN_POINT ( 'NONE',  ( -3.044812012439970683, 197.4746971517856196, 25.89886208192143613 ) ) ;
#10929=CARTESIAN_POINT ( 'NONE',  ( 0.05014649552810505201, 217.5146222423826714, 82.25113791807858377 ) ) ;
#10930=ORIENTED_EDGE ( 'NONE', *, *, #5398, .T. ) ;
#10934=CARTESIAN_POINT ( 'NONE',  ( -4.984841277089726574, 200.2242689037092305, 15.05113791807856849 ) ) ;
#10936=CARTESIAN_POINT ( 'NONE',  ( -7.375838497908014268, 196.7627149292498530, 101.0488620819214276 ) ) ;
#10943=CARTESIAN_POINT ( 'NONE',  ( -6.139770520408224463, 198.4640165459539389, 83.04886208192144181 ) ) ;
#10945=CARTESIAN_POINT ( 'NONE',  ( 3.044812012440130555, 197.4746971517856764, 20.60113791807856742 ) ) ;
#10950=CARTESIAN_POINT ( 'NONE',  ( 9.984503880673470277, 203.7031108863295401, 83.15113791807853261 ) ) ;
#10953=CARTESIAN_POINT ( 'NONE',  ( -9.736236675708031640, 214.0148392665760753, 98.79886208192142760 ) ) ;
#10963=CARTESIAN_POINT ( 'NONE',  ( 3.135527875058981895, 197.5041725223112792, 97.59886208192143897 ) ) ;
#10964=CARTESIAN_POINT ( 'NONE',  ( -3.662846001189865142, 195.5725841191952838, 28.89886208192143613 ) ) ;
#10966=CARTESIAN_POINT ( 'NONE',  ( -10.00000000000000711, 207.0476921513413515, 48.50113791807856956 ) ) ;
#10968=CARTESIAN_POINT ( 'NONE',  ( -10.10169002831358576, 228.2744804605295315, 105.4832055762869061 ) ) ;
#10972=CARTESIAN_POINT ( 'NONE',  ( -6.500168698208244500, 211.6636982574061676, 86.79886208192142760 ) ) ;
#10973=CARTESIAN_POINT ( 'NONE',  ( 2.517493886308900919, 214.5937144450984420, 28.40113791807856813 ) ) ;
#10979=CARTESIAN_POINT ( 'NONE',  ( -2.426778023690262742, 214.6231898156240163, 94.10113791807857808 ) ) ;
#10983=CARTESIAN_POINT ( 'NONE',  ( 7.984503880673422316, 209.6470497212048372, 72.84886208192143897 ) ) ;
#10987=CARTESIAN_POINT ( 'NONE',  ( 10.00000000000000711, 206.9523078486586201, 11.00113791807856600 ) ) ;
#10992=CARTESIAN_POINT ( 'NONE',  ( 7.375838497908181246, 196.7627149292499666, 74.45113791807855819 ) ) ;
#10994=CARTESIAN_POINT ( 'NONE',  ( 0.05014649552810506589, 217.5146222423826714, 97.25113791807855534 ) ) ;
#10998=CARTESIAN_POINT ( 'NONE',  ( -7.375838497908014268, 196.7627149292498530, 59.04886208192144181 ) ) ;
#10999=CARTESIAN_POINT ( 'NONE',  ( -0.05014649552828402690, 217.5146222423826714, 63.24886208192144466 ) ) ;
#11000=CARTESIAN_POINT ( 'NONE',  ( -11.98450388067341876, 203.0532714938636047, 2.348862081921434530 ) ) ;
#11002=CARTESIAN_POINT ( 'NONE',  ( 10.00000000000000711, 206.9523078486586201, 11.00113791807856600 ) ) ;
#11003=CARTESIAN_POINT ( 'NONE',  ( 10.00000000000000711, 207.0476921513415220, 78.99886208192144466 ) ) ;
#11010=CARTESIAN_POINT ( 'NONE',  ( 6.444103211790928043, 211.7408657792734061, 63.69886208192144039 ) ) ;
#11012=VERTEX_POINT ( 'NONE', #12152 ) ;
#11021=CARTESIAN_POINT ( 'NONE',  ( -6.444103211791042618, 211.7408657792732356, 72.80113791807858092 ) ) ;
#11025=CARTESIAN_POINT ( 'NONE',  ( 4.903702542908435547, 213.8346818373419751, 48.54886208192144181 ) ) ;
#11026=CARTESIAN_POINT ( 'NONE',  ( 8.062137200540920645, 201.0835637161417822, 80.30113791807858092 ) ) ;
#11027=CARTESIAN_POINT ( 'NONE',  ( 3.135527875058820690, 216.4958274776887492, 64.40113791807857524 ) ) ;
#11030=CARTESIAN_POINT ( 'NONE',  ( -4.903702542908602524, 213.8346818373418898, 21.95113791807856884 ) ) ;
#11034=CARTESIAN_POINT ( 'NONE',  ( -0.05014649552807705357, 194.3824533091408000, 44.75113791807856956 ) ) ;
#11036=CARTESIAN_POINT ( 'NONE',  ( 8.118202686958039038, 212.8392687619912635, 94.70113791807857240 ) ) ;
#11037=CARTESIAN_POINT ( 'NONE',  ( 3.044812012440130555, 197.4746971517856764, 65.60113791807857808 ) ) ;
#11038=CARTESIAN_POINT ( 'NONE',  ( 3.753561863808876797, 195.6020594897209719, 37.59886208192143187 ) ) ;
#11039=CARTESIAN_POINT ( 'NONE',  ( 6.220909254589680693, 198.5229672870052582, 40.44886208192143329 ) ) ;
#11042=CARTESIAN_POINT ( 'NONE',  ( 9.736236675707914401, 214.0148392665762458, 79.70113791807857240 ) ) ;
#11043=CARTESIAN_POINT ( 'NONE',  ( -2.517493886308901807, 199.4062855549015012, 86.90113791807857524 ) ) ;
#11044=AXIS2_PLACEMENT_3D ( 'NONE', #22230, #779, #19007 ) ;
#11045=CARTESIAN_POINT ( 'NONE',  ( 10.01549611932659545, 203.7984951890123853, 52.14886208192142192 ) ) ;
#11048=CARTESIAN_POINT ( 'NONE',  ( -3.753561863808878130, 218.3979405102790281, 66.09886208192142476 ) ) ;
#11051=CARTESIAN_POINT ( 'NONE',  ( -4.984841277089891776, 213.7757310962905990, 32.94886208192144039 ) ) ;
#11059=CARTESIAN_POINT ( 'NONE',  ( 2.426778023690261410, 199.3768101843759837, 50.60113791807857808 ) ) ;
#11062=CARTESIAN_POINT ( 'NONE',  ( 10.00000000000000711, 207.0476921513415220, 30.99886208192143755 ) ) ;
#11067=CARTESIAN_POINT ( 'NONE',  ( -4.903702542908436435, 200.1653181626580249, 14.04886208192143471 ) ) ;
#11069=CARTESIAN_POINT ( 'NONE',  ( -6.139770520408369237, 215.5359834540460042, 48.95113791807855108 ) ) ;
#11071=CARTESIAN_POINT ( 'NONE',  ( 3.135527875058820690, 216.4958274776887492, 34.40113791807856813 ) ) ;
#11075=CARTESIAN_POINT ( 'NONE',  ( 6.444103211790928043, 211.7408657792734061, 87.69886208192144750 ) ) ;
#11079=CARTESIAN_POINT ( 'NONE',  ( 11.98450388067348271, 203.0532714938637753, 23.15113791807856458 ) ) ;
#11082=CARTESIAN_POINT ( 'NONE',  ( -8.118202686958039038, 201.1607312380087080, 69.20113791807858661 ) ) ;
#11083=CARTESIAN_POINT ( 'NONE',  ( 8.062137200540920645, 201.0835637161417822, 38.30113791807857382 ) ) ;
#11087=CARTESIAN_POINT ( 'NONE',  ( 6.220909254589680693, 198.5229672870052582, 10.44886208192143506 ) ) ;
#11090=CARTESIAN_POINT ( 'NONE',  ( 12.00000000000000711, 206.9523078486586485, 44.00113791807856956 ) ) ;
#11092=CARTESIAN_POINT ( 'NONE',  ( 3.044812012439969795, 216.5253028482143520, 18.39886208192143613 ) ) ;
#11095=CARTESIAN_POINT ( 'NONE',  ( 3.044812012440130555, 197.4746971517856764, 77.60113791807857808 ) ) ;
#11102=CARTESIAN_POINT ( 'NONE',  ( -7.984503880673488041, 209.6470497212046098, 18.65113791807856458 ) ) ;
#11105=CARTESIAN_POINT ( 'NONE',  ( -10.00000000000000711, 206.9523078486584495, 8.498862081921433997 ) ) ;
#11113=CARTESIAN_POINT ( 'NONE',  ( -3.135527875058982783, 216.4958274776886924, 78.09886208192143897 ) ) ;
#11115=CARTESIAN_POINT ( 'NONE',  ( 10.00000000000000711, 206.9523078486586201, 26.00113791807856956 ) ) ;
#11117=CARTESIAN_POINT ( 'NONE',  ( -3.753561863808878130, 218.3979405102790281, 84.09886208192143897 ) ) ;
#11122=CARTESIAN_POINT ( 'NONE',  ( -8.118202686958039038, 201.1607312380087080, 93.20113791807857240 ) ) ;
#11126=CARTESIAN_POINT ( 'NONE',  ( -3.044812012440131443, 216.5253028482142952, 34.10113791807857808 ) ) ;
#11129=DIRECTION ( 'NONE',  ( -0.2649168722799616349, 0.9642688156137669830, -0.002168413296787739895 ) ) ;
#11131=CARTESIAN_POINT ( 'NONE',  ( -0.05014649552807705357, 194.3824533091408000, 8.751137918078567779 ) ) ;
#11135=( GEOMETRIC_REPRESENTATION_CONTEXT ( 3 ) GLOBAL_UNCERTAINTY_ASSIGNED_CONTEXT ( ( #13436 ) ) GLOBAL_UNIT_ASSIGNED_CONTEXT ( ( #19726, #6452, #3721 ) ) REPRESENTATION_CONTEXT ( 'NONE', 'WORKASPACE' ) );
#11136=CARTESIAN_POINT ( 'NONE',  ( -9.984503880673420539, 203.7031108863293980, 92.34886208192142476 ) ) ;
#11137=CARTESIAN_POINT ( 'NONE',  ( 9.736236675708031640, 199.9851607334238963, 28.29886208192143826 ) ) ;
#11139=CARTESIAN_POINT ( 'NONE',  ( 10.00000000000000711, 206.9523078486586201, 53.00113791807857666 ) ) ;
#11141=CARTESIAN_POINT ( 'NONE',  ( 8.000000000000008882, 207.0476921513415220, 9.998862081921435774 ) ) ;
#11144=CARTESIAN_POINT ( 'NONE',  ( -8.000000000000008882, 206.9523078486584780, 86.49886208192144466 ) ) ;
#11145=CARTESIAN_POINT ( 'NONE',  ( 4.984841277089725686, 213.7757310962907411, 34.55113791807856671 ) ) ;
#11151=CARTESIAN_POINT ( 'NONE',  ( 0.05014649552807626948, 215.4116977939061144, 100.2511379180785696 ) ) ;
#11155=CARTESIAN_POINT ( 'NONE',  ( -6.444103211790928043, 202.2591342207265939, 77.19886208192143329 ) ) ;
#11158=CARTESIAN_POINT ( 'NONE',  ( -10.00000000000000711, 207.0476921513413515, 9.501137918078566003 ) ) ;
#11162=CARTESIAN_POINT ( 'NONE',  ( -7.375838497908182134, 217.2372850707499765, 78.95113791807858661 ) ) ;
#11163=CARTESIAN_POINT ( 'NONE',  ( 10.00000000000000711, 206.9523078486586201, 101.0011379180785696 ) ) ;
#11166=CARTESIAN_POINT ( 'NONE',  ( -3.044812012439970683, 197.4746971517856196, 1.898862081921434353 ) ) ;
#11167=CARTESIAN_POINT ( 'NONE',  ( 0.05014649552828288198, 194.3824533091408000, 64.74886208192143044 ) ) ;
#11168=CARTESIAN_POINT ( 'NONE',  ( 8.062137200540822946, 212.9164362838583315, 69.69886208192144750 ) ) ;
#11169=CARTESIAN_POINT ( 'NONE',  ( -9.736236675708031640, 214.0148392665760753, 8.798862081921434708 ) ) ;
#11171=CARTESIAN_POINT ( 'NONE',  ( -3.044812012440131443, 216.5253028482142952, 25.10113791807856742 ) ) ;
#11172=CARTESIAN_POINT ( 'NONE',  ( 9.984503880673420539, 210.2968891136705167, 84.84886208192143897 ) ) ;
#11176=CARTESIAN_POINT ( 'NONE',  ( -8.015496119326597224, 209.5516654185217362, 62.64886208192143613 ) ) ;
#11179=VERTEX_POINT ( 'NONE', #2108 ) ;
#11182=CARTESIAN_POINT ( 'NONE',  ( 8.015496119326531499, 209.5516654185219636, 64.85113791807857808 ) ) ;
#11186=CARTESIAN_POINT ( 'NONE',  ( -2.517493886309087880, 214.5937144450984135, 45.09886208192144608 ) ) ;
#11187=CARTESIAN_POINT ( 'NONE',  ( 6.139770520408368348, 198.4640165459539674, 77.45113791807854398 ) ) ;
#11188=CARTESIAN_POINT ( 'NONE',  ( -6.139770520408369237, 215.5359834540460042, 63.95113791807857950 ) ) ;
#11191=CARTESIAN_POINT ( 'NONE',  ( -0.05014649552807731031, 198.5883022060938572, 23.75113791807855890 ) ) ;
#11195=CARTESIAN_POINT ( 'NONE',  ( -9.680171189290831535, 214.0920067884431148, 51.80113791807857382 ) ) ;
#11196=DIRECTION ( 'NONE',  ( 0.000000000000000000, -0.04769215134144196705, 0.9988620819214357738 ) ) ;
#11197=CARTESIAN_POINT ( 'NONE',  ( -9.984503880673473830, 210.2968891136704315, 96.65113791807857524 ) ) ;
#11198=CARTESIAN_POINT ( 'NONE',  ( -6.220909254589537696, 198.5229672870051445, 69.05113791807856671 ) ) ;
#11199=CARTESIAN_POINT ( 'NONE',  ( -3.753561863808878130, 218.3979405102790281, 30.09886208192144252 ) ) ;
#11200=CARTESIAN_POINT ( 'NONE',  ( -0.05014649552828402690, 217.5146222423826714, 39.24886208192143044 ) ) ;
#11202=CARTESIAN_POINT ( 'NONE',  ( 9.736236675707914401, 214.0148392665762458, 73.70113791807857240 ) ) ;
#11203=CARTESIAN_POINT ( 'NONE',  ( -2.517493886308901807, 199.4062855549015012, 101.9011379180785895 ) ) ;
#11205=CARTESIAN_POINT ( 'NONE',  ( 9.984503880673420539, 210.2968891136705167, 48.84886208192143187 ) ) ;
#11208=CARTESIAN_POINT ( 'NONE',  ( 12.01549611932659367, 203.1486557965466773, 64.14886208192143613 ) ) ;
#11209=EDGE_LOOP ( 'NONE', ( #2289, #25889, #17489, #22174 ) ) ;
#11210=CARTESIAN_POINT ( 'NONE',  ( 7.984503880673422316, 209.6470497212048372, 33.84886208192144608 ) ) ;
#11217=CARTESIAN_POINT ( 'NONE',  ( 6.444103211791042618, 202.2591342207267644, 56.30113791807857382 ) ) ;
#11218=CARTESIAN_POINT ( 'NONE',  ( 6.139770520408223575, 215.5359834540460611, 36.54886208192142050 ) ) ;
#11223=CARTESIAN_POINT ( 'NONE',  ( -0.05014649552828365914, 215.4116977939061144, 12.24886208192143577 ) ) ;
#11224=CARTESIAN_POINT ( 'NONE',  ( -10.01549611932653860, 203.7984951890123284, 48.35113791807855677 ) ) ;
#11226=CARTESIAN_POINT ( 'NONE',  ( -8.118202686958039038, 201.1607312380087080, 33.20113791807857240 ) ) ;
#11228=CARTESIAN_POINT ( 'NONE',  ( -8.015496119326597224, 209.5516654185217362, 98.64886208192146455 ) ) ;
#11232=CARTESIAN_POINT ( 'NONE',  ( 12.01549611932652972, 210.8513442034534933, 16.85113791807856742 ) ) ;
#11236=CARTESIAN_POINT ( 'NONE',  ( -9.984503880673473830, 210.2968891136704315, 63.65113791807857524 ) ) ;
#11238=CARTESIAN_POINT ( 'NONE',  ( -8.062137200540920645, 212.9164362838581894, 39.80113791807857382 ) ) ;
#11243=CARTESIAN_POINT ( 'NONE',  ( -9.736236675707914401, 199.9851607334237542, 102.2011379180785866 ) ) ;
#11244=CARTESIAN_POINT ( 'NONE',  ( -9.984503880673420539, 203.7031108863293980, 11.34886208192143364 ) ) ;
#11247=CARTESIAN_POINT ( 'NONE',  ( 0.05014649552807549926, 219.6175466908591716, 46.25113791807856956 ) ) ;
#11250=CYLINDRICAL_SURFACE ( 'NONE', #5560, 1.000000000000000222 ) ;
#11251=CARTESIAN_POINT ( 'NONE',  ( -3.044812012439970683, 197.4746971517856196, 19.89886208192143613 ) ) ;
#11255=CARTESIAN_POINT ( 'NONE',  ( 10.00000000000000711, 206.9523078486586201, 77.00113791807858377 ) ) ;
#11261=CARTESIAN_POINT ( 'NONE',  ( -6.444103211791042618, 211.7408657792732356, 24.80113791807857027 ) ) ;
#11265=CARTESIAN_POINT ( 'NONE',  ( -8.118202686958138514, 212.8392687619910930, 2.798862081921434708 ) ) ;
#11273=CARTESIAN_POINT ( 'NONE',  ( -8.118202686958138514, 212.8392687619910930, 86.79886208192142760 ) ) ;
#11275=CARTESIAN_POINT ( 'NONE',  ( 3.044812012440130555, 197.4746971517856764, 26.60113791807856742 ) ) ;
#11277=CARTESIAN_POINT ( 'NONE',  ( 12.01549611932659367, 203.1486557965466773, 79.14886208192143613 ) ) ;
#11281=CARTESIAN_POINT ( 'NONE',  ( -3.135527875058821579, 197.5041725223112223, 92.90113791807857524 ) ) ;
#11284=CARTESIAN_POINT ( 'NONE',  ( 10.00000000000000711, 206.9523078486586201, 35.00113791807856956 ) ) ;
#11289=CARTESIAN_POINT ( 'NONE',  ( -12.00000000000000711, 207.0476921513413515, 18.50113791807856956 ) ) ;
#11295=TOROIDAL_SURFACE ( 'NONE', #10690, 4.999999999999993783, 1.000000000000000222 ) ;
#11296=CARTESIAN_POINT ( 'NONE',  ( -12.00000000000000711, 206.9523078486584780, 32.49886208192143044 ) ) ;
#11298=CARTESIAN_POINT ( 'NONE',  ( 10.01549611932653860, 210.2015048109876716, 49.85113791807857808 ) ) ;
#11301=CARTESIAN_POINT ( 'NONE',  ( 0.05014649552828262524, 198.5883022060938572, 10.74886208192143577 ) ) ;
#11305=CARTESIAN_POINT ( 'NONE',  ( -2.426778023690076225, 199.3768101843759553, 103.8988620819214361 ) ) ;
#11306=CARTESIAN_POINT ( 'NONE',  ( 7.984503880673485376, 204.3529502787953902, 41.15113791807857524 ) ) ;
#11310=AXIS2_PLACEMENT_3D ( 'NONE', #24923, #17088, #8746 ) ;
#11311=CARTESIAN_POINT ( 'NONE',  ( 3.135527875058981895, 197.5041725223112792, 58.59886208192143897 ) ) ;
#11314=CARTESIAN_POINT ( 'NONE',  ( 0.05014649552807626948, 215.4116977939061144, 94.25113791807859798 ) ) ;
#11317=CARTESIAN_POINT ( 'NONE',  ( -8.000000000000008882, 206.9523078486584780, 68.49886208192144466 ) ) ;
#11319=CIRCLE ( 'NONE', #11880, 8.624472924841564136 ) ;
#11321=CARTESIAN_POINT ( 'NONE',  ( 3.135527875058820690, 216.4958274776887492, 7.401137918078566358 ) ) ;
#11326=CARTESIAN_POINT ( 'NONE',  ( -12.01549611932652972, 203.1486557965464499, 78.35113791807857808 ) ) ;
#11327=CARTESIAN_POINT ( 'NONE',  ( -8.062137200540920645, 212.9164362838581894, 93.80113791807858092 ) ) ;
#11330=CARTESIAN_POINT ( 'NONE',  ( -9.984503880673420539, 203.7031108863293980, 2.348862081921433198 ) ) ;
#11331=CARTESIAN_POINT ( 'NONE',  ( 7.456977232089471386, 196.8216656703012006, 64.44886208192143329 ) ) ;
#11332=CARTESIAN_POINT ( 'NONE',  ( -6.220909254589682469, 215.4770327129947134, 62.94886208192143329 ) ) ;
#11333=CARTESIAN_POINT ( 'NONE',  ( 7.375838497908012492, 217.2372850707501186, 6.548862081921433820 ) ) ;
#11336=CARTESIAN_POINT ( 'NONE',  ( -8.118202686958039038, 201.1607312380087080, 24.20113791807856884 ) ) ;
#11337=CARTESIAN_POINT ( 'NONE',  ( -10.00000000000000711, 206.9523078486584495, 86.49886208192144466 ) ) ;
#11344=CARTESIAN_POINT ( 'NONE',  ( 8.000000000000008882, 207.0476921513415220, 72.99886208192144466 ) ) ;
#11351=CARTESIAN_POINT ( 'NONE',  ( 6.500168698208129925, 211.6636982574063381, 70.70113791807857240 ) ) ;
#11355=CARTESIAN_POINT ( 'NONE',  ( -6.500168698208244500, 211.6636982574061676, 44.79886208192144181 ) ) ;
#11357=CARTESIAN_POINT ( 'NONE',  ( 6.220909254589536808, 215.4770327129947702, 82.55113791807858092 ) ) ;
#11358=CARTESIAN_POINT ( 'NONE',  ( 6.220909254589536808, 215.4770327129947702, 67.55113791807853829 ) ) ;
#11360=CARTESIAN_POINT ( 'NONE',  ( -7.375838497908014268, 196.7627149292498530, 23.04886208192143826 ) ) ;
#11362=CARTESIAN_POINT ( 'NONE',  ( -6.444103211791042618, 211.7408657792732356, 24.80113791807857027 ) ) ;
#11367=CARTESIAN_POINT ( 'NONE',  ( 9.680171189290831535, 199.9079932115568852, 47.30113791807856671 ) ) ;
#11369=CARTESIAN_POINT ( 'NONE',  ( -10.00000000000000711, 207.0476921513413515, 96.50113791807856956 ) ) ;
#11370=CARTESIAN_POINT ( 'NONE',  ( 9.984503880673473830, 203.7031108863295401, 68.15113791807857524 ) ) ;
#11372=CARTESIAN_POINT ( 'NONE',  ( 9.736236675708031640, 199.9851607334238963, 34.29886208192143471 ) ) ;
#11373=CARTESIAN_POINT ( 'NONE',  ( 9.984503880673420539, 210.2968891136705736, 39.84886208192142476 ) ) ;
#11375=CARTESIAN_POINT ( 'NONE',  ( -3.753561863808691168, 195.6020594897209435, 74.90113791807856103 ) ) ;
#11376=CARTESIAN_POINT ( 'NONE',  ( 4.903702542908601636, 200.1653181626581102, 98.45113791807858661 ) ) ;
#11377=CARTESIAN_POINT ( 'NONE',  ( -9.984503880673420539, 203.7031108863293980, 59.34886208192141765 ) ) ;
#11380=CARTESIAN_POINT ( 'NONE',  ( -9.736236675708031640, 214.0148392665760753, 59.79886208192143471 ) ) ;
#11383=CARTESIAN_POINT ( 'NONE',  ( -8.000000000000008882, 206.9523078486584780, 29.49886208192143400 ) ) ;
#11391=CARTESIAN_POINT ( 'NONE',  ( -8.000000000000008882, 207.0476921513413515, 51.50113791807856956 ) ) ;
#11393=CARTESIAN_POINT ( 'NONE',  ( 8.118202686958138514, 201.1607312380088501, 37.29886208192143471 ) ) ;
#11399=CARTESIAN_POINT ( 'NONE',  ( -4.984841277089891776, 213.7757310962905990, 11.94886208192143506 ) ) ;
#11400=CARTESIAN_POINT ( 'NONE',  ( 3.044812012440130555, 197.4746971517856764, 47.60113791807857098 ) ) ;
#11402=CARTESIAN_POINT ( 'NONE',  ( -6.139770520408369237, 215.5359834540460042, 36.95113791807857240 ) ) ;
#11404=CARTESIAN_POINT ( 'NONE',  ( -2.426778023690076225, 199.3768101843759553, 103.8988620819214361 ) ) ;
#11408=CARTESIAN_POINT ( 'NONE',  ( 3.753561863808689836, 218.3979405102790565, 22.40113791807856813 ) ) ;
#11409=AXIS2_PLACEMENT_3D ( 'NONE', #23527, #5954, #29134 ) ;
#11412=CARTESIAN_POINT ( 'NONE',  ( -9.984503880673473830, 210.2968891136704315, 66.65113791807857524 ) ) ;
#11413=CARTESIAN_POINT ( 'NONE',  ( -10.00000000000000711, 207.0476921513413515, 42.50113791807856956 ) ) ;
#11414=CARTESIAN_POINT ( 'NONE',  ( 8.640141755188686545, 206.6086104956403915, 111.6972426105882477 ) ) ;
#11416=CARTESIAN_POINT ( 'NONE',  ( 3.662846001189864698, 218.4274158808046593, 6.398862081921435241 ) ) ;
#11417=CARTESIAN_POINT ( 'NONE',  ( 10.01549611932659367, 203.7984951890124421, 13.14886208192143435 ) ) ;
#11420=CARTESIAN_POINT ( 'NONE',  ( 3.753561863808689836, 218.3979405102790565, 46.40113791807856813 ) ) ;
#11421=CARTESIAN_POINT ( 'NONE',  ( 2.426778023690261410, 199.3768101843759837, 68.60113791807857808 ) ) ;
#11422=CARTESIAN_POINT ( 'NONE',  ( -0.05014649552828403384, 217.5146222423826714, 30.24886208192142689 ) ) ;
#11426=CARTESIAN_POINT ( 'NONE',  ( -8.118202686958039038, 201.1607312380087080, 81.20113791807857240 ) ) ;
#11431=CARTESIAN_POINT ( 'NONE',  ( 7.984503880673485376, 204.3529502787953902, 23.15113791807856458 ) ) ;
#11434=CARTESIAN_POINT ( 'NONE',  ( -6.220909254589682469, 215.4770327129946850, 5.948862081921435063 ) ) ;
#11441=CARTESIAN_POINT ( 'NONE',  ( 6.139770520408223575, 215.5359834540460611, 93.54886208192139918 ) ) ;
#11443=CARTESIAN_POINT ( 'NONE',  ( 6.220909254589536808, 215.4770327129947702, 19.55113791807856671 ) ) ;
#11445=CARTESIAN_POINT ( 'NONE',  ( -3.662846001189865142, 195.5725841191952838, 79.89886208192143613 ) ) ;
#11449=CARTESIAN_POINT ( 'NONE',  ( -3.044812012440131443, 216.5253028482142952, 91.10113791807857808 ) ) ;
#11452=CARTESIAN_POINT ( 'NONE',  ( 9.984503880673470277, 203.7031108863295401, 41.15113791807855392 ) ) ;
#11457=CARTESIAN_POINT ( 'NONE',  ( 12.00000000000000711, 206.9523078486586485, 17.00113791807856956 ) ) ;
#11462=CARTESIAN_POINT ( 'NONE',  ( -9.736236675708031640, 214.0148392665760753, 32.79886208192143471 ) ) ;
#11463=CARTESIAN_POINT ( 'NONE',  ( 10.00000000000000711, 206.9523078486586201, -0.9988620819214343305 ) ) ;
#11464=CARTESIAN_POINT ( 'NONE',  ( -9.984503880673473830, 210.2968891136704315, 54.65113791807858235 ) ) ;
#11466=CARTESIAN_POINT ( 'NONE',  ( 8.000000000000008882, 207.0476921513415220, 15.99886208192143577 ) ) ;
#11472=CARTESIAN_POINT ( 'NONE',  ( 7.984503880673422316, 209.6470497212048372, 96.84886208192143897 ) ) ;
#11475=CARTESIAN_POINT ( 'NONE',  ( -2.426778023690262742, 214.6231898156240163, 37.10113791807857098 ) ) ;
#11479=CARTESIAN_POINT ( 'NONE',  ( -10.01549611932659722, 210.2015048109875011, 59.64886208192143613 ) ) ;
#11482=CARTESIAN_POINT ( 'NONE',  ( -8.000000000000008882, 207.0476921513413515, 93.50113791807858377 ) ) ;
#11486=CARTESIAN_POINT ( 'NONE',  ( -8.015496119326597224, 209.5516654185217362, 68.64886208192142192 ) ) ;
#11490=CARTESIAN_POINT ( 'NONE',  ( -8.062137200540920645, 212.9164362838581894, 6.801137918078565825 ) ) ;
#11496=CARTESIAN_POINT ( 'NONE',  ( -9.680171189290831535, 214.0920067884431148, 72.80113791807858092 ) ) ;
#11497=CARTESIAN_POINT ( 'NONE',  ( -9.984503880673475606, 210.2968891136704315, 96.65113791807858945 ) ) ;
#11500=CARTESIAN_POINT ( 'NONE',  ( 3.044812012439969795, 216.5253028482143520, 3.398862081921434797 ) ) ;
#11501=CARTESIAN_POINT ( 'NONE',  ( -9.680171189290716072, 199.9079932115567146, 62.19886208192144039 ) ) ;
#11502=CARTESIAN_POINT ( 'NONE',  ( -3.135527875058982783, 216.4958274776886924, 69.09886208192143897 ) ) ;
#11503=CARTESIAN_POINT ( 'NONE',  ( 9.680171189290716072, 214.0920067884432854, 3.698862081921433731 ) ) ;
#11505=CARTESIAN_POINT ( 'NONE',  ( -8.062137200540920645, 212.9164362838581894, 18.80113791807856671 ) ) ;
#11506=CARTESIAN_POINT ( 'NONE',  ( 6.220909254589681581, 198.5229672870052582, 88.44886208192144750 ) ) ;
#11509=ORIENTED_EDGE ( 'NONE', *, *, #20368, .T. ) ;
#11511=CARTESIAN_POINT ( 'NONE',  ( 6.500168698208244500, 202.3363017425938324, 67.29886208192144181 ) ) ;
#11518=CARTESIAN_POINT ( 'NONE',  ( -6.444103211791042618, 211.7408657792732356, 69.80113791807856671 ) ) ;
#11522=CARTESIAN_POINT ( 'NONE',  ( 4.903702542908435547, 213.8346818373419751, 42.54886208192144181 ) ) ;
#11523=CARTESIAN_POINT ( 'NONE',  ( -3.135527875058821579, 197.5041725223112223, 92.90113791807857524 ) ) ;
#11524=CARTESIAN_POINT ( 'NONE',  ( -8.062137200540920645, 212.9164362838581894, 69.80113791807856671 ) ) ;
#11530=CARTESIAN_POINT ( 'NONE',  ( 0.05014649552807549926, 219.6175466908591716, 49.25113791807856956 ) ) ;
#11532=CARTESIAN_POINT ( 'NONE',  ( 10.00000000000000711, 206.9523078486586201, 95.00113791807856956 ) ) ;
#11533=CARTESIAN_POINT ( 'NONE',  ( -10.01549611932653860, 203.7984951890123000, 69.35113791807857808 ) ) ;
#11534=CARTESIAN_POINT ( 'NONE',  ( -7.375838497908014268, 196.7627149292498530, 32.04886208192143471 ) ) ;
#11535=CARTESIAN_POINT ( 'NONE',  ( -3.044812012439970683, 197.4746971517856196, 40.89886208192143613 ) ) ;
#11537=CARTESIAN_POINT ( 'NONE',  ( 7.456977232089302632, 217.1783343296989131, 76.55113791807858092 ) ) ;
#11538=CARTESIAN_POINT ( 'NONE',  ( 4.984841277089725686, 213.7757310962907411, 94.55113791807855250 ) ) ;
#11539=CARTESIAN_POINT ( 'NONE',  ( 6.220909254589681581, 198.5229672870052582, 55.44886208192141908 ) ) ;
#11542=CARTESIAN_POINT ( 'NONE',  ( 9.680171189290716072, 214.0920067884432854, 57.69886208192144039 ) ) ;
#11545=CARTESIAN_POINT ( 'NONE',  ( -8.015496119326597224, 209.5516654185217362, 41.64886208192143613 ) ) ;
#11550=CARTESIAN_POINT ( 'NONE',  ( 4.984841277089725686, 213.7757310962907411, 49.55113791807858092 ) ) ;
#11552=CARTESIAN_POINT ( 'NONE',  ( -3.044812012439970683, 197.4746971517856196, 31.89886208192143613 ) ) ;
#11557=FILL_AREA_STYLE_COLOUR ( '', #2964 ) ;
#11560=CARTESIAN_POINT ( 'NONE',  ( 2.426778023690075337, 214.6231898156240447, 12.39886208192143613 ) ) ;
#11561=CARTESIAN_POINT ( 'NONE',  ( 6.139770520408368348, 198.4640165459539674, 59.45113791807855819 ) ) ;
#11563=CARTESIAN_POINT ( 'NONE',  ( -6.139770520408369237, 215.5359834540460042, 39.95113791807857240 ) ) ;
#11565=CARTESIAN_POINT ( 'NONE',  ( 6.444103211790928043, 211.7408657792734061, 99.69886208192144750 ) ) ;
#11570=CARTESIAN_POINT ( 'NONE',  ( -0.05014649552807705357, 194.3824533091408000, 23.75113791807855890 ) ) ;
#11572=CARTESIAN_POINT ( 'NONE',  ( 8.118202686958039038, 212.8392687619912635, 61.70113791807857240 ) ) ;
#11573=CARTESIAN_POINT ( 'NONE',  ( 8.062137200540920645, 201.0835637161417822, 44.30113791807857382 ) ) ;
#11576=CARTESIAN_POINT ( 'NONE',  ( 0.05014649552828288198, 194.3824533091408000, 7.748862081921433109 ) ) ;
#11577=CARTESIAN_POINT ( 'NONE',  ( -10.00000000000000711, 206.9523078486584495, 5.498862081921434886 ) ) ;
#11580=CARTESIAN_POINT ( 'NONE',  ( -7.375838497908182134, 217.2372850707499765, 51.95113791807855819 ) ) ;
#11581=CARTESIAN_POINT ( 'NONE',  ( -6.444103211791042618, 211.7408657792732356, 66.80113791807858092 ) ) ;
#11583=CARTESIAN_POINT ( 'NONE',  ( -8.062137200540822946, 201.0835637161416400, 29.19886208192143684 ) ) ;
#11587=CARTESIAN_POINT ( 'NONE',  ( -6.139770520408369237, 215.5359834540460042, 81.95113791807854398 ) ) ;
#11592=CARTESIAN_POINT ( 'NONE',  ( -4.903702542908602524, 213.8346818373418898, 18.95113791807856529 ) ) ;
#11596=CARTESIAN_POINT ( 'NONE',  ( -12.05084501415679199, 219.7456114157811271, 104.9910338291041114 ) ) ;
#11601=CARTESIAN_POINT ( 'NONE',  ( -0.05014649552807731031, 198.5883022060938572, 47.75113791807856245 ) ) ;
#11604=CARTESIAN_POINT ( 'NONE',  ( 6.220909254589681581, 198.5229672870052582, 91.44886208192143329 ) ) ;
#11606=CARTESIAN_POINT ( 'NONE',  ( -10.00000000000000711, 207.0476921513413515, 33.50113791807856956 ) ) ;
#11609=CARTESIAN_POINT ( 'NONE',  ( 9.680171189290716072, 214.0920067884432854, 81.69886208192144750 ) ) ;
#11615=CARTESIAN_POINT ( 'NONE',  ( 8.118202686958039038, 212.8392687619912635, 97.70113791807857240 ) ) ;
#11618=CARTESIAN_POINT ( 'NONE',  ( -6.220909254589537696, 198.5229672870051161, 42.05113791807857382 ) ) ;
#11625=AXIS2_PLACEMENT_3D ( 'NONE', #7172, #2062, #2229 ) ;
#11627=CARTESIAN_POINT ( 'NONE',  ( 7.375838497908181246, 196.7627149292499666, 20.45113791807856529 ) ) ;
#11634=CARTESIAN_POINT ( 'NONE',  ( -11.98450388067341876, 203.0532714938636047, 47.34886208192143897 ) ) ;
#11635=CARTESIAN_POINT ( 'NONE',  ( -10.00000000000000711, 207.0476921513413515, 0.5011379180785656695 ) ) ;
#11636=CARTESIAN_POINT ( 'NONE',  ( -10.01549611932653860, 203.7984951890123284, 54.35113791807856387 ) ) ;
#11638=CARTESIAN_POINT ( 'NONE',  ( -4.984841277089891776, 213.7757310962905990, 11.94886208192143506 ) ) ;
#11641=CARTESIAN_POINT ( 'NONE',  ( -2.517493886309087880, 214.5937144450984135, 99.09886208192145318 ) ) ;
#11644=CARTESIAN_POINT ( 'NONE',  ( -0.05014649552807731031, 198.5883022060938572, 44.75113791807857666 ) ) ;
#11645=DIRECTION ( 'NONE',  ( -0.2649168722799636333, 0.9642688156137663169, -0.002168413296789690158 ) ) ;
#11649=CARTESIAN_POINT ( 'NONE',  ( -10.01549611932659722, 210.2015048109875011, 62.64886208192143613 ) ) ;
#11653=CARTESIAN_POINT ( 'NONE',  ( 6.444103211791042618, 202.2591342207267644, 95.30113791807858092 ) ) ;
#11656=CARTESIAN_POINT ( 'NONE',  ( -6.444103211790928043, 202.2591342207265939, 80.19886208192143329 ) ) ;
#11660=CARTESIAN_POINT ( 'NONE',  ( -10.00000000000000711, 207.0476921513413515, 21.50113791807856956 ) ) ;
#11664=CARTESIAN_POINT ( 'NONE',  ( -3.753561863808691168, 195.6020594897209435, 83.90113791807856103 ) ) ;
#11670=CARTESIAN_POINT ( 'NONE',  ( 9.736236675708031640, 199.9851607334238963, 64.29886208192144181 ) ) ;
#11671=CARTESIAN_POINT ( 'NONE',  ( 10.00000000000000711, 207.0476921513415220, 75.99886208192144466 ) ) ;
#11672=CARTESIAN_POINT ( 'NONE',  ( 9.680171189290716072, 214.0920067884432854, 12.69886208192143684 ) ) ;
#11674=CARTESIAN_POINT ( 'NONE',  ( -8.062137200540920645, 212.9164362838581894, 21.80113791807856671 ) ) ;
#11676=CARTESIAN_POINT ( 'NONE',  ( 6.220909254589681581, 198.5229672870052582, 91.44886208192143329 ) ) ;
#11681=CARTESIAN_POINT ( 'NONE',  ( -2.517493886309087880, 214.5937144450984135, 75.09886208192142476 ) ) ;
#11682=ADVANCED_FACE ( 'NONE', ( #19611 ), #9549, .F. ) ;
#11690=CARTESIAN_POINT ( 'NONE',  ( 4.903702542908601636, 200.1653181626581102, 65.45113791807858661 ) ) ;
#11694=CARTESIAN_POINT ( 'NONE',  ( -4.984841277089891776, 213.7757310962905990, 41.94886208192144750 ) ) ;
#11695=CARTESIAN_POINT ( 'NONE',  ( -3.044812012440131443, 216.5253028482142952, 76.10113791807856387 ) ) ;
#11700=CARTESIAN_POINT ( 'NONE',  ( 0.05014649552807549926, 219.6175466908591716, 58.25113791807856245 ) ) ;
#11702=CARTESIAN_POINT ( 'NONE',  ( -7.456977232089304408, 196.8216656703010301, 3.051137918078566269 ) ) ;
#11703=CARTESIAN_POINT ( 'NONE',  ( 3.135527875058820690, 216.4958274776887492, 64.40113791807857524 ) ) ;
#11704=CARTESIAN_POINT ( 'NONE',  ( -3.753561863808878130, 218.3979405102790281, 33.09886208192143187 ) ) ;
#11705=CARTESIAN_POINT ( 'NONE',  ( 10.00000000000000711, 207.0476921513415220, 51.99886208192143755 ) ) ;
#11707=CARTESIAN_POINT ( 'NONE',  ( -9.736236675707914401, 199.9851607334237542, 75.20113791807857240 ) ) ;
#11708=CARTESIAN_POINT ( 'NONE',  ( -8.000000000000008882, 207.0476921513413515, 96.50113791807856956 ) ) ;
#11709=CARTESIAN_POINT ( 'NONE',  ( 8.062137200540822946, 212.9164362838583315, 57.69886208192144039 ) ) ;
#11712=CARTESIAN_POINT ( 'NONE',  ( 11.98450388067341876, 210.9467285061363953, 63.84886208192143187 ) ) ;
#11715=CARTESIAN_POINT ( 'NONE',  ( -6.500168698208244500, 211.6636982574061676, 38.79886208192143471 ) ) ;
#11720=CARTESIAN_POINT ( 'NONE',  ( 4.984841277089725686, 213.7757310962907411, 52.55113791807858092 ) ) ;
#11722=CARTESIAN_POINT ( 'NONE',  ( -10.00000000000000711, 206.9523078486584495, 32.49886208192143044 ) ) ;
#11728=CARTESIAN_POINT ( 'NONE',  ( 6.500168698208244500, 202.3363017425938324, 13.29886208192143826 ) ) ;
#11729=CARTESIAN_POINT ( 'NONE',  ( -8.062137200540920645, 212.9164362838581894, 57.80113791807857382 ) ) ;
#11730=CARTESIAN_POINT ( 'NONE',  ( -10.00000000000000711, 207.0476921513413515, 48.50113791807856956 ) ) ;
#11732=CARTESIAN_POINT ( 'NONE',  ( 2.517493886309087436, 199.4062855549015865, 100.5988620819214532 ) ) ;
#11736=CARTESIAN_POINT ( 'NONE',  ( 9.736236675707914401, 214.0148392665762458, 22.70113791807856529 ) ) ;
#11738=CARTESIAN_POINT ( 'NONE',  ( -8.118202686958039038, 201.1607312380087080, 66.20113791807857240 ) ) ;
#11739=CARTESIAN_POINT ( 'NONE',  ( 9.984503880673473830, 203.7031108863295401, 35.15113791807856103 ) ) ;
#11742=CARTESIAN_POINT ( 'NONE',  ( -12.00000000000000711, 206.9523078486584780, 2.498862081921434442 ) ) ;
#11743=CARTESIAN_POINT ( 'NONE',  ( 6.220909254589680693, 198.5229672870052582, 19.44886208192143329 ) ) ;
#11746=CARTESIAN_POINT ( 'NONE',  ( -12.00000000000000711, 207.0476921513413515, 51.50113791807856956 ) ) ;
#11747=CARTESIAN_POINT ( 'NONE',  ( 0.05014649552807626948, 215.4116977939061144, 73.25113791807858377 ) ) ;
#11748=CARTESIAN_POINT ( 'NONE',  ( -8.118202686958138514, 212.8392687619910930, 29.79886208192143826 ) ) ;
#11752=CARTESIAN_POINT ( 'NONE',  ( -6.220909254589537696, 198.5229672870051161, 90.05113791807858092 ) ) ;
#11758=CARTESIAN_POINT ( 'NONE',  ( -8.015496119326531499, 204.4483345814780364, 27.35113791807856742 ) ) ;
#11760=CARTESIAN_POINT ( 'NONE',  ( 6.139770520408223575, 215.5359834540460611, 3.548862081921434708 ) ) ;
#11763=CARTESIAN_POINT ( 'NONE',  ( 2.426778023690261410, 199.3768101843759837, 50.60113791807857808 ) ) ;
#11766=CARTESIAN_POINT ( 'NONE',  ( -9.984503880673420539, 203.7031108863293980, 95.34886208192142476 ) ) ;
#11768=CARTESIAN_POINT ( 'NONE',  ( 10.01549611932653860, 210.2015048109876716, 34.85113791807856387 ) ) ;
#11770=CARTESIAN_POINT ( 'NONE',  ( -9.736236675708031640, 214.0148392665760753, 83.79886208192144181 ) ) ;
#11775=DIRECTION ( 'NONE',  ( 0.000000000000000000, 0.9963496021943381020, -0.08536668089591059605 ) ) ;
#11776=CARTESIAN_POINT ( 'NONE',  ( -10.00000000000000711, 207.0476921513413515, 93.50113791807858377 ) ) ;
#11779=CARTESIAN_POINT ( 'NONE',  ( -3.135527875058821579, 197.5041725223112223, 35.90113791807856813 ) ) ;
#11787=CARTESIAN_POINT ( 'NONE',  ( 7.456977232089302632, 217.1783343296989131, 16.55113791807857027 ) ) ;
#11790=CARTESIAN_POINT ( 'NONE',  ( -3.662846001189865142, 195.5725841191952838, 40.89886208192143613 ) ) ;
#11791=CARTESIAN_POINT ( 'NONE',  ( -9.984503880673473830, 210.2968891136704315, 0.6511379180785656917 ) ) ;
#11792=CARTESIAN_POINT ( 'NONE',  ( 6.220909254589536808, 215.4770327129947702, 58.55113791807858092 ) ) ;
#11793=CARTESIAN_POINT ( 'NONE',  ( -8.015496119326597224, 209.5516654185217362, 17.64886208192143968 ) ) ;
#11800=CARTESIAN_POINT ( 'NONE',  ( -4.984841277089891776, 213.7757310962905990, 101.9488620819214475 ) ) ;
#11803=CARTESIAN_POINT ( 'NONE',  ( -0.05014649552807731031, 198.5883022060938572, 35.75113791807857666 ) ) ;
#11810=CARTESIAN_POINT ( 'NONE',  ( -10.01549611932653860, 203.7984951890123284, 0.3511379180785655363 ) ) ;
#11811=CARTESIAN_POINT ( 'NONE',  ( 10.01549611932659545, 203.7984951890123853, 58.14886208192142192 ) ) ;
#11814=CARTESIAN_POINT ( 'NONE',  ( 8.062137200540920645, 201.0835637161417822, 5.301137918078566713 ) ) ;
#11818=CARTESIAN_POINT ( 'NONE',  ( 8.015496119326595448, 204.4483345814782638, 79.14886208192143613 ) ) ;
#11821=DIRECTION ( 'NONE',  ( -0.9998603841633338929, 0.01669062914075312987, 0.0007969188393214247284 ) ) ;
#11825=CARTESIAN_POINT ( 'NONE',  ( 6.139770520408367460, 198.4640165459539389, 23.45113791807856884 ) ) ;
#11826=VERTEX_POINT ( 'NONE', #1549 ) ;
#11830=CARTESIAN_POINT ( 'NONE',  ( 0.05014649552807549926, 219.6175466908591716, 88.25113791807856956 ) ) ;
#11835=CARTESIAN_POINT ( 'NONE',  ( -7.375838497908014268, 196.7627149292498530, 68.04886208192144181 ) ) ;
#11836=CARTESIAN_POINT ( 'NONE',  ( -3.135527875058982783, 216.4958274776886924, 81.09886208192143897 ) ) ;
#11837=CARTESIAN_POINT ( 'NONE',  ( 12.01549611932659367, 203.1486557965466773, 13.14886208192143613 ) ) ;
#11839=CARTESIAN_POINT ( 'NONE',  ( 10.01549611932653860, 210.2015048109876716, 19.85113791807856387 ) ) ;
#11841=CARTESIAN_POINT ( 'NONE',  ( -3.135527875058982783, 216.4958274776886924, 87.09886208192143897 ) ) ;
#11845=CARTESIAN_POINT ( 'NONE',  ( -0.05014649552828365914, 215.4116977939061144, 75.24886208192143044 ) ) ;
#11848=B_SPLINE_CURVE_WITH_KNOTS ( 'NONE', 3,
 ( #27294, #17409, #3950, #9404 ),
 .UNSPECIFIED., .F., .F.,
 ( 4, 4 ),
 ( -0.0005136321342257200344, 1.626303258728256651E-18 ),
 .UNSPECIFIED. ) ;
#11855=CARTESIAN_POINT ( 'NONE',  ( -6.500168698208129925, 202.3363017425936050, 81.20113791807858661 ) ) ;
#11860=CARTESIAN_POINT ( 'NONE',  ( -8.000000000000008882, 206.9523078486584780, 53.49886208192144466 ) ) ;
#11867=CARTESIAN_POINT ( 'NONE',  ( 3.662846001190051659, 195.5725841191953691, 59.60113791807857808 ) ) ;
#11871=CARTESIAN_POINT ( 'NONE',  ( 9.680171189290831535, 199.9079932115568852, 2.301137918078565825 ) ) ;
#11872=CARTESIAN_POINT ( 'NONE',  ( 8.118202686958039038, 212.8392687619912635, 79.70113791807857240 ) ) ;
#11874=CARTESIAN_POINT ( 'NONE',  ( 3.753561863808876797, 195.6020594897209719, 40.59886208192143187 ) ) ;
#11875=CARTESIAN_POINT ( 'NONE',  ( 10.01549611932659367, 203.7984951890124421, 46.14886208192143613 ) ) ;
#11877=CARTESIAN_POINT ( 'NONE',  ( 7.456977232089302632, 217.1783343296989131, 82.55113791807858092 ) ) ;
#11878=CARTESIAN_POINT ( 'NONE',  ( 8.000000000000008882, 206.9523078486586485, 98.00113791807856956 ) ) ;
#11879=CARTESIAN_POINT ( 'NONE',  ( 3.044812012439969795, 216.5253028482143520, 63.39886208192144323 ) ) ;
#11880=AXIS2_PLACEMENT_3D ( 'NONE', #4407, #27566, #30476 ) ;
#11882=CARTESIAN_POINT ( 'NONE',  ( 7.456977232089471386, 196.8216656703012006, 70.44886208192144750 ) ) ;
#11886=CARTESIAN_POINT ( 'NONE',  ( 6.444103211790928043, 211.7408657792734061, 42.69886208192144039 ) ) ;
#11890=CARTESIAN_POINT ( 'NONE',  ( -9.335145149336232961, 207.8126765316083038, 102.7601261637465910 ) ) ;
#11891=CARTESIAN_POINT ( 'NONE',  ( -2.426778023690262742, 214.6231898156240163, 61.10113791807857808 ) ) ;
#11896=CARTESIAN_POINT ( 'NONE',  ( 6.220909254589681581, 198.5229672870052582, 40.44886208192141908 ) ) ;
#11901=CARTESIAN_POINT ( 'NONE',  ( -7.984503880673422316, 204.3529502787951628, 20.34886208192143542 ) ) ;
#11902=CARTESIAN_POINT ( 'NONE',  ( 8.062137200540920645, 201.0835637161417822, 62.30113791807858092 ) ) ;
#11904=CARTESIAN_POINT ( 'NONE',  ( -0.05014649552810635652, 196.4853777576173002, 44.75113791807858377 ) ) ;
#11907=CARTESIAN_POINT ( 'NONE',  ( 8.118202686958039038, 212.8392687619912635, 22.70113791807856884 ) ) ;
#11908=CARTESIAN_POINT ( 'NONE',  ( 8.015496119326595448, 204.4483345814782638, 97.14886208192146455 ) ) ;
#11911=CARTESIAN_POINT ( 'NONE',  ( -7.456977232089304408, 196.8216656703010301, 27.05113791807857027 ) ) ;
#11913=CARTESIAN_POINT ( 'NONE',  ( -10.00000000000000711, 207.0476921513413515, 78.50113791807856956 ) ) ;
#11914=CARTESIAN_POINT ( 'NONE',  ( 6.220909254589536808, 215.4770327129947987, 52.55113791807857382 ) ) ;
#11917=CARTESIAN_POINT ( 'NONE',  ( -3.753561863808878130, 218.3979405102790281, 3.098862081921434530 ) ) ;
#11918=CARTESIAN_POINT ( 'NONE',  ( 9.984503880673420539, 210.2968891136705736, 18.84886208192143542 ) ) ;
#11921=CARTESIAN_POINT ( 'NONE',  ( -9.736236675707914401, 199.9851607334237542, 54.20113791807856529 ) ) ;
#11923=CARTESIAN_POINT ( 'NONE',  ( -8.015496119326531499, 204.4483345814780364, 66.35113791807857808 ) ) ;
#11924=CARTESIAN_POINT ( 'NONE',  ( -10.01549611932659722, 210.2015048109875011, 29.64886208192143968 ) ) ;
#11929=CARTESIAN_POINT ( 'NONE',  ( 3.044812012440130555, 197.4746971517856764, 89.60113791807857808 ) ) ;
#11934=CARTESIAN_POINT ( 'NONE',  ( -4.903702542908602524, 213.8346818373418898, 36.95113791807857950 ) ) ;
#11936=CARTESIAN_POINT ( 'NONE',  ( -0.05014649552828403384, 217.5146222423826714, 15.24886208192143044 ) ) ;
#11939=CARTESIAN_POINT ( 'NONE',  ( 8.015496119326531499, 209.5516654185219636, 46.85113791807857098 ) ) ;
#11941=DIRECTION ( 'NONE',  ( 0.000000000000000000, 0.000000000000000000, 1.000000000000000000 ) ) ;
#11944=CARTESIAN_POINT ( 'NONE',  ( -9.984503880673420539, 203.7031108863293980, 89.34886208192143897 ) ) ;
#11946=CARTESIAN_POINT ( 'NONE',  ( -3.044812012440131443, 216.5253028482142952, 34.10113791807857808 ) ) ;
#11948=CARTESIAN_POINT ( 'NONE',  ( 3.044812012440130555, 197.4746971517856764, 14.60113791807856565 ) ) ;
#11953=CARTESIAN_POINT ( 'NONE',  ( -7.456977232089304408, 196.8216656703010301, 0.05113791807856556820 ) ) ;
#11955=CARTESIAN_POINT ( 'NONE',  ( 3.135527875058820690, 216.4958274776887492, 43.40113791807856813 ) ) ;
#11959=EDGE_LOOP ( 'NONE', ( #9405, #1783 ) ) ;
#11960=CARTESIAN_POINT ( 'NONE',  ( -0.05014649552807705357, 194.3824533091408000, 20.75113791807856600 ) ) ;
#11964=CARTESIAN_POINT ( 'NONE',  ( -9.736236675708031640, 214.0148392665760753, 38.79886208192142050 ) ) ;
#11965=CARTESIAN_POINT ( 'NONE',  ( 8.118202686958039038, 212.8392687619912635, 1.701137918078565736 ) ) ;
#11966=CARTESIAN_POINT ( 'NONE',  ( 8.118202686958039038, 212.8392687619912635, 64.70113791807857240 ) ) ;
#11967=CARTESIAN_POINT ( 'NONE',  ( 4.984841277089891776, 200.2242689037093726, 22.44886208192143329 ) ) ;
#11970=CARTESIAN_POINT ( 'NONE',  ( 2.517493886309087436, 199.4062855549015865, 97.59886208192145318 ) ) ;
#11972=CARTESIAN_POINT ( 'NONE',  ( -11.98450388067341876, 203.0532714938636047, 89.34886208192143897 ) ) ;
#11978=CARTESIAN_POINT ( 'NONE',  ( 8.062137200540822946, 212.9164362838583315, 57.69886208192144039 ) ) ;
#11981=CARTESIAN_POINT ( 'NONE',  ( -8.118202686958039038, 201.1607312380087080, 0.2011379180785657361 ) ) ;
#11985=CARTESIAN_POINT ( 'NONE',  ( 6.444103211790928043, 211.7408657792734061, 84.69886208192144750 ) ) ;
#11988=CARTESIAN_POINT ( 'NONE',  ( 7.456977232089471386, 196.8216656703012006, 88.44886208192144750 ) ) ;
#11991=CARTESIAN_POINT ( 'NONE',  ( 8.062137200540920645, 201.0835637161417822, 17.30113791807856671 ) ) ;
#11995=CARTESIAN_POINT ( 'NONE',  ( -12.00000000000000711, 207.0476921513413515, 87.50113791807856956 ) ) ;
#11999=CARTESIAN_POINT ( 'NONE',  ( 11.98450388067341876, 210.9467285061363953, 66.84886208192143897 ) ) ;
#12000=CARTESIAN_POINT ( 'NONE',  ( -9.984503880673420539, 203.7031108863293980, 80.34886208192143897 ) ) ;
#12001=CARTESIAN_POINT ( 'NONE',  ( -9.736236675708031640, 214.0148392665760753, 17.79886208192143471 ) ) ;
#12003=CARTESIAN_POINT ( 'NONE',  ( -6.220909254589537696, 198.5229672870051161, 36.05113791807857382 ) ) ;
#12005=CARTESIAN_POINT ( 'NONE',  ( -8.118202686958138514, 212.8392687619910930, 95.79886208192144181 ) ) ;
#12009=CARTESIAN_POINT ( 'NONE',  ( -6.444103211790928043, 202.2591342207265939, 68.19886208192143329 ) ) ;
#12017=CARTESIAN_POINT ( 'NONE',  ( -4.984841277089726574, 200.2242689037092305, 81.05113791807856671 ) ) ;
#12022=CARTESIAN_POINT ( 'NONE',  ( -6.444103211790928043, 202.2591342207265939, 56.19886208192144039 ) ) ;
#12029=CARTESIAN_POINT ( 'NONE',  ( 9.680171189290831535, 199.9079932115568852, 62.30113791807858092 ) ) ;
#12031=CARTESIAN_POINT ( 'NONE',  ( 11.98450388067348271, 203.0532714938637753, -0.8488620819214346414 ) ) ;
#12032=CARTESIAN_POINT ( 'NONE',  ( -8.118202686958039038, 201.1607312380087080, 81.20113791807857240 ) ) ;
#12034=CARTESIAN_POINT ( 'NONE',  ( 7.456977232089471386, 196.8216656703012006, 43.44886208192143329 ) ) ;
#12035=CARTESIAN_POINT ( 'NONE',  ( 6.220909254589680693, 198.5229672870052582, 46.44886208192142618 ) ) ;
#12038=CARTESIAN_POINT ( 'NONE',  ( -3.662846001190052991, 218.4274158808045740, 88.10113791807857808 ) ) ;
#12039=CARTESIAN_POINT ( 'NONE',  ( -10.00000000000000711, 207.0476921513413515, 3.501137918078566003 ) ) ;
#12040=CARTESIAN_POINT ( 'NONE',  ( 8.062137200540822946, 212.9164362838583315, 63.69886208192143329 ) ) ;
#12043=CARTESIAN_POINT ( 'NONE',  ( -12.01549611932659722, 210.8513442034533227, 71.64886208192143613 ) ) ;
#12047=CARTESIAN_POINT ( 'NONE',  ( 2.517493886309087436, 199.4062855549015865, 43.59886208192144608 ) ) ;
#12053=CARTESIAN_POINT ( 'NONE',  ( -7.984503880673488041, 209.6470497212046098, 63.65113791807855392 ) ) ;
#12055=CARTESIAN_POINT ( 'NONE',  ( -0.05014649552828403384, 217.5146222423826714, 42.24886208192143755 ) ) ;
#12058=( NAMED_UNIT ( * ) PLANE_ANGLE_UNIT ( ) SI_UNIT ( $, .RADIAN. ) );
#12061=CARTESIAN_POINT ( 'NONE',  ( 2.426778023690075337, 214.6231898156240447, 21.39886208192143613 ) ) ;
#12062=CARTESIAN_POINT ( 'NONE',  ( 3.044812012440130555, 197.4746971517856764, 65.60113791807857808 ) ) ;
#12063=CARTESIAN_POINT ( 'NONE',  ( 3.044812012440130555, 197.4746971517856764, 50.60113791807857808 ) ) ;
#12066=CARTESIAN_POINT ( 'NONE',  ( 8.062137200540920645, 201.0835637161417822, 14.30113791807856671 ) ) ;
#12068=CARTESIAN_POINT ( 'NONE',  ( 6.444103211791042618, 202.2591342207267644, 5.301137918078567601 ) ) ;
#12072=CARTESIAN_POINT ( 'NONE',  ( -11.98450388067348804, 210.9467285061362247, 30.65113791807856458 ) ) ;
#12074=CARTESIAN_POINT ( 'NONE',  ( 6.139770520408368348, 198.4640165459539674, 74.45113791807857240 ) ) ;
#12075=CARTESIAN_POINT ( 'NONE',  ( -8.118202686958039038, 201.1607312380087080, 51.20113791807857240 ) ) ;
#12078=CARTESIAN_POINT ( 'NONE',  ( -7.375838497908014268, 196.7627149292498530, 11.04886208192143648 ) ) ;
#12079=CARTESIAN_POINT ( 'NONE',  ( -8.118202686958138514, 212.8392687619910930, 17.79886208192143826 ) ) ;
#12083=CARTESIAN_POINT ( 'NONE',  ( 12.01549611932652972, 210.8513442034534933, 61.85113791807857098 ) ) ;
#12084=CARTESIAN_POINT ( 'NONE',  ( 6.500168698208129925, 211.6636982574063381, 70.70113791807857240 ) ) ;
#12086=CARTESIAN_POINT ( 'NONE',  ( -6.220909254589682469, 215.4770327129946850, 26.94886208192142618 ) ) ;
#12097=CARTESIAN_POINT ( 'NONE',  ( -0.05014649552807731031, 198.5883022060938572, 29.75113791807856956 ) ) ;
#12100=CARTESIAN_POINT ( 'NONE',  ( -10.01549611932659722, 210.2015048109875011, 11.64886208192143258 ) ) ;
#12103=CARTESIAN_POINT ( 'NONE',  ( -6.500168698208129925, 202.3363017425936050, 54.20113791807857240 ) ) ;
#12107=CARTESIAN_POINT ( 'NONE',  ( 8.062137200540822946, 212.9164362838583315, 102.6988620819214475 ) ) ;
#12110=CARTESIAN_POINT ( 'NONE',  ( -3.135527875058821579, 197.5041725223112223, 29.90113791807856813 ) ) ;
#12112=CARTESIAN_POINT ( 'NONE',  ( 8.062137200540920645, 201.0835637161417822, 17.30113791807856671 ) ) ;
#12118=CARTESIAN_POINT ( 'NONE',  ( 9.984503880673470277, 203.7031108863295401, 101.1511379180785752 ) ) ;
#12121=CARTESIAN_POINT ( 'NONE',  ( -3.044812012440131443, 216.5253028482142952, 43.10113791807857808 ) ) ;
#12127=CARTESIAN_POINT ( 'NONE',  ( 3.753561863808689836, 218.3979405102790565, 25.40113791807857169 ) ) ;
#12129=CARTESIAN_POINT ( 'NONE',  ( 6.220909254589681581, 198.5229672870052582, 4.448862081921432399 ) ) ;
#12133=CARTESIAN_POINT ( 'NONE',  ( -8.062137200540920645, 212.9164362838581894, 0.8011379180785658249 ) ) ;
#12134=CARTESIAN_POINT ( 'NONE',  ( 8.062137200540920645, 201.0835637161417822, 62.30113791807858092 ) ) ;
#12136=CARTESIAN_POINT ( 'NONE',  ( 2.517493886309087436, 199.4062855549015865, 22.59886208192143542 ) ) ;
#12139=CARTESIAN_POINT ( 'NONE',  ( -0.05014649552807731031, 198.5883022060938572, 5.751137918078564226 ) ) ;
#12141=CARTESIAN_POINT ( 'NONE',  ( 7.456977232089471386, 196.8216656703012006, 85.44886208192144750 ) ) ;
#12146=CARTESIAN_POINT ( 'NONE',  ( -0.05014649552810635652, 196.4853777576173002, -0.2488620819214343305 ) ) ;
#12147=CARTESIAN_POINT ( 'NONE',  ( 0.05014649552828275708, 196.4853777576173002, 67.74886208192140202 ) ) ;
#12150=CARTESIAN_POINT ( 'NONE',  ( -9.984503880673473830, 210.2968891136704315, 3.651137918078565026 ) ) ;
#12152=CARTESIAN_POINT ( 'NONE',  ( -10.47863426674271814, 207.9189531262114770, 102.6635298682156758 ) ) ;
#12155=CARTESIAN_POINT ( 'NONE',  ( -8.118202686958039038, 201.1607312380087080, 90.20113791807857240 ) ) ;
#12157=CARTESIAN_POINT ( 'NONE',  ( -2.517493886309087880, 214.5937144450984135, 87.09886208192143897 ) ) ;
#12161=CARTESIAN_POINT ( 'NONE',  ( 7.456977232089471386, 196.8216656703012006, 85.44886208192144750 ) ) ;
#12164=CARTESIAN_POINT ( 'NONE',  ( -8.118202686958039038, 201.1607312380087080, 21.20113791807856529 ) ) ;
#12168=CARTESIAN_POINT ( 'NONE',  ( 12.00000000000000711, 206.9523078486586485, 83.00113791807856956 ) ) ;
#12171=CARTESIAN_POINT ( 'NONE',  ( 12.00000000000000711, 207.0476921513415220, 66.99886208192144466 ) ) ;
#12173=CARTESIAN_POINT ( 'NONE',  ( -10.00000000000000711, 206.9523078486584495, 74.49886208192144466 ) ) ;
#12174=CARTESIAN_POINT ( 'NONE',  ( 9.680171189290716072, 214.0920067884432854, 15.69886208192143684 ) ) ;
#12176=CARTESIAN_POINT ( 'NONE',  ( -8.062137200540920645, 212.9164362838581894, 36.80113791807856671 ) ) ;
#12178=CARTESIAN_POINT ( 'NONE',  ( 0.05014649552828275708, 196.4853777576173002, 94.74886208192141623 ) ) ;
#12183=CARTESIAN_POINT ( 'NONE',  ( 6.500168698208244500, 202.3363017425938324, 85.29886208192145602 ) ) ;
#12192=CARTESIAN_POINT ( 'NONE',  ( -2.426778023690262742, 214.6231898156240163, 82.10113791807857808 ) ) ;
#12196=CARTESIAN_POINT ( 'NONE',  ( 2.426778023690075337, 214.6231898156240447, 57.39886208192144323 ) ) ;
#12202=CARTESIAN_POINT ( 'NONE',  ( -9.680171189290831535, 214.0920067884431148, 54.80113791807857382 ) ) ;
#12204=CARTESIAN_POINT ( 'NONE',  ( -0.05014649552810635652, 196.4853777576173002, 101.7511379180785411 ) ) ;
#12205=CARTESIAN_POINT ( 'NONE',  ( 0.05014649552810506589, 217.5146222423826714, 82.25113791807856956 ) ) ;
#12206=CARTESIAN_POINT ( 'NONE',  ( 7.375838497908012492, 217.2372850707501186, 45.54886208192143471 ) ) ;
#12207=CARTESIAN_POINT ( 'NONE',  ( -3.044812012439970683, 197.4746971517856196, 43.89886208192142902 ) ) ;
#12209=CARTESIAN_POINT ( 'NONE',  ( 9.680171189290831535, 199.9079932115568852, 86.30113791807858092 ) ) ;
#12211=CARTESIAN_POINT ( 'NONE',  ( 0.05014649552810505201, 217.5146222423826714, 7.251137918078566003 ) ) ;
#12212=CARTESIAN_POINT ( 'NONE',  ( 9.984503880673420539, 210.2968891136705167, 69.84886208192143897 ) ) ;
#12215=CARTESIAN_POINT ( 'NONE',  ( -3.753561863808878130, 218.3979405102790281, 75.09886208192142476 ) ) ;
#12218=CARTESIAN_POINT ( 'NONE',  ( 6.444103211790928043, 211.7408657792734061, 48.69886208192144750 ) ) ;
#12226=CARTESIAN_POINT ( 'NONE',  ( -3.135527875058982783, 216.4958274776886924, 42.09886208192143897 ) ) ;
#12229=ADVANCED_FACE ( 'NONE', ( #6866 ), #21389, .T. ) ;
#12232=CARTESIAN_POINT ( 'NONE',  ( 2.426778023690075337, 214.6231898156240447, 24.39886208192143258 ) ) ;
#12233=CARTESIAN_POINT ( 'NONE',  ( -10.00000000000000711, 207.0476921513413515, 63.50113791807856956 ) ) ;
#12234=CARTESIAN_POINT ( 'NONE',  ( 3.135527875058820690, 216.4958274776887492, 43.40113791807856813 ) ) ;
#12236=CARTESIAN_POINT ( 'NONE',  ( -9.984503880673473830, 210.2968891136704315, 18.65113791807856813 ) ) ;
#12237=CARTESIAN_POINT ( 'NONE',  ( -6.444103211791042618, 211.7408657792732356, 6.801137918078567601 ) ) ;
#12241=CARTESIAN_POINT ( 'NONE',  ( -11.98450388067348804, 210.9467285061362247, 24.65113791807857169 ) ) ;
#12244=CARTESIAN_POINT ( 'NONE',  ( 10.00000000000000711, 206.9523078486586201, 80.00113791807856956 ) ) ;
#12245=CARTESIAN_POINT ( 'NONE',  ( -6.139770520408368348, 215.5359834540460042, 51.95113791807857240 ) ) ;
#12248=CARTESIAN_POINT ( 'NONE',  ( 11.98450388067341876, 210.9467285061363953, 12.84886208192143719 ) ) ;
#12249=CARTESIAN_POINT ( 'NONE',  ( -8.118202686958138514, 212.8392687619910930, 14.79886208192143648 ) ) ;
#12252=CARTESIAN_POINT ( 'NONE',  ( 9.680171189290831535, 199.9079932115568852, 56.30113791807857382 ) ) ;
#12253=CARTESIAN_POINT ( 'NONE',  ( 8.015496119326531499, 209.5516654185219636, 79.85113791807857808 ) ) ;
#12255=CARTESIAN_POINT ( 'NONE',  ( -8.118202686958138514, 212.8392687619910930, 41.79886208192143471 ) ) ;
#12263=CARTESIAN_POINT ( 'NONE',  ( -4.903702542908602524, 213.8346818373418898, 33.95113791807857240 ) ) ;
#12265=CARTESIAN_POINT ( 'NONE',  ( 10.00000000000000711, 207.0476921513415220, 12.99886208192143400 ) ) ;
#12268=CARTESIAN_POINT ( 'NONE',  ( 8.000000000000008882, 206.9523078486586485, 47.00113791807856956 ) ) ;
#12272=CARTESIAN_POINT ( 'NONE',  ( -3.135527875058982783, 216.4958274776886924, 96.09886208192143897 ) ) ;
#12274=CARTESIAN_POINT ( 'NONE',  ( 10.00000000000000711, 206.9523078486586201, 29.00113791807856956 ) ) ;
#12278=CARTESIAN_POINT ( 'NONE',  ( 8.118202686958039038, 212.8392687619912635, 13.70113791807856707 ) ) ;
#12283=CARTESIAN_POINT ( 'NONE',  ( 11.98450388067348271, 203.0532714938637753, -0.8488620819214346414 ) ) ;
#12287=CARTESIAN_POINT ( 'NONE',  ( 10.01549611932653860, 210.2015048109876716, 49.85113791807857808 ) ) ;
#12293=CARTESIAN_POINT ( 'NONE',  ( 7.456977232089302632, 217.1783343296989131, 31.55113791807857027 ) ) ;
#12295=CARTESIAN_POINT ( 'NONE',  ( 4.922818201202977306, 207.4297999410988780, -9.402818167433192542 ) ) ;
#12296=CARTESIAN_POINT ( 'NONE',  ( -10.01549611932659722, 210.2015048109875011, 2.648862081921434797 ) ) ;
#12299=CARTESIAN_POINT ( 'NONE',  ( 6.139770520408368348, 198.4640165459539674, -0.5488620819214343749 ) ) ;
#12300=CARTESIAN_POINT ( 'NONE',  ( -8.118202686958039038, 201.1607312380087080, 66.20113791807857240 ) ) ;
#12302=CARTESIAN_POINT ( 'NONE',  ( -0.05014649552828365914, 215.4116977939061144, 24.24886208192144110 ) ) ;
#12305=CARTESIAN_POINT ( 'NONE',  ( 4.903702542908601636, 200.1653181626581102, 2.451137918078566180 ) ) ;
#12308=CARTESIAN_POINT ( 'NONE',  ( -0.05014649552828442242, 219.6175466908591716, 84.24886208192143044 ) ) ;
#12313=CARTESIAN_POINT ( 'NONE',  ( 10.00000000000000711, 206.9523078486586201, 2.001137918078565558 ) ) ;
#12315=CARTESIAN_POINT ( 'NONE',  ( -8.062137200540822946, 201.0835637161416400, 71.19886208192144750 ) ) ;
#12318=CARTESIAN_POINT ( 'NONE',  ( -10.00000000000000711, 207.0476921513413515, 0.5011379180785656695 ) ) ;
#12323=CARTESIAN_POINT ( 'NONE',  ( -6.220909254589537696, 198.5229672870051161, 90.05113791807858092 ) ) ;
#12325=CARTESIAN_POINT ( 'NONE',  ( -10.01549611932653860, 203.7984951890123284, 78.35113791807857808 ) ) ;
#12328=CARTESIAN_POINT ( 'NONE',  ( -12.01549611932659722, 210.8513442034533227, 89.64886208192142192 ) ) ;
#12330=CARTESIAN_POINT ( 'NONE',  ( 6.139770520408367460, 198.4640165459539389, 17.45113791807856174 ) ) ;
#12334=CARTESIAN_POINT ( 'NONE',  ( -12.01549611932652972, 203.1486557965464499, 90.35113791807857808 ) ) ;
#12338=CARTESIAN_POINT ( 'NONE',  ( -3.662846001189865142, 195.5725841191952838, 73.89886208192143613 ) ) ;
#12340=CARTESIAN_POINT ( 'NONE',  ( 6.139770520408223575, 215.5359834540460611, 81.54886208192144181 ) ) ;
#12341=CARTESIAN_POINT ( 'NONE',  ( 9.680171189290716072, 214.0920067884432854, 9.698862081921433287 ) ) ;
#12343=CARTESIAN_POINT ( 'NONE',  ( -8.118202686958039038, 201.1607312380087080, 33.20113791807857240 ) ) ;
#12345=CARTESIAN_POINT ( 'NONE',  ( 10.01549611932659545, 203.7984951890123853, 97.14886208192145034 ) ) ;
#12350=CARTESIAN_POINT ( 'NONE',  ( 0.05014649552828262524, 198.5883022060938572, 76.74886208192144466 ) ) ;
#12358=FACE_OUTER_BOUND ( 'NONE', #2593, .T. ) ;
#12359=CARTESIAN_POINT ( 'NONE',  ( -8.000000000000008882, 207.0476921513413515, 75.50113791807856956 ) ) ;
#12363=CARTESIAN_POINT ( 'NONE',  ( 7.984503880673422316, 209.6470497212048372, 57.84886208192144608 ) ) ;
#12364=TOROIDAL_SURFACE ( 'NONE', #2606, 4.999999999999993783, 1.000000000000000222 ) ;
#12370=CARTESIAN_POINT ( 'NONE',  ( -12.01549611932652972, 203.1486557965464499, 57.35113791807857098 ) ) ;
#12372=CARTESIAN_POINT ( 'NONE',  ( -11.98450388067348804, 210.9467285061362247, 3.651137918078566358 ) ) ;
#12374=CARTESIAN_POINT ( 'NONE',  ( 8.118202686958039038, 212.8392687619912635, 73.70113791807857240 ) ) ;
#12375=CARTESIAN_POINT ( 'NONE',  ( -3.662846001189865142, 195.5725841191952838, 46.89886208192143613 ) ) ;
#12376=CARTESIAN_POINT ( 'NONE',  ( 6.139770520408223575, 215.5359834540460611, 45.54886208192144181 ) ) ;
#12377=CARTESIAN_POINT ( 'NONE',  ( 12.01549611932652972, 210.8513442034534933, 85.85113791807857808 ) ) ;
#12380=CARTESIAN_POINT ( 'NONE',  ( -6.220909254589537696, 198.5229672870051161, 0.05113791807856577637 ) ) ;
#12381=CARTESIAN_POINT ( 'NONE',  ( 3.044812012439969795, 216.5253028482143520, 72.39886208192143613 ) ) ;
#12385=CARTESIAN_POINT ( 'NONE',  ( 0.05014649552828288198, 194.3824533091408000, 73.74886208192144466 ) ) ;
#12388=CARTESIAN_POINT ( 'NONE',  ( 7.984503880673422316, 209.6470497212048372, 48.84886208192143897 ) ) ;
#12395=CARTESIAN_POINT ( 'NONE',  ( -9.521242624480144912, 207.9188892840786878, 102.6634595774070533 ) ) ;
#12397=CARTESIAN_POINT ( 'NONE',  ( -8.118202686958138514, 212.8392687619910930, 38.79886208192143471 ) ) ;
#12402=CARTESIAN_POINT ( 'NONE',  ( 0.05014649552828262524, 198.5883022060938572, 25.74886208192143755 ) ) ;
#12404=CARTESIAN_POINT ( 'NONE',  ( -8.118202686958039038, 201.1607312380087080, 75.20113791807857240 ) ) ;
#12406=CARTESIAN_POINT ( 'NONE',  ( 6.220909254589536808, 215.4770327129947702, 43.55113791807857382 ) ) ;
#12407=AXIS2_PLACEMENT_3D ( 'NONE', #17291, #15865, #2929 ) ;
#12409=CARTESIAN_POINT ( 'NONE',  ( -6.139770520408369237, 215.5359834540460042, 21.95113791807856884 ) ) ;
#12410=CARTESIAN_POINT ( 'NONE',  ( -4.903702542908602524, 213.8346818373418898, 0.9511379180785658471 ) ) ;
#12412=CARTESIAN_POINT ( 'NONE',  ( 7.456977232089302632, 217.1783343296989131, 31.55113791807857027 ) ) ;
#12414=CARTESIAN_POINT ( 'NONE',  ( 6.220909254589536808, 215.4770327129947702, 76.55113791807855250 ) ) ;
#12416=CARTESIAN_POINT ( 'NONE',  ( 3.135527875058820690, 216.4958274776887492, 46.40113791807857524 ) ) ;
#12420=CARTESIAN_POINT ( 'NONE',  ( 9.680171189290716072, 214.0920067884432854, 12.69886208192143684 ) ) ;
#12421=CARTESIAN_POINT ( 'NONE',  ( -6.139770520408224463, 198.4640165459539105, 23.04886208192143471 ) ) ;
#12424=CARTESIAN_POINT ( 'NONE',  ( -11.98450388067348804, 210.9467285061362247, 60.65113791807856813 ) ) ;
#12426=CARTESIAN_POINT ( 'NONE',  ( -8.000000000000008882, 207.0476921513413515, 78.50113791807856956 ) ) ;
#12427=CARTESIAN_POINT ( 'NONE',  ( -3.135527875058982783, 216.4958274776886924, 36.09886208192143897 ) ) ;
#12438=CARTESIAN_POINT ( 'NONE',  ( -8.015496119326531499, 204.4483345814780364, 36.35113791807857098 ) ) ;
#12440=CARTESIAN_POINT ( 'NONE',  ( -3.044812012439970683, 197.4746971517856196, 13.89886208192143613 ) ) ;
#12444=CARTESIAN_POINT ( 'NONE',  ( 2.426778023690261410, 199.3768101843759837, 62.60113791807857808 ) ) ;
#12447=CARTESIAN_POINT ( 'NONE',  ( 0.05014649552828275708, 196.4853777576173002, 97.74886208192140202 ) ) ;
#12450=CARTESIAN_POINT ( 'NONE',  ( -3.135527875058821579, 197.5041725223112223, 41.90113791807856813 ) ) ;
#12452=CARTESIAN_POINT ( 'NONE',  ( -6.220909254589537696, 198.5229672870051161, 18.05113791807856671 ) ) ;
#12455=CARTESIAN_POINT ( 'NONE',  ( -9.898309971686792608, 228.3698647632124334, 103.4854814124440452 ) ) ;
#12459=CARTESIAN_POINT ( 'NONE',  ( -3.135527875058821579, 197.5041725223112223, 50.90113791807856813 ) ) ;
#12466=CARTESIAN_POINT ( 'NONE',  ( -11.98450388067348804, 210.9467285061362247, 33.65113791807856813 ) ) ;
#12468=CARTESIAN_POINT ( 'NONE',  ( -8.062137200540822946, 201.0835637161416400, 8.198862081921435063 ) ) ;
#12472=CARTESIAN_POINT ( 'NONE',  ( -3.135527875058821579, 197.5041725223112223, 8.901137918078566358 ) ) ;
#12473=CARTESIAN_POINT ( 'NONE',  ( -6.220909254589537696, 198.5229672870051161, 60.05113791807855961 ) ) ;
#12475=CARTESIAN_POINT ( 'NONE',  ( 6.500168698208244500, 202.3363017425938324, 19.29886208192143471 ) ) ;
#12480=CARTESIAN_POINT ( 'NONE',  ( -8.015496119326531499, 204.4483345814780364, 6.351137918078565647 ) ) ;
#12484=CARTESIAN_POINT ( 'NONE',  ( -7.456977232089471386, 217.1783343296987709, 92.94886208192144750 ) ) ;
#12489=CARTESIAN_POINT ( 'NONE',  ( 8.062137200540920645, 201.0835637161417822, 2.301137918078566269 ) ) ;
#12490=CARTESIAN_POINT ( 'NONE',  ( -8.062137200540822946, 201.0835637161416400, 68.19886208192144750 ) ) ;
#12493=CARTESIAN_POINT ( 'NONE',  ( 3.135527875058820690, 216.4958274776887492, 4.401137918078565470 ) ) ;
#12496=CARTESIAN_POINT ( 'NONE',  ( -0.05014649552810635652, 196.4853777576173002, 86.75113791807858377 ) ) ;
#12498=CARTESIAN_POINT ( 'NONE',  ( -8.062137200540920645, 212.9164362838581894, 72.80113791807856671 ) ) ;
#12501=CARTESIAN_POINT ( 'NONE',  ( -7.375838497908014268, 196.7627149292498530, 86.04886208192145602 ) ) ;
#12503=CARTESIAN_POINT ( 'NONE',  ( 6.220909254589536808, 215.4770327129947987, 34.55113791807856671 ) ) ;
#12508=CARTESIAN_POINT ( 'NONE',  ( 9.680171189290831535, 199.9079932115568852, 98.30113791807858092 ) ) ;
#12512=CARTESIAN_POINT ( 'NONE',  ( -10.00000000000000711, 206.9523078486584495, 86.49886208192144466 ) ) ;
#12513=CARTESIAN_POINT ( 'NONE',  ( 11.98450388067341876, 210.9467285061363953, 27.84886208192143897 ) ) ;
#12515=CARTESIAN_POINT ( 'NONE',  ( -6.139770520408369237, 215.5359834540460042, 30.95113791807857240 ) ) ;
#12517=CARTESIAN_POINT ( 'NONE',  ( -8.062137200540822946, 201.0835637161416400, 95.19886208192143329 ) ) ;
#12523=CARTESIAN_POINT ( 'NONE',  ( -6.444103211790928043, 202.2591342207265939, 80.19886208192143329 ) ) ;
#12525=ORIENTED_EDGE ( 'NONE', *, *, #5713, .F. ) ;
#12531=CARTESIAN_POINT ( 'NONE',  ( 4.984841277089725686, 213.7757310962907411, 76.55113791807858092 ) ) ;
#12534=CARTESIAN_POINT ( 'NONE',  ( -6.500168698208244500, 211.6636982574061676, 53.79886208192144892 ) ) ;
#12540=CARTESIAN_POINT ( 'NONE',  ( -11.98450388067348804, 210.9467285061362247, 66.65113791807856103 ) ) ;
#12542=CARTESIAN_POINT ( 'NONE',  ( -3.753561863808691168, 195.6020594897209435, 8.901137918078566358 ) ) ;
#12543=CARTESIAN_POINT ( 'NONE',  ( -0.05014649552810635652, 196.4853777576173002, 74.75113791807858377 ) ) ;
#12544=CARTESIAN_POINT ( 'NONE',  ( -3.662846001189865142, 195.5725841191952838, 40.89886208192143613 ) ) ;
#12545=CARTESIAN_POINT ( 'NONE',  ( -8.062137200540822946, 201.0835637161416400, 53.19886208192143329 ) ) ;
#12547=CARTESIAN_POINT ( 'NONE',  ( 7.375838497908181246, 196.7627149292499666, 86.45113791807858661 ) ) ;
#12549=CARTESIAN_POINT ( 'NONE',  ( -8.062137200540920645, 212.9164362838581894, 3.801137918078565825 ) ) ;
#12550=CARTESIAN_POINT ( 'NONE',  ( 10.01549611932659545, 203.7984951890123853, 67.14886208192143613 ) ) ;
#12553=CARTESIAN_POINT ( 'NONE',  ( 11.98450388067341876, 210.9467285061363953, 72.84886208192143897 ) ) ;
#12554=CARTESIAN_POINT ( 'NONE',  ( -10.00000000000000711, 207.0476921513413515, 87.50113791807858377 ) ) ;
#12558=CARTESIAN_POINT ( 'NONE',  ( -2.426778023690076225, 199.3768101843759553, 49.89886208192144323 ) ) ;
#12566=CARTESIAN_POINT ( 'NONE',  ( -10.00000000000000711, 206.9523078486584495, 53.49886208192143755 ) ) ;
#12571=CARTESIAN_POINT ( 'NONE',  ( -8.000000000000008882, 206.9523078486584780, 20.49886208192143755 ) ) ;
#12572=CARTESIAN_POINT ( 'NONE',  ( -8.062137200540920645, 212.9164362838581894, 72.80113791807856671 ) ) ;
#12574=CARTESIAN_POINT ( 'NONE',  ( -10.01549611932653860, 203.7984951890123284, 60.35113791807857808 ) ) ;
#12575=CARTESIAN_POINT ( 'NONE',  ( -6.220909254589537696, 198.5229672870051161, 15.05113791807856671 ) ) ;
#12576=CARTESIAN_POINT ( 'NONE',  ( -0.05014649552807731031, 198.5883022060938572, 8.751137918078567779 ) ) ;
#12579=CARTESIAN_POINT ( 'NONE',  ( -12.00000000000000711, 207.0476921513413515, 33.50113791807857666 ) ) ;
#12581=CARTESIAN_POINT ( 'NONE',  ( 6.139770520408368348, 198.4640165459539674, 86.45113791807854398 ) ) ;
#12582=CARTESIAN_POINT ( 'NONE',  ( -8.062137200540920645, 212.9164362838581894, 48.80113791807857382 ) ) ;
#12584=CARTESIAN_POINT ( 'NONE',  ( 3.662846001189864698, 218.4274158808046593, 9.398862081921436129 ) ) ;
#12585=CARTESIAN_POINT ( 'NONE',  ( -3.044812012439970683, 197.4746971517856196, 28.89886208192143613 ) ) ;
#12588=CARTESIAN_POINT ( 'NONE',  ( -0.05014649552807705357, 194.3824533091408000, 53.75113791807857666 ) ) ;
#12589=CARTESIAN_POINT ( 'NONE',  ( -7.984503880673488041, 209.6470497212046098, 75.65113791807856103 ) ) ;
#12590=CARTESIAN_POINT ( 'NONE',  ( 3.044812012439969795, 216.5253028482143520, 42.39886208192143613 ) ) ;
#12593=CARTESIAN_POINT ( 'NONE',  ( 11.98450388067341876, 210.9467285061363953, 45.84886208192143187 ) ) ;
#12600=CARTESIAN_POINT ( 'NONE',  ( -8.015496119326531499, 204.4483345814780364, 33.35113791807857098 ) ) ;
#12603=CARTESIAN_POINT ( 'NONE',  ( -6.139770520408224463, 198.4640165459539389, 17.04886208192143826 ) ) ;
#12606=CARTESIAN_POINT ( 'NONE',  ( -8.015496119326531499, 204.4483345814780364, 60.35113791807857098 ) ) ;
#12607=FACE_OUTER_BOUND ( 'NONE', #31587, .T. ) ;
#12609=CARTESIAN_POINT ( 'NONE',  ( 8.118202686958138514, 201.1607312380088501, 97.29886208192144181 ) ) ;
#12611=CARTESIAN_POINT ( 'NONE',  ( 10.01549611932653860, 210.2015048109876716, 43.85113791807854966 ) ) ;
#12613=CARTESIAN_POINT ( 'NONE',  ( -3.135527875058821579, 197.5041725223112223, 14.90113791807856636 ) ) ;
#12620=CARTESIAN_POINT ( 'NONE',  ( -0.05014649552810635652, 196.4853777576173002, 101.7511379180785411 ) ) ;
#12623=CARTESIAN_POINT ( 'NONE',  ( -3.044812012440131443, 216.5253028482142952, 49.10113791807857808 ) ) ;
#12629=CARTESIAN_POINT ( 'NONE',  ( 12.01549611932652972, 210.8513442034534933, 25.85113791807856742 ) ) ;
#12630=CARTESIAN_POINT ( 'NONE',  ( 8.118202686958138514, 201.1607312380088501, 16.29886208192143471 ) ) ;
#12633=CARTESIAN_POINT ( 'NONE',  ( 6.220909254589536808, 215.4770327129947702, 10.55113791807856138 ) ) ;
#12634=CARTESIAN_POINT ( 'NONE',  ( -9.984503880673473830, 210.2968891136704315, 75.65113791807858945 ) ) ;
#12637=CARTESIAN_POINT ( 'NONE',  ( 8.015496119326595448, 204.4483345814782638, 25.14886208192143258 ) ) ;
#12641=CARTESIAN_POINT ( 'NONE',  ( -2.426778023690262742, 214.6231898156240163, 4.101137918078565647 ) ) ;
#12644=CARTESIAN_POINT ( 'NONE',  ( 3.753561863808876797, 195.6020594897209719, 88.59886208192143897 ) ) ;
#12649=CARTESIAN_POINT ( 'NONE',  ( -6.220909254589537696, 198.5229672870051161, 9.051137918078561384 ) ) ;
#12650=CARTESIAN_POINT ( 'NONE',  ( -3.135527875058982783, 216.4958274776886924, 69.09886208192143897 ) ) ;
#12653=CARTESIAN_POINT ( 'NONE',  ( -6.220909254589537696, 198.5229672870051161, 15.05113791807856671 ) ) ;
#12658=CARTESIAN_POINT ( 'NONE',  ( 3.044812012440130555, 197.4746971517856764, 101.6011379180785781 ) ) ;
#12660=CARTESIAN_POINT ( 'NONE',  ( -9.984503880673473830, 210.2968891136704315, 75.65113791807858945 ) ) ;
#12663=CARTESIAN_POINT ( 'NONE',  ( 3.662846001189864698, 218.4274158808046593, 87.39886208192143613 ) ) ;
#12665=CARTESIAN_POINT ( 'NONE',  ( 8.062137200540920645, 201.0835637161417822, 26.30113791807856671 ) ) ;
#12670=CARTESIAN_POINT ( 'NONE',  ( -7.375838497908182134, 217.2372850707499765, 93.95113791807857240 ) ) ;
#12675=CARTESIAN_POINT ( 'NONE',  ( -8.062137200540822946, 201.0835637161416400, 86.19886208192144750 ) ) ;
#12676=CARTESIAN_POINT ( 'NONE',  ( 11.98450388067341876, 210.9467285061363953, 24.84886208192143897 ) ) ;
#12678=CARTESIAN_POINT ( 'NONE',  ( 3.044812012440130555, 197.4746971517856764, 35.60113791807857098 ) ) ;
#12681=CARTESIAN_POINT ( 'NONE',  ( -0.05014649552828403384, 217.5146222423826714, 96.24886208192144466 ) ) ;
#12686=CARTESIAN_POINT ( 'NONE',  ( -2.517493886309087880, 214.5937144450984135, 78.09886208192142476 ) ) ;
#12691=CARTESIAN_POINT ( 'NONE',  ( 0.05014649552807626948, 215.4116977939061144, 58.25113791807857666 ) ) ;
#12692=AXIS2_PLACEMENT_3D ( 'NONE', #13237, #956, #10862 ) ;
#12696=CARTESIAN_POINT ( 'NONE',  ( -7.984503880673488041, 209.6470497212046098, 90.65113791807857524 ) ) ;
#12700=CARTESIAN_POINT ( 'NONE',  ( 6.444103211790928043, 211.7408657792734061, 66.69886208192143329 ) ) ;
#12709=CARTESIAN_POINT ( 'NONE',  ( -7.456977232089304408, 196.8216656703010301, 69.05113791807856671 ) ) ;
#12712=CARTESIAN_POINT ( 'NONE',  ( 3.753561863808689836, 218.3979405102790565, 13.40113791807856636 ) ) ;
#12714=CARTESIAN_POINT ( 'NONE',  ( 3.044812012440130555, 197.4746971517856764, 83.60113791807857808 ) ) ;
#12715=CARTESIAN_POINT ( 'NONE',  ( -7.456977232089471386, 217.1783343296987709, 50.94886208192143329 ) ) ;
#12716=CARTESIAN_POINT ( 'NONE',  ( 6.220909254589680693, 198.5229672870052582, 55.44886208192142618 ) ) ;
#12719=CARTESIAN_POINT ( 'NONE',  ( 3.662846001190051659, 195.5725841191953691, 95.60113791807857808 ) ) ;
#12721=CARTESIAN_POINT ( 'NONE',  ( 6.139770520408368348, 198.4640165459539674, -0.5488620819214343749 ) ) ;
#12724=CARTESIAN_POINT ( 'NONE',  ( 3.135527875058981895, 197.5041725223112792, 70.59886208192143897 ) ) ;
#12728=CARTESIAN_POINT ( 'NONE',  ( 9.736236675708031640, 199.9851607334238963, 76.29886208192142760 ) ) ;
#12729=CARTESIAN_POINT ( 'NONE',  ( -3.135527875058821579, 197.5041725223112223, 92.90113791807857524 ) ) ;
#12733=CARTESIAN_POINT ( 'NONE',  ( 8.000000000000008882, 207.0476921513415220, 48.99886208192144466 ) ) ;
#12740=CARTESIAN_POINT ( 'NONE',  ( -6.220909254589682469, 215.4770327129946850, 56.94886208192141908 ) ) ;
#12746=CARTESIAN_POINT ( 'NONE',  ( 8.015496119326595448, 204.4483345814782638, 31.14886208192143968 ) ) ;
#12748=CARTESIAN_POINT ( 'NONE',  ( -10.01549611932653860, 203.7984951890123284, 72.35113791807859229 ) ) ;
#12750=CARTESIAN_POINT ( 'NONE',  ( 10.01549611932653860, 210.2015048109876716, 55.85113791807857808 ) ) ;
#12751=CARTESIAN_POINT ( 'NONE',  ( 6.220909254589536808, 215.4770327129947702, 25.55113791807856671 ) ) ;
#12752=CARTESIAN_POINT ( 'NONE',  ( 2.426778023690261410, 199.3768101843759837, 5.601137918078567424 ) ) ;
#12756=CARTESIAN_POINT ( 'NONE',  ( -3.753561863808691168, 195.6020594897209435, 35.90113791807856813 ) ) ;
#12758=CARTESIAN_POINT ( 'NONE',  ( -10.01549611932653860, 203.7984951890123284, 87.35113791807854966 ) ) ;
#12759=CARTESIAN_POINT ( 'NONE',  ( 3.044812012440130555, 197.4746971517856764, 62.60113791807857098 ) ) ;
#12762=CARTESIAN_POINT ( 'NONE',  ( 9.680171189290716072, 214.0920067884432854, 21.69886208192144039 ) ) ;
#12763=CARTESIAN_POINT ( 'NONE',  ( -8.062137200540822946, 201.0835637161416400, 29.19886208192143684 ) ) ;
#12766=CARTESIAN_POINT ( 'NONE',  ( -12.01549611932652972, 203.1486557965464499, 63.35113791807857098 ) ) ;
#12767=CARTESIAN_POINT ( 'NONE',  ( 2.517493886308900919, 214.5937144450984420, 79.40113791807858945 ) ) ;
#12768=CARTESIAN_POINT ( 'NONE',  ( 0.05014649552828275708, 196.4853777576173002, 40.74886208192143044 ) ) ;
#12771=CARTESIAN_POINT ( 'NONE',  ( -3.753561863808878130, 218.3979405102790281, 42.09886208192143897 ) ) ;
#12778=CARTESIAN_POINT ( 'NONE',  ( 6.500168698208129925, 211.6636982574063381, 43.70113791807857240 ) ) ;
#12780=CARTESIAN_POINT ( 'NONE',  ( 8.118202686958138514, 201.1607312380088501, 22.29886208192143826 ) ) ;
#12783=CARTESIAN_POINT ( 'NONE',  ( 9.443650191645208025, 207.8375535574373032, -0.8718850525427659370 ) ) ;
#12786=CARTESIAN_POINT ( 'NONE',  ( -0.05014649552828403384, 217.5146222423826714, 102.2488620819214020 ) ) ;
#12787=CARTESIAN_POINT ( 'NONE',  ( 0.05014649552810505201, 217.5146222423826714, 37.25113791807855534 ) ) ;
#12789=CARTESIAN_POINT ( 'NONE',  ( -9.984503880673473830, 210.2968891136704315, 24.65113791807856103 ) ) ;
#12790=CARTESIAN_POINT ( 'NONE',  ( 3.044812012439969795, 216.5253028482143520, 102.3988620819214361 ) ) ;
#12791=CARTESIAN_POINT ( 'NONE',  ( 6.500168698208244500, 202.3363017425938324, 79.29886208192144181 ) ) ;
#12794=CARTESIAN_POINT ( 'NONE',  ( 9.680171189290831535, 199.9079932115568852, 8.301137918078564937 ) ) ;
#12797=CARTESIAN_POINT ( 'NONE',  ( 6.139770520408368348, 198.4640165459539674, 53.45113791807855108 ) ) ;
#12800=CARTESIAN_POINT ( 'NONE',  ( -10.00000000000000711, 206.9523078486584495, 2.498862081921433997 ) ) ;
#12803=CARTESIAN_POINT ( 'NONE',  ( 3.662846001190051659, 195.5725841191953691, 26.60113791807856742 ) ) ;
#12806=CARTESIAN_POINT ( 'NONE',  ( -8.118202686958138514, 212.8392687619910930, 8.798862081921434708 ) ) ;
#12809=CARTESIAN_POINT ( 'NONE',  ( -9.984503880673473830, 210.2968891136704315, 6.651137918078564581 ) ) ;
#12810=CARTESIAN_POINT ( 'NONE',  ( 6.220909254589536808, 215.4770327129947702, 67.55113791807853829 ) ) ;
#12812=CARTESIAN_POINT ( 'NONE',  ( -8.000000000000008882, 206.9523078486584780, 35.49886208192143044 ) ) ;
#12816=CARTESIAN_POINT ( 'NONE',  ( 2.517493886308900919, 214.5937144450984420, 10.40113791807856636 ) ) ;
#12817=CARTESIAN_POINT ( 'NONE',  ( 9.736236675708031640, 199.9851607334238963, 103.2988620819214560 ) ) ;
#12822=CARTESIAN_POINT ( 'NONE',  ( 3.044812012440130555, 197.4746971517856764, 8.601137918078565647 ) ) ;
#12824=CARTESIAN_POINT ( 'NONE',  ( -9.984503880673420539, 203.7031108863293980, 68.34886208192143897 ) ) ;
#12826=CARTESIAN_POINT ( 'NONE',  ( -0.3755270751584372513, 206.3579517667438665, 116.9470267523194593 ) ) ;
#12827=CARTESIAN_POINT ( 'NONE',  ( -10.01549611932653860, 203.7984951890123284, 12.35113791807856387 ) ) ;
#12830=CARTESIAN_POINT ( 'NONE',  ( 8.118202686958039038, 212.8392687619912635, 100.7011379180785866 ) ) ;
#12833=CARTESIAN_POINT ( 'NONE',  ( 8.062137200540920645, 201.0835637161417822, 71.30113791807856671 ) ) ;
#12836=CARTESIAN_POINT ( 'NONE',  ( -11.98450388067341876, 203.0532714938636047, 98.34886208192145318 ) ) ;
#12841=CARTESIAN_POINT ( 'NONE',  ( 3.662846001190051659, 195.5725841191953691, 98.60113791807857808 ) ) ;
#12845=CARTESIAN_POINT ( 'NONE',  ( 6.220909254589680693, 198.5229672870052582, 82.44886208192141908 ) ) ;
#12846=CARTESIAN_POINT ( 'NONE',  ( -7.375838497908014268, 196.7627149292498530, 20.04886208192143471 ) ) ;
#12849=CARTESIAN_POINT ( 'NONE',  ( 6.139770520408368348, 198.4640165459539674, 41.45113791807857240 ) ) ;
#12851=CARTESIAN_POINT ( 'NONE',  ( -8.000000000000008882, 206.9523078486584780, 2.498862081921435330 ) ) ;
#12856=CARTESIAN_POINT ( 'NONE',  ( 2.517493886309087436, 199.4062855549015865, 82.59886208192143897 ) ) ;
#12861=CARTESIAN_POINT ( 'NONE',  ( 4.984841277089725686, 213.7757310962907411, 58.55113791807858092 ) ) ;
#12865=CARTESIAN_POINT ( 'NONE',  ( -6.444103211791042618, 211.7408657792732356, 87.80113791807858092 ) ) ;
#12868=CARTESIAN_POINT ( 'NONE',  ( 6.500168698208244500, 202.3363017425938324, 67.29886208192144181 ) ) ;
#12873=CARTESIAN_POINT ( 'NONE',  ( 6.139770520408367460, 198.4640165459539389, -0.5488620819214342639 ) ) ;
#12877=CARTESIAN_POINT ( 'NONE',  ( -0.05014649552807705357, 194.3824533091408000, 65.75113791807856956 ) ) ;
#12879=CARTESIAN_POINT ( 'NONE',  ( 7.456977232089302632, 217.1783343296989131, 13.55113791807856849 ) ) ;
#12880=CARTESIAN_POINT ( 'NONE',  ( -10.01549611932653860, 203.7984951890123000, 90.35113791807857808 ) ) ;
#12882=CARTESIAN_POINT ( 'NONE',  ( -3.662846001189865142, 195.5725841191952838, 49.89886208192143613 ) ) ;
#12883=CARTESIAN_POINT ( 'NONE',  ( 3.135527875058981895, 197.5041725223112792, 58.59886208192143897 ) ) ;
#12885=CARTESIAN_POINT ( 'NONE',  ( -9.680171189290831535, 214.0920067884431148, 99.80113791807858092 ) ) ;
#12887=CARTESIAN_POINT ( 'NONE',  ( 9.984503880673470277, 203.7031108863295401, 14.15113791807856458 ) ) ;
#12888=CARTESIAN_POINT ( 'NONE',  ( -3.135527875058982783, 216.4958274776886924, 72.09886208192143897 ) ) ;
#12890=CARTESIAN_POINT ( 'NONE',  ( 12.01549611932659367, 203.1486557965466773, 82.14886208192143613 ) ) ;
#12891=CARTESIAN_POINT ( 'NONE',  ( -8.062137200540920645, 212.9164362838581894, 90.80113791807858092 ) ) ;
#12894=CARTESIAN_POINT ( 'NONE',  ( -7.984503880673422316, 204.3529502787951628, 50.34886208192144608 ) ) ;
#12904=CARTESIAN_POINT ( 'NONE',  ( -8.062137200540822946, 201.0835637161416400, 53.19886208192143329 ) ) ;
#12908=CARTESIAN_POINT ( 'NONE',  ( 2.517493886309087436, 199.4062855549015865, 34.59886208192143897 ) ) ;
#12910=CARTESIAN_POINT ( 'NONE',  ( 8.062137200540920645, 201.0835637161417822, 74.30113791807858092 ) ) ;
#12912=CARTESIAN_POINT ( 'NONE',  ( 9.984503880673470277, 203.7031108863295401, 53.15113791807857524 ) ) ;
#12914=CARTESIAN_POINT ( 'NONE',  ( -6.139770520408369237, 215.5359834540460042, 27.95113791807856174 ) ) ;
#12915=CARTESIAN_POINT ( 'NONE',  ( -2.517493886308901807, 199.4062855549015012, 11.90113791807856813 ) ) ;
#12919=CARTESIAN_POINT ( 'NONE',  ( 7.456977232089302632, 217.1783343296989131, 40.55113791807856671 ) ) ;
#12921=CARTESIAN_POINT ( 'NONE',  ( -6.220909254589537696, 198.5229672870051161, 81.05113791807856671 ) ) ;
#12922=CARTESIAN_POINT ( 'NONE',  ( 6.139770520408367460, 198.4640165459539389, 56.45113791807857950 ) ) ;
#12925=CARTESIAN_POINT ( 'NONE',  ( -7.456977232089471386, 217.1783343296987709, 20.94886208192143684 ) ) ;
#12926=CIRCLE ( 'NONE', #13930, 8.624472924841564136 ) ;
#12927=CARTESIAN_POINT ( 'NONE',  ( -10.01549611932659545, 210.2015048109875011, 32.64886208192143613 ) ) ;
#12929=CARTESIAN_POINT ( 'NONE',  ( 3.662846001190051659, 195.5725841191953691, 68.60113791807857808 ) ) ;
#12930=CARTESIAN_POINT ( 'NONE',  ( -8.000000000000008882, 207.0476921513413515, 81.50113791807856956 ) ) ;
#12931=CARTESIAN_POINT ( 'NONE',  ( -8.118202686958138514, 212.8392687619910930, 38.79886208192143471 ) ) ;
#12935=CARTESIAN_POINT ( 'NONE',  ( 9.680171189290716072, 214.0920067884432854, 54.69886208192144039 ) ) ;
#12943=CARTESIAN_POINT ( 'NONE',  ( -2.517493886308901807, 199.4062855549015012, 38.90113791807856813 ) ) ;
#12944=CIRCLE ( 'NONE', #25439, 1.000000000000000888 ) ;
#12949=CARTESIAN_POINT ( 'NONE',  ( 10.00000000000000711, 207.0476921513415220, 24.99886208192143400 ) ) ;
#12956=CARTESIAN_POINT ( 'NONE',  ( -6.500168698208244500, 211.6636982574061676, 2.798862081921434708 ) ) ;
#12957=CARTESIAN_POINT ( 'NONE',  ( 3.135527875058820690, 216.4958274776887492, 46.40113791807857524 ) ) ;
#12958=CARTESIAN_POINT ( 'NONE',  ( -3.135527875058821579, 197.5041725223112223, 29.90113791807856813 ) ) ;
#12962=CARTESIAN_POINT ( 'NONE',  ( 2.426778023690075337, 214.6231898156240447, 96.39886208192146455 ) ) ;
#12965=CARTESIAN_POINT ( 'NONE',  ( 12.00000000000000711, 206.9523078486586485, 11.00113791807856600 ) ) ;
#12969=CARTESIAN_POINT ( 'NONE',  ( 10.00000000000000711, 206.9523078486586201, 59.00113791807857666 ) ) ;
#12976=CARTESIAN_POINT ( 'NONE',  ( -3.662846001190052991, 218.4274158808045740, 40.10113791807856387 ) ) ;
#12979=CARTESIAN_POINT ( 'NONE',  ( 3.135527875058981895, 197.5041725223112792, 13.59886208192143719 ) ) ;
#12981=CARTESIAN_POINT ( 'NONE',  ( 10.00000000000000888, 207.8294911128234617, -1.040744497668167012 ) ) ;
#12983=CARTESIAN_POINT ( 'NONE',  ( -3.044812012440131443, 216.5253028482142952, 7.101137918078566535 ) ) ;
#12984=CARTESIAN_POINT ( 'NONE',  ( -6.220909254589537696, 198.5229672870051161, 69.05113791807858092 ) ) ;
#12985=ORIENTED_EDGE ( 'NONE', *, *, #30843, .T. ) ;
#12986=CARTESIAN_POINT ( 'NONE',  ( 8.015496119326595448, 204.4483345814782638, 34.14886208192144323 ) ) ;
#12990=CARTESIAN_POINT ( 'NONE',  ( -4.984841277089726574, 200.2242689037092305, 12.05113791807856849 ) ) ;
#12991=CARTESIAN_POINT ( 'NONE',  ( -11.98450388067341876, 203.0532714938636047, 95.34886208192143897 ) ) ;
#12996=CARTESIAN_POINT ( 'NONE',  ( 10.01549611932653860, 210.2015048109876716, 7.851137918078566535 ) ) ;
#12997=CARTESIAN_POINT ( 'NONE',  ( 3.135527875058981895, 197.5041725223112792, 85.59886208192143897 ) ) ;
#13000=CARTESIAN_POINT ( 'NONE',  ( 0.05014649552810505201, 217.5146222423826714, 16.25113791807856600 ) ) ;
#13005=CARTESIAN_POINT ( 'NONE',  ( 0.05014649552810505201, 217.5146222423826714, 97.25113791807854113 ) ) ;
#13007=CARTESIAN_POINT ( 'NONE',  ( 3.135527875058820690, 216.4958274776887492, 85.40113791807857524 ) ) ;
#13010=CARTESIAN_POINT ( 'NONE',  ( -12.00000000000000711, 206.9523078486584780, 95.49886208192144466 ) ) ;
#13016=CARTESIAN_POINT ( 'NONE',  ( 0.05014649552807549926, 219.6175466908591716, 94.25113791807859798 ) ) ;
#13019=CARTESIAN_POINT ( 'NONE',  ( 9.984503880673420539, 210.2968891136705736, 84.84886208192143897 ) ) ;
#13020=CARTESIAN_POINT ( 'NONE',  ( 12.00000000000000711, 207.0476921513415220, 21.99886208192143400 ) ) ;
#13021=CARTESIAN_POINT ( 'NONE',  ( 10.20891672561132424, 208.8253170565643302, -1.573594014082846382 ) ) ;
#13023=CARTESIAN_POINT ( 'NONE',  ( 9.984503880673470277, 203.7031108863295401, 38.15113791807856813 ) ) ;
#13025=CARTESIAN_POINT ( 'NONE',  ( 6.500168698208244500, 202.3363017425938324, 4.298862081921435596 ) ) ;
#13028=CARTESIAN_POINT ( 'NONE',  ( 8.015496119326595448, 204.4483345814782638, 91.14886208192143613 ) ) ;
#13030=CARTESIAN_POINT ( 'NONE',  ( 7.984503880673485376, 204.3529502787953902, 35.15113791807856103 ) ) ;
#13036=CARTESIAN_POINT ( 'NONE',  ( -4.984841277089726574, 200.2242689037092305, 87.05113791807856671 ) ) ;
#13041=CARTESIAN_POINT ( 'NONE',  ( 4.984841277089891776, 200.2242689037093726, 64.44886208192143329 ) ) ;
#13049=CARTESIAN_POINT ( 'NONE',  ( 3.662846001190051659, 195.5725841191953691, 71.60113791807857808 ) ) ;
#13051=CARTESIAN_POINT ( 'NONE',  ( 12.01549611932652972, 210.8513442034534933, 13.85113791807856742 ) ) ;
#13052=CARTESIAN_POINT ( 'NONE',  ( -8.062137200540920645, 212.9164362838581894, 84.80113791807856671 ) ) ;
#13054=CARTESIAN_POINT ( 'NONE',  ( -3.753561863808878130, 218.3979405102790281, 51.09886208192143897 ) ) ;
#13055=CARTESIAN_POINT ( 'NONE',  ( -10.01549611932659545, 210.2015048109875011, 59.64886208192143613 ) ) ;
#13056=CARTESIAN_POINT ( 'NONE',  ( 9.736236675707914401, 214.0148392665762458, 100.7011379180785866 ) ) ;
#13058=CARTESIAN_POINT ( 'NONE',  ( -6.139770520408369237, 215.5359834540460042, 12.95113791807856352 ) ) ;
#13059=CARTESIAN_POINT ( 'NONE',  ( -0.05014649552828403384, 217.5146222423826714, 75.24886208192144466 ) ) ;
#13061=CARTESIAN_POINT ( 'NONE',  ( -11.98450388067341876, 203.0532714938636047, 80.34886208192143897 ) ) ;
#13062=CARTESIAN_POINT ( 'NONE',  ( 3.044812012440130555, 197.4746971517856764, 95.60113791807857808 ) ) ;
#13065=CARTESIAN_POINT ( 'NONE',  ( -2.426778023690076225, 199.3768101843759553, 64.89886208192143613 ) ) ;
#13074=CARTESIAN_POINT ( 'NONE',  ( -10.00000000000000711, 206.9523078486584495, 50.49886208192143044 ) ) ;
#13079=CARTESIAN_POINT ( 'NONE',  ( -6.444103211790928043, 202.2591342207265939, 32.19886208192144039 ) ) ;
#13080=CARTESIAN_POINT ( 'NONE',  ( -10.01549611932653860, 203.7984951890123284, 75.35113791807853545 ) ) ;
#13082=CARTESIAN_POINT ( 'NONE',  ( 8.062137200540920645, 201.0835637161417822, 53.30113791807857382 ) ) ;
#13084=CARTESIAN_POINT ( 'NONE',  ( 6.139770520408368348, 198.4640165459539674, 32.45113791807856529 ) ) ;
#13085=CARTESIAN_POINT ( 'NONE',  ( -2.517493886308901807, 199.4062855549015012, 17.90113791807856458 ) ) ;
#13089=CARTESIAN_POINT ( 'NONE',  ( 0.05014649552807549926, 219.6175466908591716, 40.25113791807856245 ) ) ;
#13091=CARTESIAN_POINT ( 'NONE',  ( 8.062137200540920645, 201.0835637161417822, 83.30113791807858092 ) ) ;
#13092=CARTESIAN_POINT ( 'NONE',  ( -8.062137200540920645, 212.9164362838581894, 54.80113791807857382 ) ) ;
#13093=CARTESIAN_POINT ( 'NONE',  ( 3.662846001189864698, 218.4274158808046593, 21.39886208192143613 ) ) ;
#13094=CARTESIAN_POINT ( 'NONE',  ( -3.044812012439970683, 197.4746971517856196, 25.89886208192143613 ) ) ;
#13096=CARTESIAN_POINT ( 'NONE',  ( -12.00000000000000711, 207.0476921513413515, 69.50113791807856956 ) ) ;
#13097=CARTESIAN_POINT ( 'NONE',  ( -8.015496119326531499, 204.4483345814780364, 87.35113791807857808 ) ) ;
#13099=CARTESIAN_POINT ( 'NONE',  ( 8.062137200540822946, 212.9164362838583315, 48.69886208192144039 ) ) ;
#13102=CARTESIAN_POINT ( 'NONE',  ( 11.98450388067341876, 210.9467285061363953, 51.84886208192144608 ) ) ;
#13109=CARTESIAN_POINT ( 'NONE',  ( 0.05014649552807626948, 215.4116977939061144, 46.25113791807857666 ) ) ;
#13111=CARTESIAN_POINT ( 'NONE',  ( 8.062137200540822946, 212.9164362838583315, 21.69886208192143684 ) ) ;
#13117=CARTESIAN_POINT ( 'NONE',  ( -8.015496119326597224, 209.5516654185217362, 8.648862081921436129 ) ) ;
#13118=CARTESIAN_POINT ( 'NONE',  ( 8.118202686958039038, 212.8392687619912635, 40.70113791807857240 ) ) ;
#13119=CARTESIAN_POINT ( 'NONE',  ( -10.00000000000000711, 207.0476921513413515, 27.50113791807856600 ) ) ;
#13120=CARTESIAN_POINT ( 'NONE',  ( -3.044812012439970683, 197.4746971517856196, 103.8988620819214361 ) ) ;
#13123=CARTESIAN_POINT ( 'NONE',  ( 2.517493886309087436, 199.4062855549015865, 91.59886208192145318 ) ) ;
#13127=CARTESIAN_POINT ( 'NONE',  ( 7.456977232089302632, 217.1783343296989131, 10.55113791807856671 ) ) ;
#13131=CARTESIAN_POINT ( 'NONE',  ( -6.139770520408369237, 215.5359834540460042, 54.95113791807856529 ) ) ;
#13138=CARTESIAN_POINT ( 'NONE',  ( -7.456977232089304408, 196.8216656703010301, 36.05113791807855961 ) ) ;
#13141=CARTESIAN_POINT ( 'NONE',  ( 10.01549611932659545, 203.7984951890123853, 10.14886208192143613 ) ) ;
#13145=CARTESIAN_POINT ( 'NONE',  ( -3.044812012440131443, 216.5253028482142952, 73.10113791807857808 ) ) ;
#13148=CARTESIAN_POINT ( 'NONE',  ( 6.500168698208244500, 202.3363017425938324, 37.29886208192144181 ) ) ;
#13152=CARTESIAN_POINT ( 'NONE',  ( 8.000000000000008882, 206.9523078486586485, 14.00113791807856600 ) ) ;
#13153=CARTESIAN_POINT ( 'NONE',  ( 12.00000000000000711, 207.0476921513415220, 102.9988620819214304 ) ) ;
#13158=CARTESIAN_POINT ( 'NONE',  ( -10.01549611932653860, 203.7984951890123284, 12.35113791807856387 ) ) ;
#13160=CARTESIAN_POINT ( 'NONE',  ( 10.00000000000000711, 207.0476921513415220, 78.99886208192144466 ) ) ;
#13163=CARTESIAN_POINT ( 'NONE',  ( -9.984503880673473830, 210.2968891136704315, 15.65113791807856813 ) ) ;
#13168=CARTESIAN_POINT ( 'NONE',  ( 6.139770520408368348, 198.4640165459539674, 83.45113791807858661 ) ) ;
#13171=CARTESIAN_POINT ( 'NONE',  ( 0.05014649552828288198, 194.3824533091408000, 94.74886208192144466 ) ) ;
#13173=ORIENTED_EDGE ( 'NONE', *, *, #18151, .T. ) ;
#13177=CARTESIAN_POINT ( 'NONE',  ( 12.01549611932652972, 210.8513442034534933, 94.85113791807856387 ) ) ;
#13180=CARTESIAN_POINT ( 'NONE',  ( 6.139770520408223575, 215.5359834540460611, 93.54886208192142760 ) ) ;
#13182=CARTESIAN_POINT ( 'NONE',  ( 7.456977232089471386, 196.8216656703012006, 25.44886208192143684 ) ) ;
#13184=CARTESIAN_POINT ( 'NONE',  ( 6.220909254589536808, 215.4770327129947702, 46.55113791807856671 ) ) ;
#13186=CARTESIAN_POINT ( 'NONE',  ( -7.984503880673422316, 204.3529502787951628, 8.348862081921435419 ) ) ;
#13189=CARTESIAN_POINT ( 'NONE',  ( -2.517493886309087880, 214.5937144450984135, 93.09886208192145318 ) ) ;
#13190=CARTESIAN_POINT ( 'NONE',  ( -2.517493886308901807, 199.4062855549015012, 29.90113791807857169 ) ) ;
#13196=CARTESIAN_POINT ( 'NONE',  ( -5.935092644091702674, 206.1175677538518585, -6.000000000000015987 ) ) ;
#13197=CARTESIAN_POINT ( 'NONE',  ( 8.000000000000008882, 206.9523078486586485, 92.00113791807858377 ) ) ;
#13201=CARTESIAN_POINT ( 'NONE',  ( 4.903702542908435547, 213.8346818373419751, 63.54886208192144181 ) ) ;
#13205=CARTESIAN_POINT ( 'NONE',  ( -0.05014649552810635652, 196.4853777576173002, 5.751137918078565114 ) ) ;
#13209=CARTESIAN_POINT ( 'NONE',  ( 7.375838497908181246, 196.7627149292499666, 65.45113791807858661 ) ) ;
#13211=CARTESIAN_POINT ( 'NONE',  ( -0.05014649552810635652, 196.4853777576173002, 86.75113791807858377 ) ) ;
#13213=CARTESIAN_POINT ( 'NONE',  ( -11.98450388067341876, 203.0532714938636047, 50.34886208192144608 ) ) ;
#13215=CARTESIAN_POINT ( 'NONE',  ( 9.984503880673420539, 210.2968891136705736, 54.84886208192142476 ) ) ;
#13216=CARTESIAN_POINT ( 'NONE',  ( -12.00000000000000711, 207.0476921513413515, 93.50113791807858377 ) ) ;
#13218=CARTESIAN_POINT ( 'NONE',  ( -0.05014649552810635652, 196.4853777576173002, 8.751137918078562450 ) ) ;
#13219=CARTESIAN_POINT ( 'NONE',  ( -9.984503880673420539, 203.7031108863293980, 77.34886208192142476 ) ) ;
#13222=CARTESIAN_POINT ( 'NONE',  ( -3.135527875058821579, 197.5041725223112223, 98.90113791807857524 ) ) ;
#13226=CARTESIAN_POINT ( 'NONE',  ( 8.015496119326595448, 204.4483345814782638, 61.14886208192145034 ) ) ;
#13234=CARTESIAN_POINT ( 'NONE',  ( -4.984841277089726574, 200.2242689037092305, 60.05113791807858092 ) ) ;
#13236=CARTESIAN_POINT ( 'NONE',  ( 6.139770520408223575, 215.5359834540460611, 48.54886208192143471 ) ) ;
#13237=CARTESIAN_POINT ( 'NONE',  ( -10.00000000000000888, 210.1396626997885448, 100.6464902082600474 ) ) ;
#13240=CARTESIAN_POINT ( 'NONE',  ( -7.984503880673422316, 204.3529502787951628, 38.34886208192142476 ) ) ;
#13241=CARTESIAN_POINT ( 'NONE',  ( -10.00000000000000711, 207.0476921513413515, 78.50113791807856956 ) ) ;
#13243=CARTESIAN_POINT ( 'NONE',  ( -0.05014649552810635652, 196.4853777576173002, 53.75113791807857666 ) ) ;
#13244=CARTESIAN_POINT ( 'NONE',  ( -10.00000000000000711, 207.0476921513413515, 27.50113791807856600 ) ) ;
#13245=CARTESIAN_POINT ( 'NONE',  ( 4.903702542908601636, 200.1653181626581102, 11.45113791807856529 ) ) ;
#13250=CARTESIAN_POINT ( 'NONE',  ( 12.00000000000000711, 206.9523078486586485, 41.00113791807856245 ) ) ;
#13253=CARTESIAN_POINT ( 'NONE',  ( -3.135527875058821579, 197.5041725223112223, 89.90113791807857524 ) ) ;
#13254=CARTESIAN_POINT ( 'NONE',  ( 8.062137200540920645, 201.0835637161417822, 59.30113791807857382 ) ) ;
#13255=CARTESIAN_POINT ( 'NONE',  ( 0.05014649552828288198, 194.3824533091408000, 25.74886208192143755 ) ) ;
#13256=CARTESIAN_POINT ( 'NONE',  ( 10.00000000000000711, 207.0476921513415220, 30.99886208192143755 ) ) ;
#13258=CARTESIAN_POINT ( 'NONE',  ( -7.375838497908182134, 217.2372850707499765, 69.95113791807858661 ) ) ;
#13259=CARTESIAN_POINT ( 'NONE',  ( 2.517493886308900919, 214.5937144450984420, 91.40113791807857524 ) ) ;
#13260=CARTESIAN_POINT ( 'NONE',  ( -10.00000000000000711, 206.9523078486584495, 53.49886208192143755 ) ) ;
#13264=CARTESIAN_POINT ( 'NONE',  ( -12.00000000000000711, 206.9523078486584780, 47.49886208192144466 ) ) ;
#13272=CARTESIAN_POINT ( 'NONE',  ( -7.984503880673488041, 209.6470497212046098, 45.65113791807857524 ) ) ;
#13274=CARTESIAN_POINT ( 'NONE',  ( 10.01549611932659545, 203.7984951890123853, 28.14886208192143613 ) ) ;
#13280=CARTESIAN_POINT ( 'NONE',  ( 0.05014649552828262524, 198.5883022060938572, 1.748862081921434886 ) ) ;
#13281=CARTESIAN_POINT ( 'NONE',  ( 9.984503880673470277, 203.7031108863295401, 50.15113791807855392 ) ) ;
#13285=CARTESIAN_POINT ( 'NONE',  ( 8.062137200540920645, 201.0835637161417822, 32.30113791807857382 ) ) ;
#13288=CARTESIAN_POINT ( 'NONE',  ( -6.444103211790928043, 202.2591342207265939, 95.19886208192144750 ) ) ;
#13291=CARTESIAN_POINT ( 'NONE',  ( 7.456977232089302632, 217.1783343296989131, 13.55113791807856849 ) ) ;
#13295=CARTESIAN_POINT ( 'NONE',  ( 8.062137200540920645, 201.0835637161417822, 59.30113791807857382 ) ) ;
#13296=CARTESIAN_POINT ( 'NONE',  ( -8.062137200540920645, 212.9164362838581894, 27.80113791807856671 ) ) ;
#13298=CARTESIAN_POINT ( 'NONE',  ( -6.139770520408224463, 198.4640165459539105, 2.048862081921434264 ) ) ;
#13301=VERTEX_POINT ( 'NONE', #20591 ) ;
#13302=CARTESIAN_POINT ( 'NONE',  ( 3.753561863808689836, 218.3979405102790565, 43.40113791807856813 ) ) ;
#13304=CARTESIAN_POINT ( 'NONE',  ( -6.139770520408224463, 198.4640165459539389, 17.04886208192143826 ) ) ;
#13308=CARTESIAN_POINT ( 'NONE',  ( -10.01549611932653860, 203.7984951890123284, 75.35113791807853545 ) ) ;
#13313=CARTESIAN_POINT ( 'NONE',  ( -0.05014649552807731031, 198.5883022060938572, 17.75113791807856956 ) ) ;
#13316=CARTESIAN_POINT ( 'NONE',  ( 7.456977232089471386, 196.8216656703012006, 100.4488620819214475 ) ) ;
#13322=CARTESIAN_POINT ( 'NONE',  ( 8.062137200540920645, 201.0835637161417822, 5.301137918078566713 ) ) ;
#13323=CARTESIAN_POINT ( 'NONE',  ( -3.044812012439970683, 197.4746971517856196, 76.89886208192143613 ) ) ;
#13326=CARTESIAN_POINT ( 'NONE',  ( -8.118202686958039038, 201.1607312380087080, 9.201137918078565292 ) ) ;
#13330=CARTESIAN_POINT ( 'NONE',  ( -3.135527875058821579, 197.5041725223112223, 95.90113791807858945 ) ) ;
#13332=CARTESIAN_POINT ( 'NONE',  ( -6.139770520408369237, 215.5359834540460042, 81.95113791807854398 ) ) ;
#13335=CARTESIAN_POINT ( 'NONE',  ( 12.00000000000000711, 207.0476921513415220, 93.99886208192144466 ) ) ;
#13343=CARTESIAN_POINT ( 'NONE',  ( -8.062137200540822946, 201.0835637161416400, 98.19886208192143329 ) ) ;
#13344=CARTESIAN_POINT ( 'NONE',  ( 3.753561863808876797, 195.6020594897209719, 34.59886208192143187 ) ) ;
#13346=CARTESIAN_POINT ( 'NONE',  ( -10.01549611932653860, 203.7984951890123284, 39.35113791807857098 ) ) ;
#13348=CARTESIAN_POINT ( 'NONE',  ( -8.062137200540822946, 201.0835637161416400, 104.1988620819214475 ) ) ;
#13351=CARTESIAN_POINT ( 'NONE',  ( 8.000000000000008882, 207.0476921513415220, 90.99886208192144466 ) ) ;
#13354=CARTESIAN_POINT ( 'NONE',  ( 4.984841277089725686, 213.7757310962907411, 31.55113791807857382 ) ) ;
#13360=CARTESIAN_POINT ( 'NONE',  ( -8.000000000000008882, 207.0476921513413515, 84.50113791807856956 ) ) ;
#13363=CARTESIAN_POINT ( 'NONE',  ( 8.015496119326595448, 204.4483345814782638, 67.14886208192143613 ) ) ;
#13366=CARTESIAN_POINT ( 'NONE',  ( -10.01549611932653860, 203.7984951890123000, 15.35113791807856565 ) ) ;
#13370=CARTESIAN_POINT ( 'NONE',  ( -9.680171189290831535, 214.0920067884431148, 78.80113791807858092 ) ) ;
#13372=CARTESIAN_POINT ( 'NONE',  ( 3.044812012440130555, 197.4746971517856764, 89.60113791807857808 ) ) ;
#13375=CARTESIAN_POINT ( 'NONE',  ( 12.01549611932659367, 203.1486557965466773, 52.14886208192143613 ) ) ;
#13376=CARTESIAN_POINT ( 'NONE',  ( 3.044812012439969795, 216.5253028482143520, 69.39886208192143613 ) ) ;
#13377=CARTESIAN_POINT ( 'NONE',  ( 7.375838497908181246, 196.7627149292499666, 95.45113791807858661 ) ) ;
#13380=CARTESIAN_POINT ( 'NONE',  ( 8.062137200540920645, 201.0835637161417822, 17.30113791807856671 ) ) ;
#13381=CARTESIAN_POINT ( 'NONE',  ( -3.135527875058982783, 216.4958274776886924, 78.09886208192143897 ) ) ;
#13383=CARTESIAN_POINT ( 'NONE',  ( -0.05014649552810635652, 196.4853777576173002, 101.7511379180785411 ) ) ;
#13386=CARTESIAN_POINT ( 'NONE',  ( 4.984841277089891776, 200.2242689037093726, 61.44886208192144039 ) ) ;
#13389=DIRECTION ( 'NONE',  ( 0.000000000000000000, -0.04769215134144196705, 0.9988620819214357738 ) ) ;
#13393=CARTESIAN_POINT ( 'NONE',  ( -6.444103211791042618, 211.7408657792732356, 57.80113791807857382 ) ) ;
#13394=CYLINDRICAL_SURFACE ( 'NONE', #31972, 1.000000000000000000 ) ;
#13396=CARTESIAN_POINT ( 'NONE',  ( -9.395856286962974480, 206.1620322824069831, 104.2858818099143008 ) ) ;
#13400=CARTESIAN_POINT ( 'NONE',  ( -8.000000000000008882, 206.9523078486584780, 38.49886208192143044 ) ) ;
#13401=CARTESIAN_POINT ( 'NONE',  ( 10.01549611932653860, 210.2015048109876716, 79.85113791807853545 ) ) ;
#13404=CARTESIAN_POINT ( 'NONE',  ( -8.062137200540920645, 212.9164362838581894, 66.80113791807858092 ) ) ;
#13407=CARTESIAN_POINT ( 'NONE',  ( -4.984841277089726574, 200.2242689037092305, 18.05113791807856316 ) ) ;
#13411=CARTESIAN_POINT ( 'NONE',  ( -9.736236675707914401, 199.9851607334237542, 42.20113791807857240 ) ) ;
#13413=CARTESIAN_POINT ( 'NONE',  ( -6.139770520408369237, 215.5359834540460042, 93.95113791807854398 ) ) ;
#13414=CARTESIAN_POINT ( 'NONE',  ( 8.118202686958039038, 212.8392687619912635, 61.70113791807857240 ) ) ;
#13415=CARTESIAN_POINT ( 'NONE',  ( 0.05014649552828288198, 194.3824533091408000, 22.74886208192143755 ) ) ;
#13416=CARTESIAN_POINT ( 'NONE',  ( -8.118202686958138514, 212.8392687619910930, 35.79886208192143471 ) ) ;
#13418=CARTESIAN_POINT ( 'NONE',  ( -12.01549611932652972, 203.1486557965464499, 69.35113791807857808 ) ) ;
#13419=CARTESIAN_POINT ( 'NONE',  ( -4.903702542908602524, 213.8346818373418898, 87.95113791807857240 ) ) ;
#13420=CARTESIAN_POINT ( 'NONE',  ( 10.01549611932659545, 203.7984951890123853, 55.14886208192143613 ) ) ;
#13423=CARTESIAN_POINT ( 'NONE',  ( 3.753561863808876797, 195.6020594897209719, 52.59886208192143897 ) ) ;
#13431=CARTESIAN_POINT ( 'NONE',  ( 6.444103211791042618, 202.2591342207267644, 38.30113791807856671 ) ) ;
#13432=CARTESIAN_POINT ( 'NONE',  ( -6.220909254589682469, 215.4770327129946850, 26.94886208192142618 ) ) ;
#13436=UNCERTAINTY_MEASURE_WITH_UNIT (LENGTH_MEASURE( 1.000000000000000082E-05 ), #19726, 'distance_accuracy_value', 'NONE');
#13439=CARTESIAN_POINT ( 'NONE',  ( -2.517493886309087880, 214.5937144450984135, 6.098862081921434530 ) ) ;
#13441=CARTESIAN_POINT ( 'NONE',  ( 8.118202686958039038, 212.8392687619912635, 55.70113791807857950 ) ) ;
#13443=EDGE_CURVE ( 'NONE', #13301, #4391, #26354, .T. ) ;
#13444=CARTESIAN_POINT ( 'NONE',  ( 8.118202686958039038, 212.8392687619912635, 25.70113791807856529 ) ) ;
#13448=CARTESIAN_POINT ( 'NONE',  ( 4.903702542908435547, 213.8346818373419751, 87.54886208192142760 ) ) ;
#13451=DIRECTION ( 'NONE',  ( 0.000000000000000000, -0.04769215134145524809, -0.9988620819214351076 ) ) ;
#13452=CARTESIAN_POINT ( 'NONE',  ( -11.98450388067348804, 210.9467285061362247, 6.651137918078566358 ) ) ;
#13455=CARTESIAN_POINT ( 'NONE',  ( -8.062137200540920645, 212.9164362838581894, 54.80113791807857382 ) ) ;
#13456=CARTESIAN_POINT ( 'NONE',  ( -3.135527875058821579, 197.5041725223112223, 26.90113791807856813 ) ) ;
#13461=CARTESIAN_POINT ( 'NONE',  ( -9.984503880673420539, 203.7031108863293980, 2.348862081921433642 ) ) ;
#13464=CARTESIAN_POINT ( 'NONE',  ( 11.98450388067348271, 203.0532714938637753, 38.15113791807856813 ) ) ;
#13466=CARTESIAN_POINT ( 'NONE',  ( 10.01549611932659545, 203.7984951890123853, 25.14886208192143613 ) ) ;
#13470=CARTESIAN_POINT ( 'NONE',  ( -10.00000000000000711, 207.0476921513413515, 81.50113791807856956 ) ) ;
#13476=CARTESIAN_POINT ( 'NONE',  ( -7.984503880673488041, 209.6470497212046098, 12.65113791807856636 ) ) ;
#13479=CARTESIAN_POINT ( 'NONE',  ( -7.456977232089471386, 217.1783343296987709, 95.94886208192144750 ) ) ;
#13486=CARTESIAN_POINT ( 'NONE',  ( 10.00000000000000711, 207.0476921513415220, 84.99886208192143044 ) ) ;
#13488=CARTESIAN_POINT ( 'NONE',  ( -10.00000000000000711, 207.0476921513413515, 21.50113791807856956 ) ) ;
#13494=CARTESIAN_POINT ( 'NONE',  ( -0.05014649552810635652, 196.4853777576173002, 80.75113791807854113 ) ) ;
#13495=CIRCLE ( 'NONE', #11310, 0.9999999999999947820 ) ;
#13498=CARTESIAN_POINT ( 'NONE',  ( 7.456977232089471386, 196.8216656703012006, 94.44886208192143329 ) ) ;
#13509=CARTESIAN_POINT ( 'NONE',  ( 10.01549611932659367, 203.7984951890124421, 94.14886208192143613 ) ) ;
#13510=CARTESIAN_POINT ( 'NONE',  ( 0.05014649552828288198, 194.3824533091408000, 34.74886208192142334 ) ) ;
#13512=CARTESIAN_POINT ( 'NONE',  ( 8.062137200540920645, 201.0835637161417822, 41.30113791807857382 ) ) ;
#13515=CARTESIAN_POINT ( 'NONE',  ( 4.903702542908435547, 213.8346818373419751, 3.548862081921434264 ) ) ;
#13518=CARTESIAN_POINT ( 'NONE',  ( 6.500168698208244500, 202.3363017425938324, 88.29886208192142760 ) ) ;
#13521=CARTESIAN_POINT ( 'NONE',  ( -0.05014649552807731031, 198.5883022060938572, 32.75113791807856956 ) ) ;
#13528=CARTESIAN_POINT ( 'NONE',  ( 4.903702542908601636, 200.1653181626581102, 101.4511379180785866 ) ) ;
#13532=CARTESIAN_POINT ( 'NONE',  ( -6.500168698208244500, 211.6636982574061676, 68.79886208192144181 ) ) ;
#13535=CARTESIAN_POINT ( 'NONE',  ( 6.220909254589536808, 215.4770327129947987, 7.551137918078564937 ) ) ;
#13540=CARTESIAN_POINT ( 'NONE',  ( -9.736236675707914401, 199.9851607334237542, 78.20113791807857240 ) ) ;
#13544=CARTESIAN_POINT ( 'NONE',  ( -6.220909254589537696, 198.5229672870051445, 93.05113791807856671 ) ) ;
#13547=CARTESIAN_POINT ( 'NONE',  ( 7.456977232089471386, 196.8216656703012006, 58.44886208192144039 ) ) ;
#13548=CARTESIAN_POINT ( 'NONE',  ( -10.00000000000000711, 207.0476921513413515, 54.50113791807857666 ) ) ;
#13549=CARTESIAN_POINT ( 'NONE',  ( -3.044812012439970683, 197.4746971517856196, 70.89886208192143613 ) ) ;
#13550=CARTESIAN_POINT ( 'NONE',  ( -9.680171189290716072, 199.9079932115567146, 8.198862081921433287 ) ) ;
#13552=CARTESIAN_POINT ( 'NONE',  ( -6.139770520408369237, 215.5359834540460042, 9.951137918078567068 ) ) ;
#13555=CARTESIAN_POINT ( 'NONE',  ( -8.062137200540822946, 201.0835637161416400, 83.19886208192143329 ) ) ;
#13557=AXIS2_PLACEMENT_3D ( 'NONE', #4138, #32418, #22035 ) ;
#13559=CARTESIAN_POINT ( 'NONE',  ( 6.139770520408368348, 198.4640165459539674, 98.45113791807854398 ) ) ;
#13562=CARTESIAN_POINT ( 'NONE',  ( -6.444103211790928043, 202.2591342207265939, 59.19886208192144750 ) ) ;
#13569=CARTESIAN_POINT ( 'NONE',  ( -6.500168698208129925, 202.3363017425936050, 57.20113791807857240 ) ) ;
#13573=CARTESIAN_POINT ( 'NONE',  ( 0.05014649552828262524, 198.5883022060938572, 43.74886208192144466 ) ) ;
#13574=CARTESIAN_POINT ( 'NONE',  ( -8.118202686958039038, 201.1607312380087080, 81.20113791807857240 ) ) ;
#13576=CARTESIAN_POINT ( 'NONE',  ( 6.220909254589536808, 215.4770327129947702, 61.55113791807858092 ) ) ;
#13577=DIRECTION ( 'NONE',  ( -0.3500148194780949296, -0.04467534437043436252, 0.9356782244720135422 ) ) ;
#13578=CARTESIAN_POINT ( 'NONE',  ( 6.500168698208129925, 211.6636982574063381, 19.70113791807856884 ) ) ;
#13582=CARTESIAN_POINT ( 'NONE',  ( -3.753561863808691168, 195.6020594897209435, 44.90113791807856813 ) ) ;
#13584=CARTESIAN_POINT ( 'NONE',  ( -3.135527875058821579, 197.5041725223112223, 92.90113791807857524 ) ) ;
#13585=CARTESIAN_POINT ( 'NONE',  ( 0.05014649552810506589, 217.5146222423826714, 64.25113791807856956 ) ) ;
#13586=CARTESIAN_POINT ( 'NONE',  ( 12.00000000000000711, 207.0476921513415220, 30.99886208192143400 ) ) ;
#13587=CARTESIAN_POINT ( 'NONE',  ( 8.118202686958138514, 201.1607312380088501, 34.29886208192143471 ) ) ;
#13589=CARTESIAN_POINT ( 'NONE',  ( -11.98450388067348804, 210.9467285061362247, 72.65113791807856103 ) ) ;
#13590=CARTESIAN_POINT ( 'NONE',  ( 6.500168698208129925, 211.6636982574063381, 85.70113791807858661 ) ) ;
#13591=CARTESIAN_POINT ( 'NONE',  ( 3.044812012439969795, 216.5253028482143520, 48.39886208192143613 ) ) ;
#13594=CARTESIAN_POINT ( 'NONE',  ( 11.98450388067341876, 210.9467285061363953, 48.84886208192143897 ) ) ;
#13596=ORIENTED_EDGE ( 'NONE', *, *, #4778, .T. ) ;
#13600=CARTESIAN_POINT ( 'NONE',  ( -8.000000000000008882, 207.0476921513413515, 48.50113791807856956 ) ) ;
#13601=CARTESIAN_POINT ( 'NONE',  ( 8.062137200540822946, 212.9164362838583315, 33.69886208192143329 ) ) ;
#13603=VERTEX_POINT ( 'NONE', #9471 ) ;
#13606=CARTESIAN_POINT ( 'NONE',  ( 6.444103211790928043, 211.7408657792734061, 15.69886208192143684 ) ) ;
#13607=CARTESIAN_POINT ( 'NONE',  ( -3.044812012440131443, 216.5253028482142952, 55.10113791807857098 ) ) ;
#13610=CARTESIAN_POINT ( 'NONE',  ( -0.05014649552810635652, 196.4853777576173002, 38.75113791807856956 ) ) ;
#13613=CARTESIAN_POINT ( 'NONE',  ( -7.984503880673422316, 204.3529502787951628, 92.34886208192143897 ) ) ;
#13616=CARTESIAN_POINT ( 'NONE',  ( -7.456977232089304408, 196.8216656703010301, 18.05113791807856316 ) ) ;
#13619=CARTESIAN_POINT ( 'NONE',  ( -6.220909254589537696, 198.5229672870051161, 69.05113791807858092 ) ) ;
#13620=CARTESIAN_POINT ( 'NONE',  ( -10.00000000000000711, 207.0476921513413515, 27.50113791807856600 ) ) ;
#13623=CARTESIAN_POINT ( 'NONE',  ( -9.984503880673420539, 203.7031108863293980, 8.348862081921435419 ) ) ;
#13627=CARTESIAN_POINT ( 'NONE',  ( 3.753561863808689836, 218.3979405102790565, 52.40113791807858235 ) ) ;
#13629=CARTESIAN_POINT ( 'NONE',  ( -6.139770520408224463, 198.4640165459539389, 23.04886208192143116 ) ) ;
#13632=CIRCLE ( 'NONE', #32667, 5.999999999999995559 ) ;
#13633=CARTESIAN_POINT ( 'NONE',  ( -3.044812012440131443, 216.5253028482142952, 76.10113791807856387 ) ) ;
#13639=CARTESIAN_POINT ( 'NONE',  ( -7.984503880673488041, 209.6470497212046098, 27.65113791807857169 ) ) ;
#13641=CARTESIAN_POINT ( 'NONE',  ( -6.139770520408224463, 198.4640165459539389, 2.048862081921434264 ) ) ;
#13649=CARTESIAN_POINT ( 'NONE',  ( 0.05014649552828275708, 196.4853777576173002, 82.74886208192143044 ) ) ;
#13651=CARTESIAN_POINT ( 'NONE',  ( -3.135527875058821579, 197.5041725223112223, 23.90113791807856813 ) ) ;
#13653=CARTESIAN_POINT ( 'NONE',  ( -7.375838497908014268, 196.7627149292498530, 83.04886208192144181 ) ) ;
#13657=CARTESIAN_POINT ( 'NONE',  ( 8.118202686958039038, 212.8392687619912635, 85.70113791807858661 ) ) ;
#13660=CARTESIAN_POINT ( 'NONE',  ( -10.00000000000000711, 207.0476921513413515, 39.50113791807856956 ) ) ;
#13664=CARTESIAN_POINT ( 'NONE',  ( -7.375838497908182134, 217.2372850707499765, 6.951137918078566180 ) ) ;
#13667=CARTESIAN_POINT ( 'NONE',  ( 6.220909254589680693, 198.5229672870052582, 91.44886208192144750 ) ) ;
#13669=CARTESIAN_POINT ( 'NONE',  ( 9.680171189290716072, 214.0920067884432854, 36.69886208192142618 ) ) ;
#13671=CARTESIAN_POINT ( 'NONE',  ( 3.135527875058820690, 216.4958274776887492, 55.40113791807857524 ) ) ;
#13673=CARTESIAN_POINT ( 'NONE',  ( 4.903702542908435547, 213.8346818373419751, 9.548862081921432932 ) ) ;
#13677=CARTESIAN_POINT ( 'NONE',  ( -8.015496119326597224, 209.5516654185217362, 89.64886208192142192 ) ) ;
#13678=CARTESIAN_POINT ( 'NONE',  ( -7.984503880673488041, 209.6470497212046098, 27.65113791807857169 ) ) ;
#13685=CARTESIAN_POINT ( 'NONE',  ( -6.500168698208129925, 202.3363017425936050, 93.20113791807858661 ) ) ;
#13687=CARTESIAN_POINT ( 'NONE',  ( 0.05014649552828262524, 198.5883022060938572, 76.74886208192144466 ) ) ;
#13691=CARTESIAN_POINT ( 'NONE',  ( 0.05014649552810506589, 217.5146222423826714, 13.25113791807856600 ) ) ;
#13696=CARTESIAN_POINT ( 'NONE',  ( 9.680171189290831535, 199.9079932115568852, 80.30113791807858092 ) ) ;
#13699=CARTESIAN_POINT ( 'NONE',  ( 3.135527875058820690, 216.4958274776887492, 100.4011379180785752 ) ) ;
#13702=CARTESIAN_POINT ( 'NONE',  ( -8.118202686958138514, 212.8392687619910930, 5.798862081921434708 ) ) ;
#13703=CARTESIAN_POINT ( 'NONE',  ( 3.662846001189864698, 218.4274158808046593, 60.39886208192143613 ) ) ;
#13704=CARTESIAN_POINT ( 'NONE',  ( 9.984503880673420539, 210.2968891136705736, 63.84886208192141765 ) ) ;
#13705=CARTESIAN_POINT ( 'NONE',  ( 3.662846001189864698, 218.4274158808046593, 3.398862081921433909 ) ) ;
#13708=CARTESIAN_POINT ( 'NONE',  ( 8.062137200540920645, 201.0835637161417822, 26.30113791807856671 ) ) ;
#13709=CARTESIAN_POINT ( 'NONE',  ( -0.05014649552828403384, 217.5146222423826714, 78.24886208192144466 ) ) ;
#13712=CARTESIAN_POINT ( 'NONE',  ( 0.05014649552810505201, 217.5146222423826714, 100.2511379180785838 ) ) ;
#13715=CARTESIAN_POINT ( 'NONE',  ( 7.984503880673422316, 209.6470497212048372, 60.84886208192144608 ) ) ;
#13719=CARTESIAN_POINT ( 'NONE',  ( 9.379977934355958169, 208.8253170565643302, -1.014254689207424676 ) ) ;
#13723=CARTESIAN_POINT ( 'NONE',  ( 2.517493886308900919, 214.5937144450984420, 70.40113791807856103 ) ) ;
#13725=FACE_OUTER_BOUND ( 'NONE', #30925, .T. ) ;
#13730=CARTESIAN_POINT ( 'NONE',  ( 6.444103211790928043, 211.7408657792734061, 42.69886208192144039 ) ) ;
#13731=CARTESIAN_POINT ( 'NONE',  ( -8.062137200540920645, 212.9164362838581894, 75.80113791807858092 ) ) ;
#13734=CARTESIAN_POINT ( 'NONE',  ( -10.00000000000000711, 207.0476921513413515, 63.50113791807856956 ) ) ;
#13737=CARTESIAN_POINT ( 'NONE',  ( 6.500168698208129925, 211.6636982574063381, 22.70113791807856529 ) ) ;
#13741=CARTESIAN_POINT ( 'NONE',  ( -7.456977232089304408, 196.8216656703010301, 51.05113791807856671 ) ) ;
#13744=CARTESIAN_POINT ( 'NONE',  ( -10.00000000000000711, 207.0476921513413515, 93.50113791807858377 ) ) ;
#13746=CARTESIAN_POINT ( 'NONE',  ( -8.118202686958039038, 201.1607312380087080, 66.20113791807857240 ) ) ;
#13747=CARTESIAN_POINT ( 'NONE',  ( -7.456977232089471386, 217.1783343296987709, 32.94886208192144039 ) ) ;
#13748=CARTESIAN_POINT ( 'NONE',  ( -3.044812012439970683, 197.4746971517856196, 37.89886208192143613 ) ) ;
#13751=CARTESIAN_POINT ( 'NONE',  ( 7.456977232089302632, 217.1783343296989131, 79.55113791807858092 ) ) ;
#13752=CARTESIAN_POINT ( 'NONE',  ( -4.903702542908602524, 213.8346818373418898, 93.95113791807857240 ) ) ;
#13754=CARTESIAN_POINT ( 'NONE',  ( 3.135527875058981895, 197.5041725223112792, 52.59886208192143897 ) ) ;
#13758=CARTESIAN_POINT ( 'NONE',  ( 11.98450388067341876, 210.9467285061363953, 57.84886208192143187 ) ) ;
#13760=CARTESIAN_POINT ( 'NONE',  ( 2.517493886309087436, 199.4062855549015865, 37.59886208192143187 ) ) ;
#13767=CARTESIAN_POINT ( 'NONE',  ( -4.984841277089726574, 200.2242689037092305, 54.05113791807856671 ) ) ;
#13769=CARTESIAN_POINT ( 'NONE',  ( -3.135527875058982783, 216.4958274776886924, 36.09886208192143897 ) ) ;
#13775=CARTESIAN_POINT ( 'NONE',  ( -4.984841277089891776, 213.7757310962905990, 14.94886208192143506 ) ) ;
#13777=CARTESIAN_POINT ( 'NONE',  ( -8.118202686958039038, 201.1607312380087080, 54.20113791807857240 ) ) ;
#13779=CARTESIAN_POINT ( 'NONE',  ( -6.139770520408369237, 215.5359834540460042, 33.95113791807855108 ) ) ;
#13782=PRODUCT_CONTEXT ( 'NONE', #6585, 'mechanical' ) ;
#13783=CARTESIAN_POINT ( 'NONE',  ( -8.000000000000008882, 206.9523078486584780, 98.49886208192143044 ) ) ;
#13787=CARTESIAN_POINT ( 'NONE',  ( 0.05014649552807549926, 219.6175466908591716, 16.25113791807856600 ) ) ;
#13790=CARTESIAN_POINT ( 'NONE',  ( 10.01549611932653860, 210.2015048109876716, 67.85113791807857808 ) ) ;
#13791=CARTESIAN_POINT ( 'NONE',  ( -6.220909254589537696, 198.5229672870051445, 39.05113791807856671 ) ) ;
#13795=CARTESIAN_POINT ( 'NONE',  ( 9.736236675708031640, 199.9851607334238963, 4.298862081921434708 ) ) ;
#13796=CARTESIAN_POINT ( 'NONE',  ( 3.044812012439969795, 216.5253028482143520, 9.398862081921436129 ) ) ;
#13799=CARTESIAN_POINT ( 'NONE',  ( 12.01549611932652972, 210.8513442034534933, 46.85113791807857098 ) ) ;
#13801=CARTESIAN_POINT ( 'NONE',  ( -3.135527875058982783, 216.4958274776886924, 18.09886208192143542 ) ) ;
#13805=CARTESIAN_POINT ( 'NONE',  ( -10.01549611932653860, 203.7984951890123284, 84.35113791807856387 ) ) ;
#13811=CARTESIAN_POINT ( 'NONE',  ( -6.500168698208129925, 202.3363017425936050, 27.20113791807857240 ) ) ;
#13813=CARTESIAN_POINT ( 'NONE',  ( -9.680171189290716072, 199.9079932115567146, 104.1988620819214475 ) ) ;
#13821=CARTESIAN_POINT ( 'NONE',  ( 10.00000000000000711, 207.0476921513415220, 87.99886208192144466 ) ) ;
#13823=CARTESIAN_POINT ( 'NONE',  ( 3.135527875058820690, 216.4958274776887492, 25.40113791807856813 ) ) ;
#13825=CARTESIAN_POINT ( 'NONE',  ( 9.680171189290716072, 214.0920067884432854, 75.69886208192143329 ) ) ;
#13831=CARTESIAN_POINT ( 'NONE',  ( -6.220909254589537696, 198.5229672870051161, 99.05113791807858092 ) ) ;
#13834=CARTESIAN_POINT ( 'NONE',  ( 10.01549611932653860, 210.2015048109876716, 40.85113791807857098 ) ) ;
#13840=CARTESIAN_POINT ( 'NONE',  ( 9.736236675707914401, 214.0148392665762458, 16.70113791807856529 ) ) ;
#13845=CARTESIAN_POINT ( 'NONE',  ( -8.118202686958138514, 212.8392687619910930, 98.79886208192144181 ) ) ;
#13846=CARTESIAN_POINT ( 'NONE',  ( 11.98450388067341876, 210.9467285061363953, 36.84886208192142476 ) ) ;
#13848=CARTESIAN_POINT ( 'NONE',  ( 8.118202686958039038, 212.8392687619912635, 49.70113791807857240 ) ) ;
#13850=CARTESIAN_POINT ( 'NONE',  ( 6.500168698208244500, 202.3363017425938324, 16.29886208192143471 ) ) ;
#13854=CARTESIAN_POINT ( 'NONE',  ( 2.517493886309087436, 199.4062855549015865, 103.5988620819214532 ) ) ;
#13856=CARTESIAN_POINT ( 'NONE',  ( 4.903702542908601636, 200.1653181626581102, 41.45113791807857240 ) ) ;
#13860=CARTESIAN_POINT ( 'NONE',  ( -8.118202686958138514, 212.8392687619910930, 62.79886208192144181 ) ) ;
#13863=CARTESIAN_POINT ( 'NONE',  ( -2.517493886308901807, 199.4062855549015012, 101.9011379180785895 ) ) ;
#13865=CARTESIAN_POINT ( 'NONE',  ( -7.984503880673422316, 204.3529502787951628, 71.34886208192142476 ) ) ;
#13869=CARTESIAN_POINT ( 'NONE',  ( 10.00000000000000711, 206.9523078486586201, 8.001137918078566003 ) ) ;
#13874=CARTESIAN_POINT ( 'NONE',  ( -11.98450388067348804, 210.9467285061362247, 72.65113791807856103 ) ) ;
#13875=CARTESIAN_POINT ( 'NONE',  ( 3.044812012440130555, 197.4746971517856764, 95.60113791807857808 ) ) ;
#13879=CARTESIAN_POINT ( 'NONE',  ( 3.753561863808876797, 195.6020594897209719, 103.5988620819214532 ) ) ;
#13880=CARTESIAN_POINT ( 'NONE',  ( 12.00000000000000711, 207.0476921513415220, 57.99886208192143044 ) ) ;
#13881=CARTESIAN_POINT ( 'NONE',  ( 6.220909254589680693, 198.5229672870052582, 70.44886208192144750 ) ) ;
#13882=CARTESIAN_POINT ( 'NONE',  ( -12.01549611932659722, 210.8513442034533227, 2.648862081921433909 ) ) ;
#13884=CARTESIAN_POINT ( 'NONE',  ( -10.01549611932653860, 203.7984951890123284, 21.35113791807855677 ) ) ;
#13885=CARTESIAN_POINT ( 'NONE',  ( -3.135527875058982783, 216.4958274776886924, 84.09886208192143897 ) ) ;
#13890=CARTESIAN_POINT ( 'NONE',  ( 2.426778023690075337, 214.6231898156240447, 72.39886208192143613 ) ) ;
#13897=B_SPLINE_CURVE_WITH_KNOTS ( 'NONE', 3,
 ( #3179, #23794, #24125, #16116, #8624, #21236, #2852, #13396, #24284, #18687, #8458, #294 ),
 .UNSPECIFIED., .F., .F.,
 ( 4, 2, 2, 2, 2, 4 ),
 ( -6.324557791138001430E-06, 0.0004602121660163784782, 0.0009267488898238950392, 0.001160017251727653428, 0.001393285613631411492, 0.001859822337438910272 ),
 .UNSPECIFIED. ) ;
#13900=CARTESIAN_POINT ( 'NONE',  ( 8.000000000000008882, 206.9523078486586485, 71.00113791807856956 ) ) ;
#13904=CARTESIAN_POINT ( 'NONE',  ( -0.05014649552828365914, 215.4116977939061144, 42.24886208192143755 ) ) ;
#13905=CARTESIAN_POINT ( 'NONE',  ( 8.118202686958039038, 212.8392687619912635, 79.70113791807857240 ) ) ;
#13906=CARTESIAN_POINT ( 'NONE',  ( 6.139770520408368348, 198.4640165459539674, 65.45113791807857240 ) ) ;
#13909=CARTESIAN_POINT ( 'NONE',  ( -2.426778023690262742, 214.6231898156240163, 25.10113791807856742 ) ) ;
#13913=CARTESIAN_POINT ( 'NONE',  ( -7.375838497908182134, 217.2372850707499765, 51.95113791807855819 ) ) ;
#13915=CARTESIAN_POINT ( 'NONE',  ( -10.01549611932653860, 203.7984951890123284, 93.35113791807857808 ) ) ;
#13916=CARTESIAN_POINT ( 'NONE',  ( 6.220909254589536808, 215.4770327129947987, 67.55113791807855250 ) ) ;
#13917=CARTESIAN_POINT ( 'NONE',  ( 7.375838497908012492, 217.2372850707501186, 33.54886208192143471 ) ) ;
#13918=CARTESIAN_POINT ( 'NONE',  ( -6.220909254589682469, 215.4770327129947134, 38.94886208192143329 ) ) ;
#13920=CARTESIAN_POINT ( 'NONE',  ( -3.662846001190052991, 218.4274158808045740, 76.10113791807854966 ) ) ;
#13921=CARTESIAN_POINT ( 'NONE',  ( 2.426778023690261410, 199.3768101843759837, 95.60113791807857808 ) ) ;
#13923=CARTESIAN_POINT ( 'NONE',  ( -8.062137200540822946, 201.0835637161416400, 56.19886208192144039 ) ) ;
#13925=CARTESIAN_POINT ( 'NONE',  ( -9.680171189290716072, 199.9079932115567146, 59.19886208192144750 ) ) ;
#13927=CARTESIAN_POINT ( 'NONE',  ( 2.426778023690075337, 214.6231898156240447, 36.39886208192144323 ) ) ;
#13930=AXIS2_PLACEMENT_3D ( 'NONE', #1097, #6877, #19657 ) ;
#13934=CARTESIAN_POINT ( 'NONE',  ( 8.000000000000008882, 206.9523078486586485, 50.00113791807856956 ) ) ;
#13937=CARTESIAN_POINT ( 'NONE',  ( -3.044812012439970683, 197.4746971517856196, 28.89886208192143613 ) ) ;
#13944=CARTESIAN_POINT ( 'NONE',  ( -2.517493886309087880, 214.5937144450984135, 18.09886208192143187 ) ) ;
#13945=CARTESIAN_POINT ( 'NONE',  ( -10.00000000000000711, 207.0476921513413515, 48.50113791807856956 ) ) ;
#13946=CARTESIAN_POINT ( 'NONE',  ( -8.062137200540920645, 212.9164362838581894, 33.80113791807857382 ) ) ;
#13948=SHAPE_DEFINITION_REPRESENTATION ( #4537, #21975 ) ;
#13949=CARTESIAN_POINT ( 'NONE',  ( -2.426778023690076225, 199.3768101843759553, 97.89886208192146455 ) ) ;
#13953=CARTESIAN_POINT ( 'NONE',  ( -7.375838497908182134, 217.2372850707499765, 15.95113791807856707 ) ) ;
#13956=CARTESIAN_POINT ( 'NONE',  ( 8.062137200540920645, 201.0835637161417822, 68.30113791807856671 ) ) ;
#13957=CARTESIAN_POINT ( 'NONE',  ( 6.139770520408367460, 198.4640165459539389, 41.45113791807857240 ) ) ;
#13959=CARTESIAN_POINT ( 'NONE',  ( 9.680171189290716072, 214.0920067884432854, 3.698862081921433731 ) ) ;
#13960=CARTESIAN_POINT ( 'NONE',  ( -10.01549611932659545, 210.2015048109875011, 11.64886208192143435 ) ) ;
#13963=CARTESIAN_POINT ( 'NONE',  ( -9.680171189290831535, 214.0920067884431148, 48.80113791807857382 ) ) ;
#13964=CARTESIAN_POINT ( 'NONE',  ( -8.000000000000008882, 207.0476921513413515, 66.50113791807856956 ) ) ;
#13966=CARTESIAN_POINT ( 'NONE',  ( 8.062137200540822946, 212.9164362838583315, 18.69886208192143329 ) ) ;
#13970=ORIENTED_EDGE ( 'NONE', *, *, #7388, .T. ) ;
#13971=CARTESIAN_POINT ( 'NONE',  ( 3.135527875058820690, 216.4958274776887492, 85.40113791807857524 ) ) ;
#13977=CARTESIAN_POINT ( 'NONE',  ( -2.426778023690262742, 214.6231898156240163, 22.10113791807856742 ) ) ;
#13980=CARTESIAN_POINT ( 'NONE',  ( -6.220909254589682469, 215.4770327129946850, 2.948862081921434175 ) ) ;
#13988=CARTESIAN_POINT ( 'NONE',  ( -8.062137200540822946, 201.0835637161416400, 89.19886208192144750 ) ) ;
#13990=CARTESIAN_POINT ( 'NONE',  ( -10.01549611932653860, 203.7984951890123284, 27.35113791807856742 ) ) ;
#13992=CARTESIAN_POINT ( 'NONE',  ( 7.456977232089471386, 196.8216656703012006, 79.44886208192144750 ) ) ;
#13996=CARTESIAN_POINT ( 'NONE',  ( 9.443650191645208025, 207.8375535574373032, -0.8718850525427659370 ) ) ;
#13997=CARTESIAN_POINT ( 'NONE',  ( -10.00000000000000711, 207.0476921513413515, 96.50113791807856956 ) ) ;
#14000=CARTESIAN_POINT ( 'NONE',  ( 8.062137200540920645, 201.0835637161417822, 38.30113791807857382 ) ) ;
#14005=CARTESIAN_POINT ( 'NONE',  ( -12.00000000000000711, 207.0476921513413515, 21.50113791807856956 ) ) ;
#14010=ORIENTED_EDGE ( 'NONE', *, *, #29028, .F. ) ;
#14011=CARTESIAN_POINT ( 'NONE',  ( -3.662846001189865142, 195.5725841191952838, 31.89886208192143613 ) ) ;
#14013=CARTESIAN_POINT ( 'NONE',  ( 8.062137200540920645, 201.0835637161417822, 53.30113791807857382 ) ) ;
#14015=CARTESIAN_POINT ( 'NONE',  ( 6.500168698208244500, 202.3363017425938324, 13.29886208192143826 ) ) ;
#14019=CARTESIAN_POINT ( 'NONE',  ( -2.517493886309087880, 214.5937144450984135, 96.09886208192143897 ) ) ;
#14020=CARTESIAN_POINT ( 'NONE',  ( -4.984841277089726574, 200.2242689037092305, 36.05113791807856671 ) ) ;
#14025=CARTESIAN_POINT ( 'NONE',  ( 6.139770520408223575, 215.5359834540460611, 60.54886208192143471 ) ) ;
#14028=CARTESIAN_POINT ( 'NONE',  ( -8.015496119326531499, 204.4483345814780364, 102.3511379180785639 ) ) ;
#14033=CARTESIAN_POINT ( 'NONE',  ( 8.015496119326595448, 204.4483345814782638, 76.14886208192143613 ) ) ;
#14038=CARTESIAN_POINT ( 'NONE',  ( -9.984503880673475606, 210.2968891136704315, 9.651137918078566358 ) ) ;
#14043=CARTESIAN_POINT ( 'NONE',  ( 3.753561863808689836, 218.3979405102790565, 79.40113791807858945 ) ) ;
#14044=CARTESIAN_POINT ( 'NONE',  ( -10.00000000000000711, 207.0476921513413515, 93.50113791807858377 ) ) ;
#14045=CARTESIAN_POINT ( 'NONE',  ( -10.00000000000000178, 208.0352956435529563, 102.7846294209004441 ) ) ;
#14046=VERTEX_POINT ( 'NONE', #27641 ) ;
#14047=CARTESIAN_POINT ( 'NONE',  ( 9.984503880673420539, 210.2968891136705167, 3.848862081921433642 ) ) ;
#14048=CARTESIAN_POINT ( 'NONE',  ( -7.375838497908014268, 196.7627149292498530, 62.04886208192144181 ) ) ;
#14049=CARTESIAN_POINT ( 'NONE',  ( 6.220909254589680693, 198.5229672870052582, 67.44886208192143329 ) ) ;
#14050=CARTESIAN_POINT ( 'NONE',  ( 3.753561863808876797, 195.6020594897209719, 4.598862081921434530 ) ) ;
#14052=CARTESIAN_POINT ( 'NONE',  ( -9.984503880673473830, 210.2968891136704315, 27.65113791807855748 ) ) ;
#14053=CARTESIAN_POINT ( 'NONE',  ( 0.05014649552828275708, 196.4853777576173002, 88.74886208192140202 ) ) ;
#14058=CARTESIAN_POINT ( 'NONE',  ( 0.05014649552828262524, 198.5883022060938572, 73.74886208192144466 ) ) ;
#14066=CARTESIAN_POINT ( 'NONE',  ( -4.984841277089726574, 200.2242689037092305, 66.05113791807858092 ) ) ;
#14069=CARTESIAN_POINT ( 'NONE',  ( 8.015496119326595448, 204.4483345814782638, 43.14886208192144323 ) ) ;
#14071=CARTESIAN_POINT ( 'NONE',  ( -10.01549611932653860, 203.7984951890123284, 90.35113791807857808 ) ) ;
#14072=CARTESIAN_POINT ( 'NONE',  ( -6.139770520408369237, 215.5359834540460042, 66.95113791807858661 ) ) ;
#14074=CARTESIAN_POINT ( 'NONE',  ( 8.062137200540920645, 201.0835637161417822, 89.30113791807858092 ) ) ;
#14076=CARTESIAN_POINT ( 'NONE',  ( 4.903702542908601636, 200.1653181626581102, 23.45113791807856884 ) ) ;
#14080=CARTESIAN_POINT ( 'NONE',  ( 9.680171189290831535, 199.9079932115568852, 44.30113791807857382 ) ) ;
#14082=CARTESIAN_POINT ( 'NONE',  ( -9.984503880673473830, 210.2968891136704315, 90.65113791807854682 ) ) ;
#14083=CARTESIAN_POINT ( 'NONE',  ( 0.05014649552810506589, 217.5146222423826714, 73.25113791807855534 ) ) ;
#14085=CARTESIAN_POINT ( 'NONE',  ( 9.736236675708031640, 199.9851607334238963, 37.29886208192143471 ) ) ;
#14086=CARTESIAN_POINT ( 'NONE',  ( -8.118202686958138514, 212.8392687619910930, 41.79886208192143471 ) ) ;
#14088=CARTESIAN_POINT ( 'NONE',  ( -9.680171189290831535, 214.0920067884431148, 81.80113791807858092 ) ) ;
#14089=CARTESIAN_POINT ( 'NONE',  ( -0.05014649552807731031, 198.5883022060938572, 98.75113791807856956 ) ) ;
#14091=CARTESIAN_POINT ( 'NONE',  ( 10.01549611932659545, 203.7984951890123853, 61.14886208192144323 ) ) ;
#14094=CARTESIAN_POINT ( 'NONE',  ( -9.680171189290716072, 199.9079932115567146, 62.19886208192144039 ) ) ;
#14097=CARTESIAN_POINT ( 'NONE',  ( -7.984503880673422316, 204.3529502787951628, 38.34886208192142476 ) ) ;
#14103=CARTESIAN_POINT ( 'NONE',  ( -8.015496119326531499, 204.4483345814780364, 54.35113791807857098 ) ) ;
#14105=CARTESIAN_POINT ( 'NONE',  ( -8.118202686958138514, 212.8392687619910930, 29.79886208192143826 ) ) ;
#14114=CARTESIAN_POINT ( 'NONE',  ( -2.517493886309087880, 214.5937144450984135, 15.09886208192143719 ) ) ;
#14115=CARTESIAN_POINT ( 'NONE',  ( -0.05014649552810635652, 196.4853777576173002, 62.75113791807856956 ) ) ;
#14116=CARTESIAN_POINT ( 'NONE',  ( 6.220909254589536808, 215.4770327129947702, 37.55113791807856671 ) ) ;
#14118=CARTESIAN_POINT ( 'NONE',  ( -0.05014649552807731031, 198.5883022060938572, -0.2488620819214341084 ) ) ;
#14122=CARTESIAN_POINT ( 'NONE',  ( 3.753561863808689836, 218.3979405102790565, 16.40113791807856458 ) ) ;
#14125=EDGE_CURVE ( 'NONE', #17153, #14862, #9978, .T. ) ;
#14126=CARTESIAN_POINT ( 'NONE',  ( 3.135527875058820690, 216.4958274776887492, 61.40113791807857524 ) ) ;
#14127=CARTESIAN_POINT ( 'NONE',  ( 10.00000000000000711, 206.9523078486586201, 44.00113791807857666 ) ) ;
#14130=CARTESIAN_POINT ( 'NONE',  ( 12.01549611932659367, 203.1486557965466773, 7.148862081921435241 ) ) ;
#14131=CARTESIAN_POINT ( 'NONE',  ( 10.01549611932659367, 203.7984951890124421, 10.14886208192143435 ) ) ;
#14134=CARTESIAN_POINT ( 'NONE',  ( 3.753561863808689836, 218.3979405102790565, 49.40113791807856813 ) ) ;
#14135=CARTESIAN_POINT ( 'NONE',  ( 4.903702542908601636, 200.1653181626581102, 71.45113791807854398 ) ) ;
#14136=ADVANCED_FACE ( 'NONE', ( #24591 ), #14314, .T. ) ;
#14138=CARTESIAN_POINT ( 'NONE',  ( -9.984503880673420539, 203.7031108863293980, 35.34886208192142476 ) ) ;
#14141=CARTESIAN_POINT ( 'NONE',  ( 6.220909254589536808, 215.4770327129947702, 76.55113791807855250 ) ) ;
#14146=CARTESIAN_POINT ( 'NONE',  ( 7.984503880673485376, 204.3529502787953902, 20.15113791807856458 ) ) ;
#14148=CARTESIAN_POINT ( 'NONE',  ( 3.044812012439969795, 216.5253028482143520, 3.398862081921434797 ) ) ;
#14152=CARTESIAN_POINT ( 'NONE',  ( -7.984503880673488041, 209.6470497212046098, 48.65113791807857524 ) ) ;
#14156=CARTESIAN_POINT ( 'NONE',  ( 3.044812012439969795, 216.5253028482143520, 93.39886208192143613 ) ) ;
#14158=CARTESIAN_POINT ( 'NONE',  ( -6.220909254589537696, 198.5229672870051161, 18.05113791807856671 ) ) ;
#14162=CARTESIAN_POINT ( 'NONE',  ( 9.736236675708031640, 199.9851607334238963, 79.29886208192144181 ) ) ;
#14167=CARTESIAN_POINT ( 'NONE',  ( -3.044812012440131443, 216.5253028482142952, 94.10113791807857808 ) ) ;
#14171=CARTESIAN_POINT ( 'NONE',  ( -3.135527875058821579, 197.5041725223112223, 41.90113791807856813 ) ) ;
#14177=CARTESIAN_POINT ( 'NONE',  ( 9.736236675707914401, 214.0148392665762458, 22.70113791807856529 ) ) ;
#14179=CARTESIAN_POINT ( 'NONE',  ( -10.66474937096564624, 207.8127639808361948, 102.7602103102857996 ) ) ;
#14182=CARTESIAN_POINT ( 'NONE',  ( 7.456977232089471386, 196.8216656703012006, 40.44886208192144039 ) ) ;
#14184=CARTESIAN_POINT ( 'NONE',  ( -6.139770520408369237, 215.5359834540460042, 54.95113791807856529 ) ) ;
#14185=CARTESIAN_POINT ( 'NONE',  ( 2.426778023690075337, 214.6231898156240447, 18.39886208192143613 ) ) ;
#14190=CARTESIAN_POINT ( 'NONE',  ( -8.000000000000008882, 206.9523078486584780, 101.4988620819214304 ) ) ;
#14192=CARTESIAN_POINT ( 'NONE',  ( 0.05014649552807626948, 215.4116977939061144, 37.25113791807857666 ) ) ;
#14196=CARTESIAN_POINT ( 'NONE',  ( -6.220909254589682469, 215.4770327129946850, 62.94886208192143329 ) ) ;
#14199=CARTESIAN_POINT ( 'NONE',  ( -2.426778023690262742, 214.6231898156240163, 97.10113791807857808 ) ) ;
#14203=CARTESIAN_POINT ( 'NONE',  ( -4.903702542908436435, 200.1653181626580249, 83.04886208192144181 ) ) ;
#14207=CARTESIAN_POINT ( 'NONE',  ( 6.139770520408367460, 198.4640165459539389, 20.45113791807856174 ) ) ;
#14212=CARTESIAN_POINT ( 'NONE',  ( -3.662846001190052991, 218.4274158808045740, 88.10113791807857808 ) ) ;
#14213=CARTESIAN_POINT ( 'NONE',  ( 0.05014649552810506589, 217.5146222423826714, 94.25113791807856956 ) ) ;
#14216=CARTESIAN_POINT ( 'NONE',  ( 9.984503880673420539, 210.2968891136705167, 6.848862081921434530 ) ) ;
#14217=CARTESIAN_POINT ( 'NONE',  ( 11.98450388067341876, 210.9467285061363953, 63.84886208192143187 ) ) ;
#14218=CARTESIAN_POINT ( 'NONE',  ( -3.135527875058982783, 216.4958274776886924, 72.09886208192143897 ) ) ;
#14219=CARTESIAN_POINT ( 'NONE',  ( 3.662846001189864698, 218.4274158808046593, 15.39886208192143613 ) ) ;
#14221=CARTESIAN_POINT ( 'NONE',  ( 6.139770520408368348, 198.4640165459539674, 23.45113791807856884 ) ) ;
#14222=CARTESIAN_POINT ( 'NONE',  ( 3.044812012439969795, 216.5253028482143520, 84.39886208192143613 ) ) ;
#14228=CARTESIAN_POINT ( 'NONE',  ( -6.500168698208244500, 211.6636982574061676, 74.79886208192142760 ) ) ;
#14235=CARTESIAN_POINT ( 'NONE',  ( 2.426778023690261410, 199.3768101843759837, 71.60113791807857808 ) ) ;
#14239=CARTESIAN_POINT ( 'NONE',  ( -4.984841277089891776, 213.7757310962905990, 44.94886208192144039 ) ) ;
#14240=CARTESIAN_POINT ( 'NONE',  ( -8.062137200540920645, 212.9164362838581894, 93.80113791807858092 ) ) ;
#14241=CARTESIAN_POINT ( 'NONE',  ( 9.984503880673470277, 203.7031108863295401, 71.15113791807857524 ) ) ;
#14242=DIRECTION ( 'NONE',  ( 0.000000000000000000, 0.000000000000000000, 1.000000000000000000 ) ) ;
#14246=CARTESIAN_POINT ( 'NONE',  ( 9.736236675707914401, 214.0148392665762458, 52.70113791807856529 ) ) ;
#14248=CARTESIAN_POINT ( 'NONE',  ( 3.753561863808689836, 218.3979405102790565, 4.401137918078566358 ) ) ;
#14250=CARTESIAN_POINT ( 'NONE',  ( 10.01549611932653860, 210.2015048109876716, 64.85113791807857808 ) ) ;
#14251=CARTESIAN_POINT ( 'NONE',  ( 12.01549611932659367, 203.1486557965466773, 28.14886208192143968 ) ) ;
#14252=CARTESIAN_POINT ( 'NONE',  ( -0.05014649552828402690, 217.5146222423826714, 48.24886208192143044 ) ) ;
#14253=AXIS2_PLACEMENT_3D ( 'NONE', #1387, #30693, #11775 ) ;
#14255=CARTESIAN_POINT ( 'NONE',  ( -12.01549611932652972, 203.1486557965464499, 75.35113791807856387 ) ) ;
#14256=CARTESIAN_POINT ( 'NONE',  ( 6.444103211791042618, 202.2591342207267644, 101.3011379180785951 ) ) ;
#14257=CARTESIAN_POINT ( 'NONE',  ( 3.135527875058981895, 197.5041725223112792, 55.59886208192143187 ) ) ;
#14260=CARTESIAN_POINT ( 'NONE',  ( -0.05014649552828442242, 219.6175466908591716, 60.24886208192143755 ) ) ;
#14263=CARTESIAN_POINT ( 'NONE',  ( 4.903702542908435547, 213.8346818373419751, 45.54886208192144181 ) ) ;
#14269=CARTESIAN_POINT ( 'NONE',  ( 7.984503880673485376, 204.3529502787953902, 47.15113791807857524 ) ) ;
#14271=CARTESIAN_POINT ( 'NONE',  ( -6.220909254589682469, 215.4770327129946850, 32.94886208192144039 ) ) ;
#14278=CARTESIAN_POINT ( 'NONE',  ( 8.000000000000008882, 207.0476921513415220, 15.99886208192143577 ) ) ;
#14279=CARTESIAN_POINT ( 'NONE',  ( 6.139770520408368348, 198.4640165459539674, 62.45113791807857950 ) ) ;
#14280=CARTESIAN_POINT ( 'NONE',  ( 3.044812012440130555, 197.4746971517856764, 38.60113791807857098 ) ) ;
#14282=CARTESIAN_POINT ( 'NONE',  ( -4.984841277089891776, 213.7757310962905990, 101.9488620819214475 ) ) ;
#14287=CARTESIAN_POINT ( 'NONE',  ( 9.680171189290831535, 199.9079932115568852, 17.30113791807856671 ) ) ;
#14290=CARTESIAN_POINT ( 'NONE',  ( -6.220909254589537696, 198.5229672870051161, 63.05113791807858092 ) ) ;
#14292=CARTESIAN_POINT ( 'NONE',  ( -8.118202686958039038, 201.1607312380087080, 42.20113791807857240 ) ) ;
#14295=CARTESIAN_POINT ( 'NONE',  ( 3.753561863808876797, 195.6020594897209719, 7.598862081921434530 ) ) ;
#14296=CARTESIAN_POINT ( 'NONE',  ( 9.984503880673420539, 210.2968891136705736, 12.84886208192143364 ) ) ;
#14299=CARTESIAN_POINT ( 'NONE',  ( 9.736236675707914401, 214.0148392665762458, 46.70113791807857240 ) ) ;
#14301=CARTESIAN_POINT ( 'NONE',  ( -7.984503880673488041, 209.6470497212046098, 72.65113791807856103 ) ) ;
#14302=CARTESIAN_POINT ( 'NONE',  ( -10.00000000000000711, 206.9523078486584495, 26.49886208192143755 ) ) ;
#14307=CARTESIAN_POINT ( 'NONE',  ( 3.135527875058820690, 216.4958274776887492, 88.40113791807857524 ) ) ;
#14313=CARTESIAN_POINT ( 'NONE',  ( -0.05014649552807731031, 198.5883022060938572, 26.75113791807856956 ) ) ;
#14314=TOROIDAL_SURFACE ( 'NONE', #8267, 9.624472924841564136, 1.000000000000000444 ) ;
#14317=DIRECTION ( 'NONE',  ( 0.000000000000000000, -0.04769215134144316748, 0.9988620819214356628 ) ) ;
#14318=CARTESIAN_POINT ( 'NONE',  ( -10.01549611932659722, 210.2015048109875011, 2.648862081921434797 ) ) ;
#14322=CARTESIAN_POINT ( 'NONE',  ( -8.000000000000008882, 207.0476921513413515, 51.50113791807856956 ) ) ;
#14326=CARTESIAN_POINT ( 'NONE',  ( -10.00000000000000711, 206.9523078486584495, 86.49886208192144466 ) ) ;
#14329=CARTESIAN_POINT ( 'NONE',  ( -10.00000000000000711, 207.0476921513413515, 30.50113791807856600 ) ) ;
#14331=CARTESIAN_POINT ( 'NONE',  ( 7.456977232089471386, 196.8216656703012006, 76.44886208192143329 ) ) ;
#14338=CARTESIAN_POINT ( 'NONE',  ( -10.00000000000000711, 207.0476921513413515, 99.50113791807856956 ) ) ;
#14341=CARTESIAN_POINT ( 'NONE',  ( 3.044812012440130555, 197.4746971517856764, 32.60113791807857098 ) ) ;
#14348=CARTESIAN_POINT ( 'NONE',  ( 12.01549611932652972, 210.8513442034534933, 16.85113791807856742 ) ) ;
#14354=CARTESIAN_POINT ( 'NONE',  ( -7.375838497908014268, 196.7627149292498530, 38.04886208192144181 ) ) ;
#14355=CARTESIAN_POINT ( 'NONE',  ( -10.01549611932653860, 203.7984951890123284, 0.3511379180785655363 ) ) ;
#14356=CARTESIAN_POINT ( 'NONE',  ( -10.00000000000000711, 207.0476921513413515, 63.50113791807856956 ) ) ;
#14357=CARTESIAN_POINT ( 'NONE',  ( 8.000000000000008882, 207.0476921513415220, 12.99886208192143400 ) ) ;
#14362=CARTESIAN_POINT ( 'NONE',  ( -8.050845014156799095, 215.4811768934071665, 104.9910338291041114 ) ) ;
#14365=CARTESIAN_POINT ( 'NONE',  ( -0.05014649552807731031, 198.5883022060938572, 41.75113791807856956 ) ) ;
#14371=CARTESIAN_POINT ( 'NONE',  ( -0.05014649552828403384, 217.5146222423826714, 63.24886208192143755 ) ) ;
#14376=CARTESIAN_POINT ( 'NONE',  ( -10.00000000000000711, 207.0476921513413515, 6.501137918078566003 ) ) ;
#14379=CARTESIAN_POINT ( 'NONE',  ( 7.984503880673422316, 209.6470497212048372, 81.84886208192142476 ) ) ;
#14384=CARTESIAN_POINT ( 'NONE',  ( 3.135527875058820690, 216.4958274776887492, 22.40113791807856458 ) ) ;
#14388=CARTESIAN_POINT ( 'NONE',  ( -11.98450388067348804, 210.9467285061362247, 87.65113791807857524 ) ) ;
#14392=CARTESIAN_POINT ( 'NONE',  ( -3.662846001189865142, 195.5725841191952838, 70.89886208192143613 ) ) ;
#14393=CARTESIAN_POINT ( 'NONE',  ( -0.05014649552828402690, 217.5146222423826714, 81.24886208192141623 ) ) ;
#14395=CARTESIAN_POINT ( 'NONE',  ( 3.662846001189864698, 218.4274158808046593, 12.39886208192143613 ) ) ;
#14397=CARTESIAN_POINT ( 'NONE',  ( -10.01549611932653860, 203.7984951890123284, 24.35113791807855677 ) ) ;
#14398=CARTESIAN_POINT ( 'NONE',  ( -10.00000000000000711, 206.9523078486584495, 89.49886208192144466 ) ) ;
#14403=CARTESIAN_POINT ( 'NONE',  ( 8.000000000000008882, 207.0476921513415220, 75.99886208192144466 ) ) ;
#14410=CARTESIAN_POINT ( 'NONE',  ( 2.517493886308900919, 214.5937144450984420, 64.40113791807856103 ) ) ;
#14413=CARTESIAN_POINT ( 'NONE',  ( -0.05014649552828365914, 215.4116977939061144, 51.24886208192144466 ) ) ;
#14418=CARTESIAN_POINT ( 'NONE',  ( 9.680171189290831535, 199.9079932115568852, 59.30113791807857382 ) ) ;
#14420=CARTESIAN_POINT ( 'NONE',  ( -9.898309971686792608, 228.3698647632124334, 103.4854814124440452 ) ) ;
#14421=CARTESIAN_POINT ( 'NONE',  ( 6.220909254589536808, 215.4770327129947987, 76.55113791807856671 ) ) ;
#14422=CARTESIAN_POINT ( 'NONE',  ( -7.375838497908014268, 196.7627149292498530, 44.04886208192143471 ) ) ;
#14423=CARTESIAN_POINT ( 'NONE',  ( -0.05014649552828402690, 217.5146222423826714, 45.24886208192143755 ) ) ;
#14426=CARTESIAN_POINT ( 'NONE',  ( -3.662846001190052991, 218.4274158808045740, 85.10113791807857808 ) ) ;
#14427=CARTESIAN_POINT ( 'NONE',  ( -7.984503880673488041, 209.6470497212046098, 93.65113791807857524 ) ) ;
#14428=CARTESIAN_POINT ( 'NONE',  ( -0.05014649552828403384, 217.5146222423826714, 57.24886208192144466 ) ) ;
#14431=CARTESIAN_POINT ( 'NONE',  ( -7.456977232089471386, 217.1783343296987709, 65.94886208192144750 ) ) ;
#14432=ORIENTED_EDGE ( 'NONE', *, *, #30843, .F. ) ;
#14434=CARTESIAN_POINT ( 'NONE',  ( -0.05014649552828365914, 215.4116977939061144, 39.24886208192144466 ) ) ;
#14440=CARTESIAN_POINT ( 'NONE',  ( -7.984503880673488041, 209.6470497212046098, 60.65113791807856813 ) ) ;
#14442=CARTESIAN_POINT ( 'NONE',  ( -6.139770520408224463, 198.4640165459539389, 47.04886208192142050 ) ) ;
#14447=CARTESIAN_POINT ( 'NONE',  ( -2.426778023690076225, 199.3768101843759553, 25.89886208192143613 ) ) ;
#14448=CARTESIAN_POINT ( 'NONE',  ( 10.01549611932653860, 210.2015048109876716, 58.85113791807856387 ) ) ;
#14449=CARTESIAN_POINT ( 'NONE',  ( 8.118202686958039038, 212.8392687619912635, 43.70113791807857240 ) ) ;
#14451=CARTESIAN_POINT ( 'NONE',  ( -6.220909254589537696, 198.5229672870051161, 21.05113791807855961 ) ) ;
#14452=CARTESIAN_POINT ( 'NONE',  ( 4.903702542908435547, 213.8346818373419751, 102.5488620819214560 ) ) ;
#14455=CARTESIAN_POINT ( 'NONE',  ( 9.736236675707914401, 214.0148392665762458, 25.70113791807857240 ) ) ;
#14457=CARTESIAN_POINT ( 'NONE',  ( -10.01549611932653860, 203.7984951890123284, 78.35113791807857808 ) ) ;
#14458=CARTESIAN_POINT ( 'NONE',  ( 8.118202686958039038, 212.8392687619912635, 46.70113791807857240 ) ) ;
#14461=CARTESIAN_POINT ( 'NONE',  ( -11.94915498584342295, 219.8409957184640291, 102.9933096652613642 ) ) ;
#14462=CARTESIAN_POINT ( 'NONE',  ( 0.05014649552828275014, 196.4853777576173002, 19.74886208192143400 ) ) ;
#14465=CARTESIAN_POINT ( 'NONE',  ( -3.753561863808691168, 195.6020594897209435, 59.90113791807856103 ) ) ;
#14466=CARTESIAN_POINT ( 'NONE',  ( -7.984503880673488041, 209.6470497212046098, 66.65113791807856103 ) ) ;
#14467=CARTESIAN_POINT ( 'NONE',  ( 9.984503880673420539, 210.2968891136705167, 27.84886208192143187 ) ) ;
#14471=CARTESIAN_POINT ( 'NONE',  ( -0.05014649552810635652, 196.4853777576173002, 86.75113791807858377 ) ) ;
#14476=CARTESIAN_POINT ( 'NONE',  ( -6.500168698208129925, 202.3363017425936050, 30.20113791807856529 ) ) ;
#14479=CARTESIAN_POINT ( 'NONE',  ( -0.05014649552828403384, 217.5146222423826714, 18.24886208192143755 ) ) ;
#14482=CARTESIAN_POINT ( 'NONE',  ( -4.903702542908602524, 213.8346818373418898, 51.95113791807857240 ) ) ;
#14485=CARTESIAN_POINT ( 'NONE',  ( -9.984503880673420539, 203.7031108863293980, 86.34886208192143897 ) ) ;
#14487=CARTESIAN_POINT ( 'NONE',  ( -8.062137200540920645, 212.9164362838581894, 33.80113791807857382 ) ) ;
#14489=CARTESIAN_POINT ( 'NONE',  ( 8.118202686958039038, 212.8392687619912635, 22.70113791807856884 ) ) ;
#14496=CARTESIAN_POINT ( 'NONE',  ( 8.062137200540920645, 201.0835637161417822, 92.30113791807858092 ) ) ;
#14499=CARTESIAN_POINT ( 'NONE',  ( -3.135527875058821579, 197.5041725223112223, 47.90113791807857524 ) ) ;
#14506=CARTESIAN_POINT ( 'NONE',  ( -12.01549611932652972, 203.1486557965464499, 21.35113791807856742 ) ) ;
#14510=CARTESIAN_POINT ( 'NONE',  ( 9.736236675708031640, 199.9851607334238963, 43.29886208192143471 ) ) ;
#14512=CARTESIAN_POINT ( 'NONE',  ( -8.118202686958039038, 201.1607312380087080, 60.20113791807857240 ) ) ;
#14514=CARTESIAN_POINT ( 'NONE',  ( -8.015496119326597224, 209.5516654185217362, 26.64886208192143968 ) ) ;
#14518=CARTESIAN_POINT ( 'NONE',  ( 2.426778023690075337, 214.6231898156240447, 99.39886208192146455 ) ) ;
#14521=CARTESIAN_POINT ( 'NONE',  ( 6.444103211791042618, 202.2591342207267644, 38.30113791807856671 ) ) ;
#14527=CARTESIAN_POINT ( 'NONE',  ( -8.118202686958039038, 201.1607312380087080, 3.201137918078566180 ) ) ;
#14528=CARTESIAN_POINT ( 'NONE',  ( -0.05014649552828403384, 217.5146222423826714, 57.24886208192144466 ) ) ;
#14531=CARTESIAN_POINT ( 'NONE',  ( 10.00000000000000711, 206.9523078486586201, 2.001137918078565558 ) ) ;
#14536=CARTESIAN_POINT ( 'NONE',  ( -2.517493886309087880, 214.5937144450984135, 78.09886208192142476 ) ) ;
#14543=CARTESIAN_POINT ( 'NONE',  ( -10.00000000000000711, 207.0476921513413515, 18.50113791807856956 ) ) ;
#14548=CARTESIAN_POINT ( 'NONE',  ( 3.753561863808689836, 218.3979405102790565, 82.40113791807856103 ) ) ;
#14552=ORIENTED_EDGE ( 'NONE', *, *, #7998, .T. ) ;
#14553=CARTESIAN_POINT ( 'NONE',  ( -7.456977232089471386, 217.1783343296987709, 71.94886208192144750 ) ) ;
#14554=CARTESIAN_POINT ( 'NONE',  ( 3.135527875058981895, 197.5041725223112792, 79.59886208192143897 ) ) ;
#14555=CARTESIAN_POINT ( 'NONE',  ( 3.753561863808876797, 195.6020594897209719, 16.59886208192143187 ) ) ;
#14557=CARTESIAN_POINT ( 'NONE',  ( 10.01549611932653860, 210.2015048109876716, 31.85113791807857453 ) ) ;
#14559=CARTESIAN_POINT ( 'NONE',  ( 0.05014649552828275708, 196.4853777576173002, 85.74886208192140202 ) ) ;
#14563=CARTESIAN_POINT ( 'NONE',  ( -6.500168698208244500, 211.6636982574061676, 71.79886208192142760 ) ) ;
#14573=CARTESIAN_POINT ( 'NONE',  ( 6.444103211791042618, 202.2591342207267644, 77.30113791807858092 ) ) ;
#14577=CARTESIAN_POINT ( 'NONE',  ( 4.903702542908435547, 213.8346818373419751, 54.54886208192144181 ) ) ;
#14585=CARTESIAN_POINT ( 'NONE',  ( 3.753561863808689836, 218.3979405102790565, 61.40113791807856103 ) ) ;
#14590=CARTESIAN_POINT ( 'NONE',  ( 9.680171189290831535, 199.9079932115568852, 5.301137918078565825 ) ) ;
#14592=CARTESIAN_POINT ( 'NONE',  ( 3.044812012440130555, 197.4746971517856764, 80.60113791807857808 ) ) ;
#14594=CARTESIAN_POINT ( 'NONE',  ( 3.662846001189864698, 218.4274158808046593, 42.39886208192144323 ) ) ;
#14595=CARTESIAN_POINT ( 'NONE',  ( -3.135527875058982783, 216.4958274776886924, 45.09886208192143897 ) ) ;
#14597=CARTESIAN_POINT ( 'NONE',  ( 7.375838497908181246, 196.7627149292499666, 89.45113791807857240 ) ) ;
#14598=CARTESIAN_POINT ( 'NONE',  ( 6.220909254589536808, 215.4770327129947702, 7.551137918078564049 ) ) ;
#14600=CARTESIAN_POINT ( 'NONE',  ( -10.00000000000000711, 206.9523078486584495, 62.49886208192143755 ) ) ;
#14603=CARTESIAN_POINT ( 'NONE',  ( 7.375838497908012492, 217.2372850707501186, 69.54886208192141339 ) ) ;
#14606=CARTESIAN_POINT ( 'NONE',  ( 0.05014649552828262524, 198.5883022060938572, 46.74886208192144466 ) ) ;
#14611=CARTESIAN_POINT ( 'NONE',  ( -8.000000000000008882, 207.0476921513413515, 63.50113791807856956 ) ) ;
#14614=CARTESIAN_POINT ( 'NONE',  ( -3.044812012439970683, 197.4746971517856196, 43.89886208192142902 ) ) ;
#14620=CARTESIAN_POINT ( 'NONE',  ( 7.984503880673422316, 209.6470497212048372, 24.84886208192143897 ) ) ;
#14621=CARTESIAN_POINT ( 'NONE',  ( 6.139770520408368348, 198.4640165459539674, 65.45113791807857240 ) ) ;
#14622=CARTESIAN_POINT ( 'NONE',  ( 8.062137200540920645, 201.0835637161417822, 50.30113791807857382 ) ) ;
#14625=CARTESIAN_POINT ( 'NONE',  ( 6.220909254589536808, 215.4770327129947702, 13.55113791807856849 ) ) ;
#14626=CARTESIAN_POINT ( 'NONE',  ( 2.426778023690261410, 199.3768101843759837, 8.601137918078565647 ) ) ;
#14630=CARTESIAN_POINT ( 'NONE',  ( -3.662846001190052991, 218.4274158808045740, 28.10113791807856742 ) ) ;
#14632=CARTESIAN_POINT ( 'NONE',  ( 3.135527875058820690, 216.4958274776887492, 73.40113791807857524 ) ) ;
#14633=CARTESIAN_POINT ( 'NONE',  ( -10.00000000000000711, 207.0476921513413515, 45.50113791807857666 ) ) ;
#14636=CARTESIAN_POINT ( 'NONE',  ( -3.753561863808878130, 218.3979405102790281, 18.09886208192143187 ) ) ;
#14637=CARTESIAN_POINT ( 'NONE',  ( -3.135527875058982783, 216.4958274776886924, 21.09886208192143897 ) ) ;
#14640=CARTESIAN_POINT ( 'NONE',  ( -7.375838497908182134, 217.2372850707499765, 60.95113791807857240 ) ) ;
#14642=CARTESIAN_POINT ( 'NONE',  ( -0.05014649552807731031, 198.5883022060938572, 68.75113791807856956 ) ) ;
#14643=CARTESIAN_POINT ( 'NONE',  ( 0.05014649552828275708, 196.4853777576173002, 28.74886208192144110 ) ) ;
#14647=CARTESIAN_POINT ( 'NONE',  ( 10.00000000000000711, 206.9523078486586201, 92.00113791807858377 ) ) ;
#14649=CARTESIAN_POINT ( 'NONE',  ( -3.956728429394472002, 206.4109532238489351, -6.000000000000015099 ) ) ;
#14652=CARTESIAN_POINT ( 'NONE',  ( 6.500168698208129925, 211.6636982574063381, 34.70113791807857240 ) ) ;
#14654=CARTESIAN_POINT ( 'NONE',  ( -6.220909254589682469, 215.4770327129946850, 14.94886208192143151 ) ) ;
#14657=CARTESIAN_POINT ( 'NONE',  ( 0.05014649552807626948, 215.4116977939061144, 46.25113791807857666 ) ) ;
#14661=CARTESIAN_POINT ( 'NONE',  ( 6.139770520408223575, 215.5359834540460611, 99.54886208192144181 ) ) ;
#14663=CARTESIAN_POINT ( 'NONE',  ( -8.062137200540920645, 212.9164362838581894, 27.80113791807856671 ) ) ;
#14665=CARTESIAN_POINT ( 'NONE',  ( 8.118202686958039038, 212.8392687619912635, 16.70113791807856529 ) ) ;
#14670=CARTESIAN_POINT ( 'NONE',  ( -11.98450388067348804, 210.9467285061362247, 3.651137918078566358 ) ) ;
#14673=CARTESIAN_POINT ( 'NONE',  ( 3.044812012440130555, 197.4746971517856764, 47.60113791807857098 ) ) ;
#14679=CARTESIAN_POINT ( 'NONE',  ( -3.662846001190052991, 218.4274158808045740, 28.10113791807856742 ) ) ;
#14685=CARTESIAN_POINT ( 'NONE',  ( 6.220909254589536808, 215.4770327129947702, 1.551137918078565825 ) ) ;
#14686=CARTESIAN_POINT ( 'NONE',  ( -0.05014649552810635652, 196.4853777576173002, 56.75113791807855534 ) ) ;
#14687=CARTESIAN_POINT ( 'NONE',  ( 4.903702542908435547, 213.8346818373419751, 18.54886208192143116 ) ) ;
#14690=CARTESIAN_POINT ( 'NONE',  ( -8.015496119326531499, 204.4483345814780364, 0.3511379180785659249 ) ) ;
#14692=CARTESIAN_POINT ( 'NONE',  ( -12.01549611932659722, 210.8513442034533227, 89.64886208192142192 ) ) ;
#14698=CARTESIAN_POINT ( 'NONE',  ( -3.044812012439970683, 197.4746971517856196, 70.89886208192143613 ) ) ;
#14701=CARTESIAN_POINT ( 'NONE',  ( -8.118202686958039038, 201.1607312380087080, 6.201137918078566180 ) ) ;
#14705=CARTESIAN_POINT ( 'NONE',  ( -4.984841277089891776, 213.7757310962905990, 86.94886208192144750 ) ) ;
#14708=CARTESIAN_POINT ( 'NONE',  ( 9.736236675708031640, 199.9851607334238963, 88.29886208192142760 ) ) ;
#14710=CARTESIAN_POINT ( 'NONE',  ( -8.062137200540920645, 212.9164362838581894, 15.80113791807856849 ) ) ;
#14712=DIRECTION ( 'NONE',  ( 0.000000000000000000, -0.04769215134144316748, 0.9988620819214356628 ) ) ;
#14714=CARTESIAN_POINT ( 'NONE',  ( 7.456977232089302632, 217.1783343296989131, 85.55113791807858092 ) ) ;
#14715=CARTESIAN_POINT ( 'NONE',  ( -10.07879766094112384, 205.9536517436126530, 104.4468559609856158 ) ) ;
#14718=CARTESIAN_POINT ( 'NONE',  ( -3.753561863808878130, 218.3979405102790281, 72.09886208192142476 ) ) ;
#14719=CARTESIAN_POINT ( 'NONE',  ( 6.139770520408223575, 215.5359834540460611, 78.54886208192144181 ) ) ;
#14721=CARTESIAN_POINT ( 'NONE',  ( -11.98450388067341876, 203.0532714938636047, 11.34886208192143542 ) ) ;
#14723=CARTESIAN_POINT ( 'NONE',  ( -0.05014649552810635652, 196.4853777576173002, 35.75113791807857666 ) ) ;
#14725=CARTESIAN_POINT ( 'NONE',  ( 6.139770520408223575, 215.5359834540460611, 99.54886208192144181 ) ) ;
#14730=CARTESIAN_POINT ( 'NONE',  ( -8.000000000000008882, 206.9523078486584780, 77.49886208192144466 ) ) ;
#14736=ADVANCED_FACE ( 'NONE', ( #18852 ), #31798, .F. ) ;
#14738=CARTESIAN_POINT ( 'NONE',  ( -6.444103211791042618, 211.7408657792732356, 81.80113791807858092 ) ) ;
#14741=CARTESIAN_POINT ( 'NONE',  ( -6.500168698208244500, 211.6636982574061676, 50.79886208192144892 ) ) ;
#14748=CARTESIAN_POINT ( 'NONE',  ( 3.662846001190051659, 195.5725841191953691, 62.60113791807857808 ) ) ;
#14750=CARTESIAN_POINT ( 'NONE',  ( 3.662846001190051659, 195.5725841191953691, -0.3988620819214345747 ) ) ;
#14751=CARTESIAN_POINT ( 'NONE',  ( -9.984503880673475606, 210.2968891136704315, 81.65113791807857524 ) ) ;
#14752=CARTESIAN_POINT ( 'NONE',  ( -3.662846001189865142, 195.5725841191952838, 43.89886208192143613 ) ) ;
#14753=CARTESIAN_POINT ( 'NONE',  ( -8.062137200540822946, 201.0835637161416400, 47.19886208192143329 ) ) ;
#14755=CARTESIAN_POINT ( 'NONE',  ( -12.00000000000000711, 207.0476921513413515, 87.50113791807856956 ) ) ;
#14757=CARTESIAN_POINT ( 'NONE',  ( 9.984503880673470277, 203.7031108863295401, 5.151137918078567246 ) ) ;
#14758=CARTESIAN_POINT ( 'NONE',  ( -9.984503880673420539, 203.7031108863293980, 74.34886208192143897 ) ) ;
#14761=CARTESIAN_POINT ( 'NONE',  ( 3.753561863808876797, 195.6020594897209719, 73.59886208192142476 ) ) ;
#14765=CARTESIAN_POINT ( 'NONE',  ( 6.500168698208244500, 202.3363017425938324, 40.29886208192144181 ) ) ;
#14776=CARTESIAN_POINT ( 'NONE',  ( -8.062137200540822946, 201.0835637161416400, 38.19886208192143329 ) ) ;
#14781=CARTESIAN_POINT ( 'NONE',  ( 8.015496119326595448, 204.4483345814782638, 28.14886208192143968 ) ) ;
#14783=CARTESIAN_POINT ( 'NONE',  ( -8.118202686958039038, 201.1607312380087080, 63.20113791807857240 ) ) ;
#14784=CARTESIAN_POINT ( 'NONE',  ( 0.05014649552810505201, 217.5146222423826714, 46.25113791807855534 ) ) ;
#14786=CARTESIAN_POINT ( 'NONE',  ( -3.135527875058821579, 197.5041725223112223, 17.90113791807856458 ) ) ;
#14787=CARTESIAN_POINT ( 'NONE',  ( -2.517493886308901807, 199.4062855549015012, 5.901137918078568134 ) ) ;
#14791=CARTESIAN_POINT ( 'NONE',  ( -3.753561863808691168, 195.6020594897209435, 32.90113791807856813 ) ) ;
#14793=CARTESIAN_POINT ( 'NONE',  ( -3.135527875058821579, 197.5041725223112223, 71.90113791807857524 ) ) ;
#14794=CARTESIAN_POINT ( 'NONE',  ( 10.01549611932653860, 210.2015048109876716, 52.85113791807856387 ) ) ;
#14798=CARTESIAN_POINT ( 'NONE',  ( -12.00000000000000711, 206.9523078486584780, 14.49886208192143577 ) ) ;
#14799=CARTESIAN_POINT ( 'NONE',  ( -3.044812012439970683, 197.4746971517856196, 19.89886208192143613 ) ) ;
#14803=CARTESIAN_POINT ( 'NONE',  ( 3.662846001190051659, 195.5725841191953691, 62.60113791807857808 ) ) ;
#14804=CARTESIAN_POINT ( 'NONE',  ( 6.444103211791042618, 202.2591342207267644, 80.30113791807858092 ) ) ;
#14805=CARTESIAN_POINT ( 'NONE',  ( 6.139770520408223575, 215.5359834540460611, 30.54886208192142760 ) ) ;
#14815=CARTESIAN_POINT ( 'NONE',  ( 4.984841277089725686, 213.7757310962907411, 31.55113791807857382 ) ) ;
#14817=CARTESIAN_POINT ( 'NONE',  ( 0.05014649552828275708, 196.4853777576173002, 13.74886208192143400 ) ) ;
#14820=CARTESIAN_POINT ( 'NONE',  ( -4.903702542908602524, 213.8346818373418898, 48.95113791807857240 ) ) ;
#14824=CARTESIAN_POINT ( 'NONE',  ( -10.01549611932659722, 210.2015048109875011, 101.6488620819214361 ) ) ;
#14827=CARTESIAN_POINT ( 'NONE',  ( 8.118202686958039038, 212.8392687619912635, 31.70113791807856884 ) ) ;
#14829=CARTESIAN_POINT ( 'NONE',  ( -9.984503880673473830, 210.2968891136704315, 21.65113791807856458 ) ) ;
#14834=CARTESIAN_POINT ( 'NONE',  ( -12.00000000000000711, 207.0476921513413515, 3.501137918078566003 ) ) ;
#14837=CARTESIAN_POINT ( 'NONE',  ( 6.220909254589536808, 215.4770327129947702, 43.55113791807857382 ) ) ;
#14844=CARTESIAN_POINT ( 'NONE',  ( -7.375838497908182134, 217.2372850707499765, 30.95113791807857595 ) ) ;
#14846=CARTESIAN_POINT ( 'NONE',  ( 3.135527875058981895, 197.5041725223112792, 1.598862081921434530 ) ) ;
#14851=CARTESIAN_POINT ( 'NONE',  ( 8.062137200540920645, 201.0835637161417822, -0.6988620819214342861 ) ) ;
#14852=CARTESIAN_POINT ( 'NONE',  ( -6.220909254589537696, 198.5229672870051161, 66.05113791807858092 ) ) ;
#14854=CARTESIAN_POINT ( 'NONE',  ( -4.903702542908436435, 200.1653181626580249, 20.04886208192143471 ) ) ;
#14858=CARTESIAN_POINT ( 'NONE',  ( 2.517493886308900919, 214.5937144450984420, 1.401137918078566136 ) ) ;
#14860=CARTESIAN_POINT ( 'NONE',  ( 7.375838497908012492, 217.2372850707501186, 84.54886208192144181 ) ) ;
#14862=VERTEX_POINT ( 'NONE', #19025 ) ;
#14866=CARTESIAN_POINT ( 'NONE',  ( 10.01549611932659545, 203.7984951890123853, 70.14886208192139350 ) ) ;
#14869=CARTESIAN_POINT ( 'NONE',  ( 8.062137200540920645, 201.0835637161417822, -0.6988620819214342861 ) ) ;
#14875=CARTESIAN_POINT ( 'NONE',  ( 3.044812012440130555, 197.4746971517856764, 92.60113791807857808 ) ) ;
#14877=CARTESIAN_POINT ( 'NONE',  ( 3.044812012440130555, 197.4746971517856764, 74.60113791807856387 ) ) ;
#14880=DIRECTION ( 'NONE',  ( -0.1461455375466716444, 0.9854922318508084755, -0.08629335326029916042 ) ) ;
#14881=CARTESIAN_POINT ( 'NONE',  ( 9.680171189290716072, 214.0920067884432854, 90.69886208192143329 ) ) ;
#14884=CARTESIAN_POINT ( 'NONE',  ( -6.220909254589537696, 198.5229672870051445, 21.05113791807856671 ) ) ;
#14888=CARTESIAN_POINT ( 'NONE',  ( -12.00000000000000711, 207.0476921513413515, 84.50113791807856956 ) ) ;
#14891=CARTESIAN_POINT ( 'NONE',  ( 7.456977232089471386, 196.8216656703012006, 70.44886208192144750 ) ) ;
#14893=CARTESIAN_POINT ( 'NONE',  ( -8.062137200540822946, 201.0835637161416400, 74.19886208192143329 ) ) ;
#14894=CARTESIAN_POINT ( 'NONE',  ( -11.98450388067341876, 203.0532714938636047, 14.34886208192143364 ) ) ;
#14896=CARTESIAN_POINT ( 'NONE',  ( -10.00000000000000711, 207.0476921513413515, 36.50113791807857666 ) ) ;
#14898=CARTESIAN_POINT ( 'NONE',  ( -9.984503880673420539, 203.7031108863293980, 95.34886208192142476 ) ) ;
#14903=CARTESIAN_POINT ( 'NONE',  ( 0.05014649552828262524, 198.5883022060938572, 79.74886208192143044 ) ) ;
#14913=CARTESIAN_POINT ( 'NONE',  ( -4.903702542908602524, 213.8346818373418898, 81.95113791807858661 ) ) ;
#14918=CARTESIAN_POINT ( 'NONE',  ( 8.000000000000008882, 207.0476921513415220, 51.99886208192144466 ) ) ;
#14927=CARTESIAN_POINT ( 'NONE',  ( 11.98450388067348271, 203.0532714938637753, 59.15113791807857524 ) ) ;
#14929=CARTESIAN_POINT ( 'NONE',  ( -9.736236675707914401, 199.9851607334237542, 3.201137918078565736 ) ) ;
#14930=CARTESIAN_POINT ( 'NONE',  ( 10.01549611932653860, 210.2015048109876716, 82.85113791807856387 ) ) ;
#14931=CARTESIAN_POINT ( 'NONE',  ( 3.753561863808876797, 195.6020594897209719, 46.59886208192143187 ) ) ;
#14932=CARTESIAN_POINT ( 'NONE',  ( -8.062137200540822946, 201.0835637161416400, 44.19886208192143329 ) ) ;
#14934=CARTESIAN_POINT ( 'NONE',  ( 7.456977232089302632, 217.1783343296989131, 85.55113791807858092 ) ) ;
#14936=CARTESIAN_POINT ( 'NONE',  ( -10.01549611932653860, 203.7984951890123284, 6.351137918078566535 ) ) ;
#14937=CARTESIAN_POINT ( 'NONE',  ( -0.05014649552828403384, 217.5146222423826714, 69.24886208192144466 ) ) ;
#14940=CARTESIAN_POINT ( 'NONE',  ( -9.680171189290716072, 199.9079932115567146, 68.19886208192143329 ) ) ;
#14944=CARTESIAN_POINT ( 'NONE',  ( 4.903702542908435547, 213.8346818373419751, 48.54886208192144181 ) ) ;
#14953=CARTESIAN_POINT ( 'NONE',  ( 0.05014649552828275708, 196.4853777576173002, 43.74886208192141623 ) ) ;
#14958=CARTESIAN_POINT ( 'NONE',  ( 8.000000000000008882, 207.0476921513415220, 24.99886208192143400 ) ) ;
#14959=CARTESIAN_POINT ( 'NONE',  ( 6.139770520408368348, 198.4640165459539674, 74.45113791807857240 ) ) ;
#14961=CARTESIAN_POINT ( 'NONE',  ( -0.05014649552810635652, 196.4853777576173002, 50.75113791807856956 ) ) ;
#14962=CARTESIAN_POINT ( 'NONE',  ( -10.01549611932653860, 203.7984951890123284, 21.35113791807855677 ) ) ;
#14963=CARTESIAN_POINT ( 'NONE',  ( -8.000000000000008882, 207.0476921513413515, 6.501137918078566891 ) ) ;
#14966=CARTESIAN_POINT ( 'NONE',  ( 9.680171189290831535, 199.9079932115568852, 29.30113791807857027 ) ) ;
#14969=CARTESIAN_POINT ( 'NONE',  ( -0.05014649552810635652, 196.4853777576173002, 77.75113791807856956 ) ) ;
#14970=CARTESIAN_POINT ( 'NONE',  ( -10.00000000000000711, 207.0476921513413515, 51.50113791807857666 ) ) ;
#14974=CARTESIAN_POINT ( 'NONE',  ( 7.375838497908012492, 217.2372850707501186, 9.548862081921432932 ) ) ;
#14975=CARTESIAN_POINT ( 'NONE',  ( 6.220909254589680693, 198.5229672870052582, 22.44886208192143329 ) ) ;
#14978=CARTESIAN_POINT ( 'NONE',  ( -0.05014649552807705357, 194.3824533091408000, 56.75113791807857666 ) ) ;
#14979=CARTESIAN_POINT ( 'NONE',  ( 8.015496119326531499, 209.5516654185219636, 76.85113791807856387 ) ) ;
#14981=CARTESIAN_POINT ( 'NONE',  ( -6.220909254589682469, 215.4770327129946850, 44.94886208192143329 ) ) ;
#14990=CARTESIAN_POINT ( 'NONE',  ( -0.05014649552807731031, 198.5883022060938572, 35.75113791807857666 ) ) ;
#14992=CARTESIAN_POINT ( 'NONE',  ( -8.118202686958138514, 212.8392687619910930, 14.79886208192143648 ) ) ;
#14995=CARTESIAN_POINT ( 'NONE',  ( 8.000000000000008882, 206.9523078486586485, 59.00113791807857666 ) ) ;
#14998=CARTESIAN_POINT ( 'NONE',  ( -10.00000000000000711, 206.9523078486584495, 95.49886208192144466 ) ) ;
#15000=CARTESIAN_POINT ( 'NONE',  ( -10.01549611932653860, 203.7984951890123284, 36.35113791807857098 ) ) ;
#15002=CARTESIAN_POINT ( 'NONE',  ( 10.00000000000000711, 206.9523078486586201, 20.00113791807856600 ) ) ;
#15007=CARTESIAN_POINT ( 'NONE',  ( -7.375838497908182134, 217.2372850707499765, 3.951137918078565736 ) ) ;
#15011=CARTESIAN_POINT ( 'NONE',  ( 9.984503880673470277, 203.7031108863295401, 50.15113791807855392 ) ) ;
#15018=CARTESIAN_POINT ( 'NONE',  ( -7.456977232089304408, 196.8216656703010301, 33.05113791807856671 ) ) ;
#15021=CARTESIAN_POINT ( 'NONE',  ( -6.220909254589682469, 215.4770327129946850, 11.94886208192143684 ) ) ;
#15024=CARTESIAN_POINT ( 'NONE',  ( 3.135527875058820690, 216.4958274776887492, 4.401137918078565470 ) ) ;
#15025=CARTESIAN_POINT ( 'NONE',  ( 9.984503880673470277, 203.7031108863295401, 59.15113791807858235 ) ) ;
#15027=CARTESIAN_POINT ( 'NONE',  ( 2.517493886309087436, 199.4062855549015865, 25.59886208192143897 ) ) ;
#15029=CARTESIAN_POINT ( 'NONE',  ( -6.500168698208129925, 202.3363017425936050, 3.201137918078566624 ) ) ;
#15031=CARTESIAN_POINT ( 'NONE',  ( -11.98450388067341876, 203.0532714938636047, 92.34886208192143897 ) ) ;
#15036=CARTESIAN_POINT ( 'NONE',  ( 10.01549611932653860, 210.2015048109876716, 1.851137918078565203 ) ) ;
#15037=CARTESIAN_POINT ( 'NONE',  ( -3.135527875058982783, 216.4958274776886924, 75.09886208192143897 ) ) ;
#15040=CARTESIAN_POINT ( 'NONE',  ( -0.05014649552810635652, 196.4853777576173002, 2.751137918078565114 ) ) ;
#15044=CARTESIAN_POINT ( 'NONE',  ( 9.984503880673470277, 203.7031108863295401, 86.15113791807857524 ) ) ;
#15046=CARTESIAN_POINT ( 'NONE',  ( -3.044812012440131443, 216.5253028482142952, 73.10113791807857808 ) ) ;
#15049=CARTESIAN_POINT ( 'NONE',  ( -12.00000000000000711, 206.9523078486584780, 89.49886208192144466 ) ) ;
#15051=CARTESIAN_POINT ( 'NONE',  ( -3.044812012440131443, 216.5253028482142952, 34.10113791807857808 ) ) ;
#15055=CARTESIAN_POINT ( 'NONE',  ( -3.753561863808691168, 195.6020594897209435, 95.90113791807857524 ) ) ;
#15056=CARTESIAN_POINT ( 'NONE',  ( -10.15808088729814074, 205.9638919399499457, 104.4339049140729543 ) ) ;
#15059=CARTESIAN_POINT ( 'NONE',  ( 3.044812012439969795, 216.5253028482143520, 87.39886208192143613 ) ) ;
#15060=CARTESIAN_POINT ( 'NONE',  ( -11.98450388067341876, 203.0532714938636047, 26.34886208192143897 ) ) ;
#15062=CARTESIAN_POINT ( 'NONE',  ( 10.00000000000000711, 206.9523078486586201, 32.00113791807856956 ) ) ;
#15064=CARTESIAN_POINT ( 'NONE',  ( 10.00000000000000711, 207.0476921513415220, 99.99886208192143044 ) ) ;
#15069=CARTESIAN_POINT ( 'NONE',  ( -4.903702542908436435, 200.1653181626580249, 80.04886208192144181 ) ) ;
#15077=CARTESIAN_POINT ( 'NONE',  ( -6.500168698208129925, 202.3363017425936050, 78.20113791807857240 ) ) ;
#15083=CARTESIAN_POINT ( 'NONE',  ( 7.984503880673422316, 209.6470497212048372, 51.84886208192144608 ) ) ;
#15085=CARTESIAN_POINT ( 'NONE',  ( -10.00000000000000711, 207.0476921513413515, 3.501137918078566003 ) ) ;
#15090=CARTESIAN_POINT ( 'NONE',  ( -0.05014649552807705357, 194.3824533091408000, 62.75113791807856245 ) ) ;
#15092=CARTESIAN_POINT ( 'NONE',  ( -9.680171189290831535, 214.0920067884431148, 6.801137918078565825 ) ) ;
#15093=CARTESIAN_POINT ( 'NONE',  ( 10.00000000000000711, 206.9523078486586201, 77.00113791807858377 ) ) ;
#15094=CARTESIAN_POINT ( 'NONE',  ( -11.98450388067341876, 203.0532714938636047, 41.34886208192143187 ) ) ;
#15095=CARTESIAN_POINT ( 'NONE',  ( -6.220909254589682469, 215.4770327129947134, 53.94886208192143329 ) ) ;
#15097=CARTESIAN_POINT ( 'NONE',  ( -0.05014649552807705357, 194.3824533091408000, 89.75113791807858377 ) ) ;
#15100=CARTESIAN_POINT ( 'NONE',  ( -10.00000000000000711, 207.0476921513413515, 0.5011379180785656695 ) ) ;
#15101=CARTESIAN_POINT ( 'NONE',  ( -3.135527875058982783, 216.4958274776886924, 66.09886208192143897 ) ) ;
#15102=EDGE_CURVE ( 'NONE', #31012, #6694, #10520, .T. ) ;
#15103=AXIS2_PLACEMENT_3D ( 'NONE', #19338, #30069, #29732 ) ;
#15106=CARTESIAN_POINT ( 'NONE',  ( -3.753561863808878130, 218.3979405102790281, 69.09886208192143897 ) ) ;
#15109=CARTESIAN_POINT ( 'NONE',  ( -6.500168698208244500, 211.6636982574061676, 56.79886208192143471 ) ) ;
#15117=CARTESIAN_POINT ( 'NONE',  ( 10.01549611932659545, 203.7984951890123853, 43.14886208192142192 ) ) ;
#15123=CARTESIAN_POINT ( 'NONE',  ( -2.517493886309087880, 214.5937144450984135, 27.09886208192143897 ) ) ;
#15124=CARTESIAN_POINT ( 'NONE',  ( 6.220909254589536808, 215.4770327129947702, 70.55113791807856671 ) ) ;
#15126=CARTESIAN_POINT ( 'NONE',  ( 0.05014649552810505201, 217.5146222423826714, 52.25113791807856245 ) ) ;
#15129=CARTESIAN_POINT ( 'NONE',  ( -3.044812012440131443, 216.5253028482142952, 22.10113791807856742 ) ) ;
#15130=CARTESIAN_POINT ( 'NONE',  ( -6.444103211791042618, 211.7408657792732356, 9.801137918078564937 ) ) ;
#15133=CARTESIAN_POINT ( 'NONE',  ( -12.00000000000000711, 207.0476921513413515, 30.50113791807856600 ) ) ;
#15136=CARTESIAN_POINT ( 'NONE',  ( -9.984503880673473830, 210.2968891136704315, 75.65113791807858945 ) ) ;
#15137=CARTESIAN_POINT ( 'NONE',  ( -3.135527875058821579, 197.5041725223112223, 50.90113791807856813 ) ) ;
#15141=CARTESIAN_POINT ( 'NONE',  ( -11.98450388067341876, 203.0532714938636047, 14.34886208192143364 ) ) ;
#15142=CARTESIAN_POINT ( 'NONE',  ( -8.062137200540822946, 201.0835637161416400, 20.19886208192143684 ) ) ;
#15145=CARTESIAN_POINT ( 'NONE',  ( -12.01549611932652972, 203.1486557965464499, 57.35113791807857098 ) ) ;
#15146=CARTESIAN_POINT ( 'NONE',  ( -2.517493886308901807, 199.4062855549015012, 77.90113791807856103 ) ) ;
#15147=CARTESIAN_POINT ( 'NONE',  ( -10.00000000000000711, 206.9523078486584495, 38.49886208192143755 ) ) ;
#15150=CARTESIAN_POINT ( 'NONE',  ( 9.680171189290716072, 214.0920067884432854, 45.69886208192143329 ) ) ;
#15160=CARTESIAN_POINT ( 'NONE',  ( -6.444103211791042618, 211.7408657792732356, 27.80113791807857027 ) ) ;
#15162=CARTESIAN_POINT ( 'NONE',  ( -6.139770520408224463, 198.4640165459539389, 14.04886208192143648 ) ) ;
#15166=CARTESIAN_POINT ( 'NONE',  ( -4.903702542908602524, 213.8346818373418898, 57.95113791807855819 ) ) ;
#15169=CARTESIAN_POINT ( 'NONE',  ( 8.062137200540822946, 212.9164362838583315, 96.69886208192143329 ) ) ;
#15171=CARTESIAN_POINT ( 'NONE',  ( -6.139770520408369237, 215.5359834540460042, 45.95113791807857950 ) ) ;
#15174=CARTESIAN_POINT ( 'NONE',  ( -0.05014649552810635652, 196.4853777576173002, 20.75113791807855890 ) ) ;
#15179=CARTESIAN_POINT ( 'NONE',  ( -8.062137200540920645, 212.9164362838581894, 99.80113791807858092 ) ) ;
#15183=CARTESIAN_POINT ( 'NONE',  ( -3.135527875058821579, 197.5041725223112223, 44.90113791807857524 ) ) ;
#15191=CARTESIAN_POINT ( 'NONE',  ( 3.753561863808689836, 218.3979405102790565, 28.40113791807856813 ) ) ;
#15193=CARTESIAN_POINT ( 'NONE',  ( 8.062137200540822946, 212.9164362838583315, 12.69886208192143506 ) ) ;
#15196=CARTESIAN_POINT ( 'NONE',  ( 8.062137200540920645, 201.0835637161417822, 8.301137918078566713 ) ) ;
#15197=CARTESIAN_POINT ( 'NONE',  ( 10.01549611932653860, 210.2015048109876716, 73.85113791807857808 ) ) ;
#15199=CARTESIAN_POINT ( 'NONE',  ( 2.426778023690075337, 214.6231898156240447, 24.39886208192143258 ) ) ;
#15202=CARTESIAN_POINT ( 'NONE',  ( 6.500168698208129925, 211.6636982574063381, 7.701137918078567068 ) ) ;
#15205=CARTESIAN_POINT ( 'NONE',  ( 9.680171189290716072, 214.0920067884432854, 93.69886208192144750 ) ) ;
#15210=CARTESIAN_POINT ( 'NONE',  ( 6.139770520408368348, 198.4640165459539674, 2.451137918078566180 ) ) ;
#15211=CARTESIAN_POINT ( 'NONE',  ( -8.062137200540822946, 201.0835637161416400, 74.19886208192143329 ) ) ;
#15214=CARTESIAN_POINT ( 'NONE',  ( -3.135527875058821579, 197.5041725223112223, 14.90113791807856636 ) ) ;
#15218=CARTESIAN_POINT ( 'NONE',  ( -3.044812012440131443, 216.5253028482142952, 91.10113791807857808 ) ) ;
#15220=CARTESIAN_POINT ( 'NONE',  ( -10.00000000000000711, 207.0476921513413515, 72.50113791807858377 ) ) ;
#15224=CARTESIAN_POINT ( 'NONE',  ( -0.05014649552828442242, 219.6175466908591716, 87.24886208192144466 ) ) ;
#15226=CARTESIAN_POINT ( 'NONE',  ( 10.00000000000000711, 206.9523078486586201, 29.00113791807856956 ) ) ;
#15230=CARTESIAN_POINT ( 'NONE',  ( 7.375838497908181246, 196.7627149292499666, 98.45113791807858661 ) ) ;
#15232=CARTESIAN_POINT ( 'NONE',  ( -10.30698760260085045, 206.0014576304403136, 104.3936231590492696 ) ) ;
#15234=CARTESIAN_POINT ( 'NONE',  ( 0.05014649552828275014, 196.4853777576173002, 88.74886208192143044 ) ) ;
#15235=CARTESIAN_POINT ( 'NONE',  ( 7.456977232089471386, 196.8216656703012006, 22.44886208192143329 ) ) ;
#15237=CARTESIAN_POINT ( 'NONE',  ( 9.984503880673470277, 203.7031108863295401, 35.15113791807856813 ) ) ;
#15239=CARTESIAN_POINT ( 'NONE',  ( 0.05014649552828275708, 196.4853777576173002, 97.74886208192140202 ) ) ;
#15241=ORIENTED_EDGE ( 'NONE', *, *, #4778, .F. ) ;
#15243=CARTESIAN_POINT ( 'NONE',  ( -8.000000000000008882, 206.9523078486584780, 83.49886208192144466 ) ) ;
#15248=CARTESIAN_POINT ( 'NONE',  ( -4.984841277089726574, 200.2242689037092305, 57.05113791807856671 ) ) ;
#15251=CARTESIAN_POINT ( 'NONE',  ( -6.444103211791042618, 211.7408657792732356, 78.80113791807858092 ) ) ;
#15252=DIRECTION ( 'NONE',  ( 0.000000000000000000, 0.000000000000000000, 1.000000000000000000 ) ) ;
#15255=CARTESIAN_POINT ( 'NONE',  ( -4.984841277089891776, 213.7757310962905990, 59.94886208192144039 ) ) ;
#15257=CARTESIAN_POINT ( 'NONE',  ( 3.044812012440130555, 197.4746971517856764, 2.601137918078566091 ) ) ;
#15263=CARTESIAN_POINT ( 'NONE',  ( -0.05014649552807705357, 194.3824533091408000, 68.75113791807856956 ) ) ;
#15265=CARTESIAN_POINT ( 'NONE',  ( -7.456977232089304408, 196.8216656703010301, 12.05113791807856849 ) ) ;
#15266=CARTESIAN_POINT ( 'NONE',  ( -9.984503880673475606, 210.2968891136704315, 90.65113791807856103 ) ) ;
#15267=CARTESIAN_POINT ( 'NONE',  ( -7.456977232089471386, 217.1783343296987709, 47.94886208192143329 ) ) ;
#15268=CARTESIAN_POINT ( 'NONE',  ( 6.139770520408223575, 215.5359834540460611, 54.54886208192144181 ) ) ;
#15270=CARTESIAN_POINT ( 'NONE',  ( 9.680171189290831535, 199.9079932115568852, 98.30113791807858092 ) ) ;
#15272=CARTESIAN_POINT ( 'NONE',  ( 9.984503880673470277, 203.7031108863295401, 2.151137918078565914 ) ) ;
#15273=CARTESIAN_POINT ( 'NONE',  ( 8.062137200540822946, 212.9164362838583315, 69.69886208192144750 ) ) ;
#15276=CARTESIAN_POINT ( 'NONE',  ( 12.00000000000000711, 207.0476921513415220, 78.99886208192144466 ) ) ;
#15277=CARTESIAN_POINT ( 'NONE',  ( 6.139770520408368348, 198.4640165459539674, 86.45113791807854398 ) ) ;
#15280=CARTESIAN_POINT ( 'NONE',  ( 0.05014649552828262524, 198.5883022060938572, 49.74886208192144466 ) ) ;
#15287=CARTESIAN_POINT ( 'NONE',  ( -3.135527875058982783, 216.4958274776886924, 51.09886208192143897 ) ) ;
#15291=CARTESIAN_POINT ( 'NONE',  ( -0.05014649552828365914, 215.4116977939061144, 30.24886208192143755 ) ) ;
#15292=CARTESIAN_POINT ( 'NONE',  ( -3.135527875058821579, 197.5041725223112223, 71.90113791807857524 ) ) ;
#15295=CARTESIAN_POINT ( 'NONE',  ( 3.135527875058820690, 216.4958274776887492, 52.40113791807857524 ) ) ;
#15298=CARTESIAN_POINT ( 'NONE',  ( -6.139770520408369237, 215.5359834540460042, 24.95113791807855819 ) ) ;
#15299=CARTESIAN_POINT ( 'NONE',  ( 4.903702542908601636, 200.1653181626581102, 8.451137918078563516 ) ) ;
#15303=CARTESIAN_POINT ( 'NONE',  ( 7.456977232089302632, 217.1783343296989131, 34.55113791807856671 ) ) ;
#15305=CARTESIAN_POINT ( 'NONE',  ( -6.139770520408369237, 215.5359834540460042, 84.95113791807858661 ) ) ;
#15306=CARTESIAN_POINT ( 'NONE',  ( 8.062137200540920645, 201.0835637161417822, 62.30113791807858092 ) ) ;
#15308=CARTESIAN_POINT ( 'NONE',  ( 0.05014649552828288198, 194.3824533091408000, 13.74886208192143577 ) ) ;
#15309=CARTESIAN_POINT ( 'NONE',  ( 10.01549611932659367, 203.7984951890124421, 25.14886208192143613 ) ) ;
#15313=CARTESIAN_POINT ( 'NONE',  ( 0.05014649552807549926, 219.6175466908591716, 70.25113791807856956 ) ) ;
#15314=CARTESIAN_POINT ( 'NONE',  ( -4.903702542908602524, 213.8346818373418898, 78.95113791807858661 ) ) ;
#15315=CARTESIAN_POINT ( 'NONE',  ( 9.984503880673420539, 210.2968891136705167, 42.84886208192143897 ) ) ;
#15318=CARTESIAN_POINT ( 'NONE',  ( 12.01549611932659367, 203.1486557965466773, 40.14886208192143613 ) ) ;
#15319=ORIENTED_EDGE ( 'NONE', *, *, #18337, .T. ) ;
#15325=CARTESIAN_POINT ( 'NONE',  ( 8.000000000000008882, 206.9523078486586485, 41.00113791807857666 ) ) ;
#15327=CARTESIAN_POINT ( 'NONE',  ( 3.044812012439969795, 216.5253028482143520, 27.39886208192143613 ) ) ;
#15330=CARTESIAN_POINT ( 'NONE',  ( -8.000000000000008882, 207.0476921513413515, 57.50113791807857666 ) ) ;
#15335=CARTESIAN_POINT ( 'NONE',  ( -6.139770520408224463, 198.4640165459539389, 98.04886208192141339 ) ) ;
#15336=CARTESIAN_POINT ( 'NONE',  ( -3.044812012440131443, 216.5253028482142952, 43.10113791807857808 ) ) ;
#15338=EDGE_CURVE ( 'NONE', #18219, #28735, #10904, .T. ) ;
#15339=CARTESIAN_POINT ( 'NONE',  ( -6.220909254589537696, 198.5229672870051161, 24.05113791807855961 ) ) ;
#15342=CARTESIAN_POINT ( 'NONE',  ( -2.426778023690076225, 199.3768101843759553, 82.89886208192143613 ) ) ;
#15347=CARTESIAN_POINT ( 'NONE',  ( 12.00000000000000711, 206.9523078486586485, 5.001137918078565114 ) ) ;
#15351=CARTESIAN_POINT ( 'NONE',  ( 6.220909254589536808, 215.4770327129947702, 58.55113791807858092 ) ) ;
#15355=CARTESIAN_POINT ( 'NONE',  ( -3.135527875058982783, 216.4958274776886924, 3.098862081921434974 ) ) ;
#15358=CARTESIAN_POINT ( 'NONE',  ( -12.01549611932652972, 203.1486557965464499, 27.35113791807856742 ) ) ;
#15360=CARTESIAN_POINT ( 'NONE',  ( 3.044812012439969795, 216.5253028482143520, 15.39886208192143613 ) ) ;
#15363=CARTESIAN_POINT ( 'NONE',  ( -10.00000000000000711, 207.0476921513413515, 12.50113791807856778 ) ) ;
#15364=CARTESIAN_POINT ( 'NONE',  ( -10.00000000000000711, 207.0476921513413515, 72.50113791807858377 ) ) ;
#15367=CARTESIAN_POINT ( 'NONE',  ( 6.500168698208244500, 202.3363017425938324, 31.29886208192143826 ) ) ;
#15370=CARTESIAN_POINT ( 'NONE',  ( -8.015496119326531499, 204.4483345814780364, 3.351137918078566535 ) ) ;
#15373=CARTESIAN_POINT ( 'NONE',  ( 12.00000000000000711, 207.0476921513415220, 84.99886208192144466 ) ) ;
#15378=CARTESIAN_POINT ( 'NONE',  ( -10.01549611932653860, 203.7984951890123284, 6.351137918078566535 ) ) ;
#15379=CARTESIAN_POINT ( 'NONE',  ( -0.05014649552828403384, 217.5146222423826714, 69.24886208192144466 ) ) ;
#15382=CARTESIAN_POINT ( 'NONE',  ( -10.00000000000000711, 207.0476921513413515, 9.501137918078566003 ) ) ;
#15386=CARTESIAN_POINT ( 'NONE',  ( 6.139770520408368348, 198.4640165459539674, 101.4511379180785866 ) ) ;
#15388=CARTESIAN_POINT ( 'NONE',  ( -0.05014649552810635652, 196.4853777576173002, 71.75113791807858377 ) ) ;
#15391=CARTESIAN_POINT ( 'NONE',  ( -0.05014649552828442242, 219.6175466908591716, 90.24886208192144466 ) ) ;
#15397=CARTESIAN_POINT ( 'NONE',  ( -7.375838497908182134, 217.2372850707499765, 99.95113791807860082 ) ) ;
#15400=CARTESIAN_POINT ( 'NONE',  ( -11.00000000000000711, 206.8801259629684921, 103.6040119011138358 ) ) ;
#15402=CARTESIAN_POINT ( 'NONE',  ( -3.135527875058982783, 216.4958274776886924, 84.09886208192143897 ) ) ;
#15403=CARTESIAN_POINT ( 'NONE',  ( 9.680171189290716072, 214.0920067884432854, 18.69886208192143684 ) ) ;
#15405=CARTESIAN_POINT ( 'NONE',  ( 9.984503880673470277, 203.7031108863295401, 44.15113791807856813 ) ) ;
#15408=CARTESIAN_POINT ( 'NONE',  ( -3.135527875058982783, 216.4958274776886924, 96.09886208192143897 ) ) ;
#15412=CARTESIAN_POINT ( 'NONE',  ( 4.903702542908435547, 213.8346818373419751, 81.54886208192144181 ) ) ;
#15418=CARTESIAN_POINT ( 'NONE',  ( 2.517493886308900919, 214.5937144450984420, 58.40113791807858235 ) ) ;
#15422=CARTESIAN_POINT ( 'NONE',  ( 4.984841277089725686, 213.7757310962907411, 85.55113791807858092 ) ) ;
#15426=CARTESIAN_POINT ( 'NONE',  ( -6.444103211790928043, 202.2591342207265939, 65.19886208192143329 ) ) ;
#15430=CARTESIAN_POINT ( 'NONE',  ( 8.118202686958039038, 212.8392687619912635, 1.701137918078565736 ) ) ;
#15431=CARTESIAN_POINT ( 'NONE',  ( 8.640141755188686545, 206.6086104956403915, 111.6972426105882477 ) ) ;
#15434=CARTESIAN_POINT ( 'NONE',  ( 9.680171189290831535, 199.9079932115568852, 68.30113791807856671 ) ) ;
#15437=CARTESIAN_POINT ( 'NONE',  ( 3.662846001190051659, 195.5725841191953691, 14.60113791807856742 ) ) ;
#15439=CARTESIAN_POINT ( 'NONE',  ( -0.05014649552810635652, 196.4853777576173002, 89.75113791807856956 ) ) ;
#15440=CARTESIAN_POINT ( 'NONE',  ( -7.375838497908014268, 196.7627149292498530, 50.04886208192142760 ) ) ;
#15441=CARTESIAN_POINT ( 'NONE',  ( -10.01549611932659545, 210.2015048109875011, 56.64886208192143613 ) ) ;
#15443=CARTESIAN_POINT ( 'NONE',  ( -11.98450388067348804, 210.9467285061362247, 93.65113791807857524 ) ) ;
#15445=CARTESIAN_POINT ( 'NONE',  ( 0.05014649552810505201, 217.5146222423826714, 16.25113791807856600 ) ) ;
#15448=CARTESIAN_POINT ( 'NONE',  ( -8.118202686958138514, 212.8392687619910930, 71.79886208192142760 ) ) ;
#15451=CARTESIAN_POINT ( 'NONE',  ( -12.01549611932659722, 210.8513442034533227, 80.64886208192145034 ) ) ;
#15452=CARTESIAN_POINT ( 'NONE',  ( 10.01549611932653860, 210.2015048109876716, 88.85113791807857808 ) ) ;
#15455=CARTESIAN_POINT ( 'NONE',  ( -8.000000000000008882, 206.9523078486584780, 47.49886208192144466 ) ) ;
#15463=CARTESIAN_POINT ( 'NONE',  ( -10.01549611932659722, 210.2015048109875011, 53.64886208192141481 ) ) ;
#15464=EDGE_LOOP ( 'NONE', ( #9618, #924 ) ) ;
#15469=CARTESIAN_POINT ( 'NONE',  ( 2.426778023690075337, 214.6231898156240447, 30.39886208192143613 ) ) ;
#15471=CARTESIAN_POINT ( 'NONE',  ( 10.01549611932653860, 210.2015048109876716, 73.85113791807857808 ) ) ;
#15473=CARTESIAN_POINT ( 'NONE',  ( -8.062137200540920645, 212.9164362838581894, 60.80113791807857382 ) ) ;
#15474=CARTESIAN_POINT ( 'NONE',  ( -6.220909254589537696, 198.5229672870051161, 24.05113791807855961 ) ) ;
#15475=CARTESIAN_POINT ( 'NONE',  ( 0.05014649552807626948, 215.4116977939061144, 16.25113791807856600 ) ) ;
#15479=CARTESIAN_POINT ( 'NONE',  ( 0.05014649552807549926, 219.6175466908591716, 37.25113791807857666 ) ) ;
#15481=CARTESIAN_POINT ( 'NONE',  ( 3.135527875058820690, 216.4958274776887492, 85.40113791807857524 ) ) ;
#15482=CARTESIAN_POINT ( 'NONE',  ( -9.984503880673475606, 210.2968891136704315, 63.65113791807856813 ) ) ;
#15484=STYLED_ITEM ( 'NONE', ( #1666 ), #21009 ) ;
#15485=CARTESIAN_POINT ( 'NONE',  ( -11.98450388067341876, 203.0532714938636047, 20.34886208192143542 ) ) ;
#15486=CARTESIAN_POINT ( 'NONE',  ( -10.01549611932659545, 210.2015048109875011, 29.64886208192143968 ) ) ;
#15488=CARTESIAN_POINT ( 'NONE',  ( 7.456977232089302632, 217.1783343296989131, 64.55113791807856671 ) ) ;
#15489=CARTESIAN_POINT ( 'NONE',  ( 7.984503880673485376, 204.3529502787953902, 77.15113791807857524 ) ) ;
#15490=CARTESIAN_POINT ( 'NONE',  ( 10.00000000000000711, 207.0476921513415220, 39.99886208192143755 ) ) ;
#15493=CARTESIAN_POINT ( 'NONE',  ( -0.05014649552828442242, 219.6175466908591716, 54.24886208192143755 ) ) ;
#15499=CARTESIAN_POINT ( 'NONE',  ( 6.444103211791042618, 202.2591342207267644, 41.30113791807857382 ) ) ;
#15502=CARTESIAN_POINT ( 'NONE',  ( 10.01549611932659545, 203.7984951890123853, 22.14886208192143613 ) ) ;
#15507=CARTESIAN_POINT ( 'NONE',  ( -0.05014649552828365914, 215.4116977939061144, 6.248862081921434886 ) ) ;
#15508=CARTESIAN_POINT ( 'NONE',  ( 9.984503880673470277, 203.7031108863295401, 44.15113791807856813 ) ) ;
#15509=CARTESIAN_POINT ( 'NONE',  ( 0.05014649552810505201, 217.5146222423826714, 25.25113791807856245 ) ) ;
#15510=FACE_OUTER_BOUND ( 'NONE', #5974, .T. ) ;
#15511=CARTESIAN_POINT ( 'NONE',  ( -0.05014649552828365914, 215.4116977939061144, 96.24886208192144466 ) ) ;
#15515=CARTESIAN_POINT ( 'NONE',  ( -7.456977232089304408, 196.8216656703010301, 9.051137918078564937 ) ) ;
#15518=CARTESIAN_POINT ( 'NONE',  ( 8.062137200540920645, 201.0835637161417822, 53.30113791807857382 ) ) ;
#15524=CARTESIAN_POINT ( 'NONE',  ( 12.00000000000000711, 206.9523078486586485, 41.00113791807856245 ) ) ;
#15526=CARTESIAN_POINT ( 'NONE',  ( 0.05014649552828275708, 196.4853777576173002, 16.74886208192143755 ) ) ;
#15530=CARTESIAN_POINT ( 'NONE',  ( 8.118202686958039038, 212.8392687619912635, 7.701137918078566180 ) ) ;
#15531=CARTESIAN_POINT ( 'NONE',  ( -3.044812012440131443, 216.5253028482142952, 67.10113791807857808 ) ) ;
#15533=CARTESIAN_POINT ( 'NONE',  ( -4.984841277089891776, 213.7757310962905990, 29.94886208192143684 ) ) ;
#15537=CARTESIAN_POINT ( 'NONE',  ( -6.500168698208129925, 202.3363017425936050, 9.201137918078563516 ) ) ;
#15538=CARTESIAN_POINT ( 'NONE',  ( 9.680171189290716072, 214.0920067884432854, 102.6988620819214475 ) ) ;
#15543=CARTESIAN_POINT ( 'NONE',  ( 3.044812012440130555, 197.4746971517856764, 11.60113791807856742 ) ) ;
#15544=CARTESIAN_POINT ( 'NONE',  ( -3.044812012439970683, 197.4746971517856196, 82.89886208192145034 ) ) ;
#15547=CARTESIAN_POINT ( 'NONE',  ( -6.139770520408369237, 215.5359834540460042, 12.95113791807856352 ) ) ;
#15550=CARTESIAN_POINT ( 'NONE',  ( 6.220909254589536808, 215.4770327129947702, 97.55113791807855250 ) ) ;
#15552=CARTESIAN_POINT ( 'NONE',  ( -3.135527875058821579, 197.5041725223112223, 80.90113791807858945 ) ) ;
#15554=CARTESIAN_POINT ( 'NONE',  ( 3.662846001189864698, 218.4274158808046593, 96.39886208192146455 ) ) ;
#15559=CARTESIAN_POINT ( 'NONE',  ( -7.456977232089304408, 196.8216656703010301, 93.05113791807858092 ) ) ;
#15563=CARTESIAN_POINT ( 'NONE',  ( 8.062137200540822946, 212.9164362838583315, 90.69886208192143329 ) ) ;
#15564=CARTESIAN_POINT ( 'NONE',  ( -7.456977232089471386, 217.1783343296987709, 20.94886208192143684 ) ) ;
#15566=CARTESIAN_POINT ( 'NONE',  ( -10.00000000000000711, 207.0476921513413515, 39.50113791807856956 ) ) ;
#15568=CARTESIAN_POINT ( 'NONE',  ( 2.517493886309087436, 199.4062855549015865, 1.598862081921434974 ) ) ;
#15572=CARTESIAN_POINT ( 'NONE',  ( -8.000000000000008882, 206.9523078486584780, 89.49886208192144466 ) ) ;
#15573=ORIENTED_EDGE ( 'NONE', *, *, #6230, .F. ) ;
#15574=CARTESIAN_POINT ( 'NONE',  ( -4.903702542908602524, 213.8346818373418898, 30.95113791807857595 ) ) ;
#15580=CARTESIAN_POINT ( 'NONE',  ( -6.444103211791042618, 211.7408657792732356, 90.80113791807858092 ) ) ;
#15584=CARTESIAN_POINT ( 'NONE',  ( 6.500168698208244500, 202.3363017425938324, 64.29886208192144181 ) ) ;
#15586=EDGE_CURVE ( 'NONE', #28270, #16107, #4254, .T. ) ;
#15590=CARTESIAN_POINT ( 'NONE',  ( -6.220909254589537696, 198.5229672870051445, 0.05113791807856578331 ) ) ;
#15591=DIRECTION ( 'NONE',  ( -0.3500148194780949296, -0.04467534437043436946, 0.9356782244720136532 ) ) ;
#15594=CARTESIAN_POINT ( 'NONE',  ( 7.375838497908181246, 196.7627149292499666, 68.45113791807857240 ) ) ;
#15596=CARTESIAN_POINT ( 'NONE',  ( 0.05014649552807549926, 219.6175466908591716, 10.25113791807856600 ) ) ;
#15597=CARTESIAN_POINT ( 'NONE',  ( -6.220909254589537696, 198.5229672870051445, 84.05113791807856671 ) ) ;
#15599=CARTESIAN_POINT ( 'NONE',  ( 7.375838497908012492, 217.2372850707501186, 54.54886208192142760 ) ) ;
#15600=CARTESIAN_POINT ( 'NONE',  ( -6.220909254589682469, 215.4770327129947134, 59.94886208192142618 ) ) ;
#15601=CARTESIAN_POINT ( 'NONE',  ( -7.456977232089304408, 196.8216656703010301, 93.05113791807858092 ) ) ;
#15603=CARTESIAN_POINT ( 'NONE',  ( 8.062137200540920645, 201.0835637161417822, 11.30113791807856671 ) ) ;
#15604=CARTESIAN_POINT ( 'NONE',  ( -10.01549611932659722, 210.2015048109875011, 74.64886208192142192 ) ) ;
#15606=CARTESIAN_POINT ( 'NONE',  ( -7.456977232089471386, 217.1783343296987709, 77.94886208192143329 ) ) ;
#15607=CARTESIAN_POINT ( 'NONE',  ( 3.044812012440130555, 197.4746971517856764, 98.60113791807857808 ) ) ;
#15610=CARTESIAN_POINT ( 'NONE',  ( 2.517493886309087436, 199.4062855549015865, 55.59886208192143897 ) ) ;
#15622=CARTESIAN_POINT ( 'NONE',  ( 3.044812012439969795, 216.5253028482143520, 48.39886208192143613 ) ) ;
#15627=CARTESIAN_POINT ( 'NONE',  ( -8.000000000000008882, 206.9523078486584780, 35.49886208192143044 ) ) ;
#15628=CARTESIAN_POINT ( 'NONE',  ( -3.135527875058821579, 197.5041725223112223, 74.90113791807857524 ) ) ;
#15631=CARTESIAN_POINT ( 'NONE',  ( 3.044812012440130555, 197.4746971517856764, 59.60113791807857808 ) ) ;
#15632=CARTESIAN_POINT ( 'NONE',  ( 3.044812012440130555, 197.4746971517856764, 26.60113791807856742 ) ) ;
#15633=CARTESIAN_POINT ( 'NONE',  ( -4.903702542908602524, 213.8346818373418898, 12.95113791807856707 ) ) ;
#15637=CARTESIAN_POINT ( 'NONE',  ( -0.05014649552807705357, 194.3824533091408000, 38.75113791807856245 ) ) ;
#15641=CARTESIAN_POINT ( 'NONE',  ( -0.05014649552810635652, 196.4853777576173002, 89.75113791807854113 ) ) ;
#15642=CARTESIAN_POINT ( 'NONE',  ( 3.135527875058820690, 216.4958274776887492, 58.40113791807857524 ) ) ;
#15646=CARTESIAN_POINT ( 'NONE',  ( 9.680171189290716072, 214.0920067884432854, 27.69886208192143684 ) ) ;
#15648=CARTESIAN_POINT ( 'NONE',  ( -0.05014649552828402690, 217.5146222423826714, 27.24886208192143400 ) ) ;
#15650=CARTESIAN_POINT ( 'NONE',  ( -0.05014649552807705357, 194.3824533091408000, 68.75113791807856956 ) ) ;
#15651=CARTESIAN_POINT ( 'NONE',  ( -2.517493886308901807, 199.4062855549015012, 89.90113791807857524 ) ) ;
#15652=CARTESIAN_POINT ( 'NONE',  ( -3.044812012439970683, 197.4746971517856196, 46.89886208192143613 ) ) ;
#15656=CARTESIAN_POINT ( 'NONE',  ( 7.375838497908012492, 217.2372850707501186, 54.54886208192142760 ) ) ;
#15662=CARTESIAN_POINT ( 'NONE',  ( -4.903702542908602524, 213.8346818373418898, 45.95113791807857950 ) ) ;
#15665=CARTESIAN_POINT ( 'NONE',  ( 0.05014649552828275708, 196.4853777576173002, 22.74886208192142689 ) ) ;
#15671=CARTESIAN_POINT ( 'NONE',  ( -8.015496119326597224, 209.5516654185217362, 2.648862081921435241 ) ) ;
#15672=CARTESIAN_POINT ( 'NONE',  ( -3.044812012440131443, 216.5253028482142952, 40.10113791807857098 ) ) ;
#15674=CARTESIAN_POINT ( 'NONE',  ( -8.062137200540920645, 212.9164362838581894, 30.80113791807856671 ) ) ;
#15678=CARTESIAN_POINT ( 'NONE',  ( 0.05014649552828262524, 198.5883022060938572, 91.74886208192144466 ) ) ;
#15682=CARTESIAN_POINT ( 'NONE',  ( 3.662846001190051659, 195.5725841191953691, 14.60113791807856742 ) ) ;
#15685=CARTESIAN_POINT ( 'NONE',  ( 0.05014649552810505201, 217.5146222423826714, 55.25113791807858377 ) ) ;
#15690=CARTESIAN_POINT ( 'NONE',  ( 12.00000000000000711, 206.9523078486586485, 35.00113791807857666 ) ) ;
#15692=CARTESIAN_POINT ( 'NONE',  ( -10.01549611932659722, 210.2015048109875011, 11.64886208192143258 ) ) ;
#15697=CARTESIAN_POINT ( 'NONE',  ( 8.062137200540920645, 201.0835637161417822, 74.30113791807858092 ) ) ;
#15699=CARTESIAN_POINT ( 'NONE',  ( 8.000000000000008882, 207.0476921513415220, 36.99886208192143044 ) ) ;
#15703=CARTESIAN_POINT ( 'NONE',  ( 6.444103211791042618, 202.2591342207267644, 14.30113791807856849 ) ) ;
#15704=CARTESIAN_POINT ( 'NONE',  ( -7.456977232089471386, 217.1783343296987709, 101.9488620819214475 ) ) ;
#15709=CARTESIAN_POINT ( 'NONE',  ( -6.220909254589537696, 198.5229672870051161, 12.05113791807856671 ) ) ;
#15711=CARTESIAN_POINT ( 'NONE',  ( -3.135527875058982783, 216.4958274776886924, 81.09886208192143897 ) ) ;
#15714=CARTESIAN_POINT ( 'NONE',  ( 6.139770520408368348, 198.4640165459539674, 14.45113791807856352 ) ) ;
#15717=CARTESIAN_POINT ( 'NONE',  ( 9.680171189290831535, 199.9079932115568852, 38.30113791807856671 ) ) ;
#15719=CARTESIAN_POINT ( 'NONE',  ( -6.139770520408369237, 215.5359834540460042, 99.95113791807855819 ) ) ;
#15721=CARTESIAN_POINT ( 'NONE',  ( 0.05014649552810505201, 217.5146222423826714, 88.25113791807858377 ) ) ;
#15724=CARTESIAN_POINT ( 'NONE',  ( -11.98450388067341876, 203.0532714938636047, 101.3488620819214390 ) ) ;
#15731=CARTESIAN_POINT ( 'NONE',  ( -9.736236675707914401, 199.9851607334237542, 96.20113791807858661 ) ) ;
#15734=CARTESIAN_POINT ( 'NONE',  ( -9.984503880673420539, 203.7031108863293980, 89.34886208192143897 ) ) ;
#15735=CARTESIAN_POINT ( 'NONE',  ( 3.662846001189864698, 218.4274158808046593, 21.39886208192143613 ) ) ;
#15738=CARTESIAN_POINT ( 'NONE',  ( -3.135527875058821579, 197.5041725223112223, 38.90113791807857524 ) ) ;
#15741=CARTESIAN_POINT ( 'NONE',  ( 8.000000000000008882, 207.0476921513415220, 6.998862081921435774 ) ) ;
#15744=CARTESIAN_POINT ( 'NONE',  ( -8.015496119326597224, 209.5516654185217362, 92.64886208192143613 ) ) ;
#15746=CARTESIAN_POINT ( 'NONE',  ( 8.000000000000008882, 206.9523078486586485, 26.00113791807856600 ) ) ;
#15752=CARTESIAN_POINT ( 'NONE',  ( 0.05014649552807626948, 215.4116977939061144, 91.25113791807856956 ) ) ;
#15755=CARTESIAN_POINT ( 'NONE',  ( -4.903702542908436435, 200.1653181626580249, 65.04886208192144181 ) ) ;
#15760=CARTESIAN_POINT ( 'NONE',  ( 9.984503880673473830, 203.7031108863295401, -0.8488620819214343083 ) ) ;
#15764=CARTESIAN_POINT ( 'NONE',  ( 12.01549611932652972, 210.8513442034534933, 64.85113791807857808 ) ) ;
#15766=CARTESIAN_POINT ( 'NONE',  ( 3.135527875058820690, 216.4958274776887492, 91.40113791807857524 ) ) ;
#15769=CARTESIAN_POINT ( 'NONE',  ( 9.680171189290716072, 214.0920067884432854, 54.69886208192144039 ) ) ;
#15770=CARTESIAN_POINT ( 'NONE',  ( 10.00000000000000711, 207.0476921513415220, 54.99886208192143755 ) ) ;
#15771=CARTESIAN_POINT ( 'NONE',  ( 0.05014649552807549926, 219.6175466908591716, 97.25113791807856956 ) ) ;
#15773=CARTESIAN_POINT ( 'NONE',  ( 3.135527875058820690, 216.4958274776887492, 13.40113791807856636 ) ) ;
#15774=CARTESIAN_POINT ( 'NONE',  ( 8.062137200540822946, 212.9164362838583315, 75.69886208192143329 ) ) ;
#15776=CARTESIAN_POINT ( 'NONE',  ( -12.01549611932659722, 210.8513442034533227, 77.64886208192143613 ) ) ;
#15777=CARTESIAN_POINT ( 'NONE',  ( -8.118202686958039038, 201.1607312380087080, 99.20113791807858661 ) ) ;
#15779=CARTESIAN_POINT ( 'NONE',  ( -4.984841277089891776, 213.7757310962905990, 65.94886208192144750 ) ) ;
#15790=CARTESIAN_POINT ( 'NONE',  ( 8.118202686958138514, 201.1607312380088501, 52.29886208192143471 ) ) ;
#15795=CARTESIAN_POINT ( 'NONE',  ( 0.05014649552828262524, 198.5883022060938572, 37.74886208192143755 ) ) ;
#15796=CARTESIAN_POINT ( 'NONE',  ( -3.135527875058821579, 197.5041725223112223, 77.90113791807857524 ) ) ;
#15798=CARTESIAN_POINT ( 'NONE',  ( -3.135527875058821579, 197.5041725223112223, 53.90113791807857524 ) ) ;
#15799=CARTESIAN_POINT ( 'NONE',  ( 10.00000000000000711, 206.9523078486586201, 23.00113791807856600 ) ) ;
#15800=CARTESIAN_POINT ( 'NONE',  ( 2.426778023690261410, 199.3768101843759837, 14.60113791807856742 ) ) ;
#15804=CARTESIAN_POINT ( 'NONE',  ( 9.736236675707914401, 214.0148392665762458, 40.70113791807857240 ) ) ;
#15806=CARTESIAN_POINT ( 'NONE',  ( -0.05014649552810635652, 196.4853777576173002, 86.75113791807858377 ) ) ;
#15807=CARTESIAN_POINT ( 'NONE',  ( -9.984503880673475606, 210.2968891136704315, 57.65113791807857524 ) ) ;
#15808=CARTESIAN_POINT ( 'NONE',  ( -3.662846001189865142, 195.5725841191952838, 22.89886208192143613 ) ) ;
#15809=CARTESIAN_POINT ( 'NONE',  ( -3.135527875058982783, 216.4958274776886924, 27.09886208192143542 ) ) ;
#15811=CARTESIAN_POINT ( 'NONE',  ( -9.680171189290831535, 214.0920067884431148, 66.80113791807858092 ) ) ;
#15812=CARTESIAN_POINT ( 'NONE',  ( 8.015496119326531499, 209.5516654185219636, 88.85113791807857808 ) ) ;
#15814=CARTESIAN_POINT ( 'NONE',  ( 10.01549611932659545, 203.7984951890123853, 46.14886208192143613 ) ) ;
#15819=CARTESIAN_POINT ( 'NONE',  ( -12.01549611932659722, 210.8513442034533227, 56.64886208192142902 ) ) ;
#15826=CARTESIAN_POINT ( 'NONE',  ( -6.500168698208129925, 202.3363017425936050, 39.20113791807857240 ) ) ;
#15829=CARTESIAN_POINT ( 'NONE',  ( -6.220909254589682469, 215.4770327129946850, 23.94886208192142618 ) ) ;
#15832=DIRECTION ( 'NONE',  ( -0.9998603841633338929, 0.01669062914075312987, 0.0007969188393214247284 ) ) ;
#15835=CARTESIAN_POINT ( 'NONE',  ( 7.984503880673422316, 209.6470497212048372, 9.848862081921433642 ) ) ;
#15836=CARTESIAN_POINT ( 'NONE',  ( 8.062137200540920645, 201.0835637161417822, 44.30113791807857382 ) ) ;
#15838=CARTESIAN_POINT ( 'NONE',  ( 8.118202686958039038, 212.8392687619912635, 28.70113791807856884 ) ) ;
#15839=CARTESIAN_POINT ( 'NONE',  ( -0.05014649552828402690, 217.5146222423826714, 102.2488620819214304 ) ) ;
#15842=CARTESIAN_POINT ( 'NONE',  ( -4.984841277089891776, 213.7757310962905990, 89.94886208192144750 ) ) ;
#15846=CARTESIAN_POINT ( 'NONE',  ( -7.456977232089304408, 196.8216656703010301, 6.051137918078566713 ) ) ;
#15849=CARTESIAN_POINT ( 'NONE',  ( 9.984503880673470277, 203.7031108863295401, 56.15113791807856103 ) ) ;
#15850=CARTESIAN_POINT ( 'NONE',  ( 8.118202686958039038, 212.8392687619912635, 31.70113791807856884 ) ) ;
#15856=CARTESIAN_POINT ( 'NONE',  ( -9.736236675707914401, 199.9851607334237542, 36.20113791807856529 ) ) ;
#15859=CARTESIAN_POINT ( 'NONE',  ( -3.044812012439970683, 197.4746971517856196, 16.89886208192143613 ) ) ;
#15863=CARTESIAN_POINT ( 'NONE',  ( -10.01549611932653860, 203.7984951890123284, 66.35113791807853545 ) ) ;
#15865=DIRECTION ( 'NONE',  ( -0.1461455375466716444, 0.9854922318508084755, -0.08629335326029916042 ) ) ;
#15868=CARTESIAN_POINT ( 'NONE',  ( -4.903702542908602524, 213.8346818373418898, 9.951137918078567068 ) ) ;
#15870=CARTESIAN_POINT ( 'NONE',  ( -11.98450388067341876, 203.0532714938636047, 98.34886208192145318 ) ) ;
#15875=CARTESIAN_POINT ( 'NONE',  ( 3.135527875058820690, 216.4958274776887492, 4.401137918078565470 ) ) ;
#15877=CARTESIAN_POINT ( 'NONE',  ( -8.118202686958138514, 212.8392687619910930, 80.79886208192144181 ) ) ;
#15880=CARTESIAN_POINT ( 'NONE',  ( -6.139770520408369237, 215.5359834540460042, 15.95113791807856884 ) ) ;
#15885=CARTESIAN_POINT ( 'NONE',  ( -6.220909254589537696, 198.5229672870051161, 81.05113791807856671 ) ) ;
#15888=CARTESIAN_POINT ( 'NONE',  ( -12.00000000000000711, 206.9523078486584780, 98.49886208192143044 ) ) ;
#15893=CARTESIAN_POINT ( 'NONE',  ( -9.680171189290716072, 199.9079932115567146, 5.198862081921434175 ) ) ;
#15896=CARTESIAN_POINT ( 'NONE',  ( 10.00000000000000711, 207.0476921513415220, 96.99886208192143044 ) ) ;
#15897=AXIS2_PLACEMENT_3D ( 'NONE', #8632, #13577, #800 ) ;
#15898=CARTESIAN_POINT ( 'NONE',  ( -12.01549611932659722, 210.8513442034533227, 35.64886208192142902 ) ) ;
#15900=CARTESIAN_POINT ( 'NONE',  ( -3.044812012440131443, 216.5253028482142952, 43.10113791807857808 ) ) ;
#15902=CARTESIAN_POINT ( 'NONE',  ( -6.444103211790928043, 202.2591342207265939, 2.198862081921435063 ) ) ;
#15905=CARTESIAN_POINT ( 'NONE',  ( -4.984841277089891776, 213.7757310962905990, 86.94886208192144750 ) ) ;
#15907=CARTESIAN_POINT ( 'NONE',  ( 4.903702542908601636, 200.1653181626581102, 29.45113791807856529 ) ) ;
#15914=CARTESIAN_POINT ( 'NONE',  ( 2.426778023690261410, 199.3768101843759837, 83.60113791807857808 ) ) ;
#15918=CARTESIAN_POINT ( 'NONE',  ( -0.05014649552828365914, 215.4116977939061144, 66.24886208192143044 ) ) ;
#15922=CARTESIAN_POINT ( 'NONE',  ( -0.05014649552810635652, 196.4853777576173002, 14.75113791807856423 ) ) ;
#15927=CARTESIAN_POINT ( 'NONE',  ( -12.01549611932652972, 203.1486557965464499, 72.35113791807857808 ) ) ;
#15929=CARTESIAN_POINT ( 'NONE',  ( 6.220909254589536808, 215.4770327129947987, 91.55113791807858092 ) ) ;
#15930=FACE_OUTER_BOUND ( 'NONE', #32324, .T. ) ;
#15932=CARTESIAN_POINT ( 'NONE',  ( -7.456977232089471386, 217.1783343296987709, 53.94886208192144039 ) ) ;
#15934=CARTESIAN_POINT ( 'NONE',  ( 8.062137200540822946, 212.9164362838583315, 66.69886208192143329 ) ) ;
#15935=CARTESIAN_POINT ( 'NONE',  ( 3.753561863808689836, 218.3979405102790565, 97.40113791807858945 ) ) ;
#15938=CARTESIAN_POINT ( 'NONE',  ( 9.984503880673470277, 203.7031108863295401, 17.15113791807856103 ) ) ;
#15939=CARTESIAN_POINT ( 'NONE',  ( -6.220909254589682469, 215.4770327129946850, 80.94886208192143329 ) ) ;
#15942=CARTESIAN_POINT ( 'NONE',  ( 10.01549611932653860, 210.2015048109876716, 100.8511379180785497 ) ) ;
#15946=CARTESIAN_POINT ( 'NONE',  ( -6.500168698208244500, 211.6636982574061676, 62.79886208192144892 ) ) ;
#15954=CARTESIAN_POINT ( 'NONE',  ( 2.517493886308900919, 214.5937144450984420, 58.40113791807858235 ) ) ;
#15962=CARTESIAN_POINT ( 'NONE',  ( 2.517493886309087436, 199.4062855549015865, 37.59886208192143187 ) ) ;
#15963=CARTESIAN_POINT ( 'NONE',  ( 10.00000000000000711, 206.9523078486586201, 83.00113791807856956 ) ) ;
#15965=CARTESIAN_POINT ( 'NONE',  ( -6.220909254589537696, 198.5229672870051161, 66.05113791807858092 ) ) ;
#15966=CARTESIAN_POINT ( 'NONE',  ( -3.135527875058821579, 197.5041725223112223, 26.90113791807856813 ) ) ;
#15967=CARTESIAN_POINT ( 'NONE',  ( -0.05014649552807731031, 198.5883022060938572, 17.75113791807856956 ) ) ;
#15972=CARTESIAN_POINT ( 'NONE',  ( 12.00000000000000711, 206.9523078486586485, 38.00113791807857666 ) ) ;
#15973=CARTESIAN_POINT ( 'NONE',  ( -0.3755270751584372513, 206.7692714347155629, 108.3323677711371573 ) ) ;
#15975=CARTESIAN_POINT ( 'NONE',  ( -8.062137200540920645, 212.9164362838581894, 84.80113791807856671 ) ) ;
#15976=CARTESIAN_POINT ( 'NONE',  ( -3.044812012440131443, 216.5253028482142952, 58.10113791807857808 ) ) ;
#15978=CARTESIAN_POINT ( 'NONE',  ( -12.01549611932659722, 210.8513442034533227, 20.64886208192143613 ) ) ;
#15979=CARTESIAN_POINT ( 'NONE',  ( -9.984503880673420539, 203.7031108863293980, 29.34886208192143542 ) ) ;
#15981=CARTESIAN_POINT ( 'NONE',  ( 0.05014649552807549926, 219.6175466908591716, 67.25113791807856956 ) ) ;
#15982=CARTESIAN_POINT ( 'NONE',  ( -0.05014649552807731031, 198.5883022060938572, 86.75113791807856956 ) ) ;
#15984=CARTESIAN_POINT ( 'NONE',  ( 8.062137200540822946, 212.9164362838583315, 54.69886208192143329 ) ) ;
#15987=CARTESIAN_POINT ( 'NONE',  ( -0.05014649552828442242, 219.6175466908591716, 51.24886208192143755 ) ) ;
#15994=CARTESIAN_POINT ( 'NONE',  ( 8.015496119326531499, 209.5516654185219636, 43.85113791807856387 ) ) ;
#15996=CARTESIAN_POINT ( 'NONE',  ( 6.139770520408223575, 215.5359834540460611, 21.54886208192143826 ) ) ;
#16002=CARTESIAN_POINT ( 'NONE',  ( 6.500168698208244500, 202.3363017425938324, 4.298862081921435596 ) ) ;
#16003=CARTESIAN_POINT ( 'NONE',  ( -3.135527875058821579, 197.5041725223112223, 50.90113791807856813 ) ) ;
#16006=CARTESIAN_POINT ( 'NONE',  ( -0.05014649552810635652, 196.4853777576173002, 23.75113791807855890 ) ) ;
#16008=CARTESIAN_POINT ( 'NONE',  ( 2.426778023690075337, 214.6231898156240447, 93.39886208192143613 ) ) ;
#16012=CARTESIAN_POINT ( 'NONE',  ( -3.662846001190052991, 218.4274158808045740, 10.10113791807856742 ) ) ;
#16016=CARTESIAN_POINT ( 'NONE',  ( -6.139770520408369237, 215.5359834540460042, 57.95113791807856529 ) ) ;
#16017=CARTESIAN_POINT ( 'NONE',  ( -6.139770520408368348, 215.5359834540460042, 30.95113791807857240 ) ) ;
#16020=CARTESIAN_POINT ( 'NONE',  ( 3.135527875058981895, 197.5041725223112792, 1.598862081921434530 ) ) ;
#16024=CARTESIAN_POINT ( 'NONE',  ( -12.01549611932652972, 203.1486557965464499, 39.35113791807856387 ) ) ;
#16027=CARTESIAN_POINT ( 'NONE',  ( 8.062137200540822946, 212.9164362838583315, 21.69886208192143684 ) ) ;
#16030=CARTESIAN_POINT ( 'NONE',  ( -9.984503880673473830, 210.2968891136704315, 81.65113791807857524 ) ) ;
#16035=CARTESIAN_POINT ( 'NONE',  ( -0.05014649552807731031, 198.5883022060938572, 8.751137918078567779 ) ) ;
#16036=CARTESIAN_POINT ( 'NONE',  ( 12.00000000000000711, 207.0476921513415220, 93.99886208192144466 ) ) ;
#16042=CARTESIAN_POINT ( 'NONE',  ( 10.01549611932659545, 203.7984951890123853, 79.14886208192142192 ) ) ;
#16044=CARTESIAN_POINT ( 'NONE',  ( -6.139770520408369237, 215.5359834540460042, 21.95113791807856884 ) ) ;
#16049=CARTESIAN_POINT ( 'NONE',  ( 10.00000000000000711, 206.9523078486586201, 98.00113791807856956 ) ) ;
#16051=CARTESIAN_POINT ( 'NONE',  ( -10.01549611932653860, 203.7984951890123284, 87.35113791807854966 ) ) ;
#16056=CARTESIAN_POINT ( 'NONE',  ( 7.456977232089471386, 196.8216656703012006, 97.44886208192143329 ) ) ;
#16065=CARTESIAN_POINT ( 'NONE',  ( -8.118202686958138514, 212.8392687619910930, 92.79886208192144181 ) ) ;
#16066=CARTESIAN_POINT ( 'NONE',  ( -11.98450388067341876, 203.0532714938636047, 35.34886208192142476 ) ) ;
#16068=CARTESIAN_POINT ( 'NONE',  ( 10.01549611932653860, 210.2015048109876716, 43.85113791807854966 ) ) ;
#16070=CARTESIAN_POINT ( 'NONE',  ( 8.015496119326595448, 204.4483345814782638, 1.148862081921434797 ) ) ;
#16073=CARTESIAN_POINT ( 'NONE',  ( 0.05014649552828262524, 198.5883022060938572, 88.74886208192143044 ) ) ;
#16074=CARTESIAN_POINT ( 'NONE',  ( -4.903702542908602524, 213.8346818373418898, 33.95113791807857240 ) ) ;
#16076=VERTEX_POINT ( 'NONE', #12295 ) ;
#16080=CARTESIAN_POINT ( 'NONE',  ( 8.015496119326531499, 209.5516654185219636, 94.85113791807856387 ) ) ;
#16083=CARTESIAN_POINT ( 'NONE',  ( -4.984841277089891776, 213.7757310962905990, 68.94886208192144750 ) ) ;
#16086=CARTESIAN_POINT ( 'NONE',  ( 8.118202686958039038, 212.8392687619912635, 7.701137918078566180 ) ) ;
#16090=CARTESIAN_POINT ( 'NONE',  ( 0.05014649552807549926, 219.6175466908591716, 76.25113791807856956 ) ) ;
#16092=CARTESIAN_POINT ( 'NONE',  ( 8.062137200540920645, 201.0835637161417822, 98.30113791807858092 ) ) ;
#16095=CARTESIAN_POINT ( 'NONE',  ( 9.736236675708031640, 199.9851607334238963, 61.29886208192144892 ) ) ;
#16096=CARTESIAN_POINT ( 'NONE',  ( -8.118202686958138514, 212.8392687619910930, 65.79886208192144181 ) ) ;
#16097=CARTESIAN_POINT ( 'NONE',  ( -7.375838497908014268, 196.7627149292498530, 8.048862081921434708 ) ) ;
#16100=CARTESIAN_POINT ( 'NONE',  ( -9.984503880673473830, 210.2968891136704315, 12.65113791807856281 ) ) ;
#16101=CARTESIAN_POINT ( 'NONE',  ( -6.139770520408224463, 198.4640165459539389, 77.04886208192144181 ) ) ;
#16103=CARTESIAN_POINT ( 'NONE',  ( -0.05014649552810635652, 196.4853777576173002, 98.75113791807854113 ) ) ;
#16106=CARTESIAN_POINT ( 'NONE',  ( 0.05014649552828262524, 198.5883022060938572, 61.74886208192144466 ) ) ;
#16107=VERTEX_POINT ( 'NONE', #3791 ) ;
#16113=CARTESIAN_POINT ( 'NONE',  ( -6.500168698208129925, 202.3363017425936050, 60.20113791807857240 ) ) ;
#16116=CARTESIAN_POINT ( 'NONE',  ( -9.087479338623817071, 206.5556122393838336, 103.9243378854531130 ) ) ;
#16119=CARTESIAN_POINT ( 'NONE',  ( 0.05014649552828262524, 198.5883022060938572, 40.74886208192143755 ) ) ;
#16120=CARTESIAN_POINT ( 'NONE',  ( -3.044812012440131443, 216.5253028482142952, 79.10113791807857808 ) ) ;
#16122=CARTESIAN_POINT ( 'NONE',  ( 10.00000000000000711, 206.9523078486586201, 68.00113791807856956 ) ) ;
#16125=CARTESIAN_POINT ( 'NONE',  ( 0.05014649552807626948, 215.4116977939061144, 19.25113791807856245 ) ) ;
#16129=CARTESIAN_POINT ( 'NONE',  ( -9.736236675707914401, 199.9851607334237542, 48.20113791807858661 ) ) ;
#16131=CARTESIAN_POINT ( 'NONE',  ( 8.118202686958039038, 212.8392687619912635, 97.70113791807857240 ) ) ;
#16133=CARTESIAN_POINT ( 'NONE',  ( 8.118202686958039038, 212.8392687619912635, 70.70113791807857240 ) ) ;
#16134=CARTESIAN_POINT ( 'NONE',  ( 3.662846001189864698, 218.4274158808046593, 27.39886208192143613 ) ) ;
#16135=CARTESIAN_POINT ( 'NONE',  ( 8.062137200540822946, 212.9164362838583315, 42.69886208192143329 ) ) ;
#16137=CARTESIAN_POINT ( 'NONE',  ( 11.98450388067348271, 203.0532714938637753, 74.15113791807857524 ) ) ;
#16138=CARTESIAN_POINT ( 'NONE',  ( 8.000000000000008882, 206.9523078486586485, 92.00113791807858377 ) ) ;
#16139=CARTESIAN_POINT ( 'NONE',  ( 8.118202686958138514, 201.1607312380088501, 46.29886208192143471 ) ) ;
#16143=CARTESIAN_POINT ( 'NONE',  ( -12.00000000000000711, 206.9523078486584780, 53.49886208192144466 ) ) ;
#16151=CARTESIAN_POINT ( 'NONE',  ( 8.015496119326531499, 209.5516654185219636, 55.85113791807856387 ) ) ;
#16153=CARTESIAN_POINT ( 'NONE',  ( 3.135527875058981895, 197.5041725223112792, 34.59886208192143897 ) ) ;
#16158=CARTESIAN_POINT ( 'NONE',  ( -0.05014649552828365914, 215.4116977939061144, 9.248862081921435774 ) ) ;
#16160=CARTESIAN_POINT ( 'NONE',  ( -6.220909254589537696, 198.5229672870051161, 54.05113791807856671 ) ) ;
#16162=CARTESIAN_POINT ( 'NONE',  ( 3.044812012440130555, 197.4746971517856764, 35.60113791807857098 ) ) ;
#16167=CARTESIAN_POINT ( 'NONE',  ( 4.903702542908435547, 213.8346818373419751, 90.54886208192144181 ) ) ;
#16170=CARTESIAN_POINT ( 'NONE',  ( 9.736236675707914401, 214.0148392665762458, 19.70113791807856884 ) ) ;
#16173=CARTESIAN_POINT ( 'NONE',  ( -3.135527875058821579, 197.5041725223112223, 62.90113791807858235 ) ) ;
#16174=EDGE_CURVE ( 'NONE', #16107, #11012, #6299, .T. ) ;
#16175=CARTESIAN_POINT ( 'NONE',  ( 9.984503880673473830, 203.7031108863295401, 26.15113791807856813 ) ) ;
#16179=CARTESIAN_POINT ( 'NONE',  ( 3.135527875058981895, 197.5041725223112792, 13.59886208192143719 ) ) ;
#16182=CARTESIAN_POINT ( 'NONE',  ( 0.05014649552807549926, 219.6175466908591716, 37.25113791807857666 ) ) ;
#16184=CARTESIAN_POINT ( 'NONE',  ( 0.05014649552828275708, 196.4853777576173002, 19.74886208192143044 ) ) ;
#16188=CARTESIAN_POINT ( 'NONE',  ( 8.062137200540920645, 201.0835637161417822, 83.30113791807858092 ) ) ;
#16195=CARTESIAN_POINT ( 'NONE',  ( 6.444103211791042618, 202.2591342207267644, 11.30113791807856671 ) ) ;
#16198=CARTESIAN_POINT ( 'NONE',  ( 7.375838497908012492, 217.2372850707501186, 102.5488620819214560 ) ) ;
#16206=CARTESIAN_POINT ( 'NONE',  ( 0.05014649552828275708, 196.4853777576173002, 76.74886208192140202 ) ) ;
#16209=CARTESIAN_POINT ( 'NONE',  ( -10.01549611932653860, 203.7984951890123284, 18.35113791807856742 ) ) ;
#16211=CARTESIAN_POINT ( 'NONE',  ( -7.456977232089471386, 217.1783343296987709, 74.94886208192143329 ) ) ;
#16215=CARTESIAN_POINT ( 'NONE',  ( -3.044812012440131443, 216.5253028482142952, 82.10113791807857808 ) ) ;
#16218=CARTESIAN_POINT ( 'NONE',  ( 7.375838497908012492, 217.2372850707501186, 99.54886208192144181 ) ) ;
#16225=CARTESIAN_POINT ( 'NONE',  ( 3.662846001190051659, 195.5725841191953691, 8.601137918078565647 ) ) ;
#16230=CARTESIAN_POINT ( 'NONE',  ( -10.01549611932659545, 210.2015048109875011, 95.64886208192143613 ) ) ;
#16231=CARTESIAN_POINT ( 'NONE',  ( 7.375838497908012492, 217.2372850707501186, 36.54886208192144181 ) ) ;
#16233=CARTESIAN_POINT ( 'NONE',  ( -6.139770520408369237, 215.5359834540460042, 51.95113791807857950 ) ) ;
#16235=CARTESIAN_POINT ( 'NONE',  ( 0.05014649552828262524, 198.5883022060938572, 16.74886208192143755 ) ) ;
#16240=CARTESIAN_POINT ( 'NONE',  ( -7.984503880673422316, 204.3529502787951628, 86.34886208192143897 ) ) ;
#16243=B_SPLINE_CURVE_WITH_KNOTS ( 'NONE', 3,
 ( #5837, #21513, #8573, #3617, #16564, #18963 ),
 .UNSPECIFIED., .F., .F.,
 ( 4, 2, 4 ),
 ( -0.0003963451516553064642, -0.0001381393104116650271, 0.0001200665308319764099 ),
 .UNSPECIFIED. ) ;
#16245=CARTESIAN_POINT ( 'NONE',  ( -8.015496119326531499, 204.4483345814780364, 33.35113791807857098 ) ) ;
#16252=CARTESIAN_POINT ( 'NONE',  ( 8.000000000000008882, 206.9523078486586485, 98.00113791807856956 ) ) ;
#16255=CARTESIAN_POINT ( 'NONE',  ( -6.444103211790928043, 202.2591342207265939, 74.19886208192143329 ) ) ;
#16258=CARTESIAN_POINT ( 'NONE',  ( 3.135527875058820690, 216.4958274776887492, 13.40113791807856636 ) ) ;
#16262=CARTESIAN_POINT ( 'NONE',  ( -11.98450388067348804, 210.9467285061362247, 75.65113791807856103 ) ) ;
#16265=CARTESIAN_POINT ( 'NONE',  ( -3.044812012440131443, 216.5253028482142952, 100.1011379180785781 ) ) ;
#16268=CARTESIAN_POINT ( 'NONE',  ( 9.736236675708031640, 199.9851607334238963, 103.2988620819214560 ) ) ;
#16270=CARTESIAN_POINT ( 'NONE',  ( 11.98450388067341876, 210.9467285061363953, 57.84886208192143187 ) ) ;
#16271=CARTESIAN_POINT ( 'NONE',  ( -3.044812012439970683, 197.4746971517856196, 67.89886208192143613 ) ) ;
#16272=CARTESIAN_POINT ( 'NONE',  ( 3.753561863808876797, 195.6020594897209719, 1.598862081921433864 ) ) ;
#16274=CARTESIAN_POINT ( 'NONE',  ( -9.984503880673473830, 210.2968891136704315, 24.65113791807856103 ) ) ;
#16275=CARTESIAN_POINT ( 'NONE',  ( 6.220909254589681581, 198.5229672870052582, 79.44886208192143329 ) ) ;
#16280=CARTESIAN_POINT ( 'NONE',  ( -2.426778023690076225, 199.3768101843759553, 58.89886208192144323 ) ) ;
#16287=CARTESIAN_POINT ( 'NONE',  ( 2.517493886308900919, 214.5937144450984420, 73.40113791807856103 ) ) ;
#16288=PRESENTATION_STYLE_ASSIGNMENT (( #24124 ) ) ;
#16291=CARTESIAN_POINT ( 'NONE',  ( 4.984841277089891776, 200.2242689037093726, 40.44886208192144750 ) ) ;
#16292=CARTESIAN_POINT ( 'NONE',  ( 10.00000000000000711, 206.9523078486586201, 77.00113791807858377 ) ) ;
#16293=CARTESIAN_POINT ( 'NONE',  ( 3.135527875058820690, 216.4958274776887492, 61.40113791807857524 ) ) ;
#16295=CARTESIAN_POINT ( 'NONE',  ( -8.000000000000008882, 207.0476921513413515, 21.50113791807856956 ) ) ;
#16300=CARTESIAN_POINT ( 'NONE',  ( -12.00000000000000711, 207.0476921513413515, 45.50113791807856956 ) ) ;
#16302=CARTESIAN_POINT ( 'NONE',  ( -8.118202686958039038, 201.1607312380087080, 90.20113791807857240 ) ) ;
#16304=CARTESIAN_POINT ( 'NONE',  ( -0.05014649552810635652, 196.4853777576173002, 71.75113791807858377 ) ) ;
#16305=CARTESIAN_POINT ( 'NONE',  ( 9.736236675708031640, 199.9851607334238963, 28.29886208192143826 ) ) ;
#16306=CARTESIAN_POINT ( 'NONE',  ( -9.984503880673420539, 203.7031108863293980, 38.34886208192143187 ) ) ;
#16308=CARTESIAN_POINT ( 'NONE',  ( 12.00000000000000711, 206.9523078486586485, 77.00113791807858377 ) ) ;
#16309=CARTESIAN_POINT ( 'NONE',  ( -7.984503880673488041, 209.6470497212046098, 84.65113791807856103 ) ) ;
#16310=CARTESIAN_POINT ( 'NONE',  ( -10.00000000000000711, 206.9523078486584495, 50.49886208192143044 ) ) ;
#16313=CARTESIAN_POINT ( 'NONE',  ( -7.456977232089471386, 217.1783343296987709, 62.94886208192144039 ) ) ;
#16315=CARTESIAN_POINT ( 'NONE',  ( 0.05014649552828262524, 198.5883022060938572, 34.74886208192143755 ) ) ;
#16320=CARTESIAN_POINT ( 'NONE',  ( -8.015496119326531499, 204.4483345814780364, 48.35113791807857098 ) ) ;
#16322=CARTESIAN_POINT ( 'NONE',  ( -10.01549611932659722, 210.2015048109875011, 32.64886208192143613 ) ) ;
#16327=CARTESIAN_POINT ( 'NONE',  ( -8.000000000000008882, 206.9523078486584780, 11.49886208192143577 ) ) ;
#16328=CARTESIAN_POINT ( 'NONE',  ( -3.135527875058821579, 197.5041725223112223, 47.90113791807857524 ) ) ;
#16330=CARTESIAN_POINT ( 'NONE',  ( -3.044812012440131443, 216.5253028482142952, 40.10113791807857098 ) ) ;
#16333=CARTESIAN_POINT ( 'NONE',  ( -0.05014649552828365914, 215.4116977939061144, 102.2488620819214447 ) ) ;
#16336=CARTESIAN_POINT ( 'NONE',  ( -1.474514954580286030E-14, 206.9977241638431167, -6.000000000000014211 ) ) ;
#16337=CARTESIAN_POINT ( 'NONE',  ( -7.375838497908182134, 217.2372850707499765, 18.95113791807856529 ) ) ;
#16340=CARTESIAN_POINT ( 'NONE',  ( -3.044812012440131443, 216.5253028482142952, 70.10113791807857808 ) ) ;
#16341=CARTESIAN_POINT ( 'NONE',  ( -9.984503880673475606, 210.2968891136704315, 36.65113791807856813 ) ) ;
#16344=CARTESIAN_POINT ( 'NONE',  ( 6.220909254589680693, 198.5229672870052582, 7.448862081921434175 ) ) ;
#16347=CARTESIAN_POINT ( 'NONE',  ( -9.736236675707914401, 199.9851607334237542, 45.20113791807857240 ) ) ;
#16349=CARTESIAN_POINT ( 'NONE',  ( -8.118202686958138514, 212.8392687619910930, 17.79886208192143826 ) ) ;
#16352=CARTESIAN_POINT ( 'NONE',  ( -6.220909254589537696, 198.5229672870051161, 84.05113791807855250 ) ) ;
#16357=CARTESIAN_POINT ( 'NONE',  ( 6.444103211791042618, 202.2591342207267644, 20.30113791807857027 ) ) ;
#16360=CARTESIAN_POINT ( 'NONE',  ( 7.456977232089471386, 196.8216656703012006, 103.4488620819214475 ) ) ;
#16368=CARTESIAN_POINT ( 'NONE',  ( 8.118202686958138514, 201.1607312380088501, 94.29886208192144181 ) ) ;
#16370=CARTESIAN_POINT ( 'NONE',  ( -8.062137200540920645, 212.9164362838581894, 24.80113791807857027 ) ) ;
#16372=CARTESIAN_POINT ( 'NONE',  ( -11.98450388067341876, 203.0532714938636047, 83.34886208192143897 ) ) ;
#16376=CARTESIAN_POINT ( 'NONE',  ( 8.551039143100592099, 208.8253170565643302, -0.4549153643320029139 ) ) ;
#16377=CARTESIAN_POINT ( 'NONE',  ( 6.139770520408368348, 198.4640165459539674, 98.45113791807854398 ) ) ;
#16380=CARTESIAN_POINT ( 'NONE',  ( 6.220909254589536808, 215.4770327129947702, 40.55113791807855250 ) ) ;
#16385=CARTESIAN_POINT ( 'NONE',  ( -7.456977232089304408, 196.8216656703010301, 24.05113791807857027 ) ) ;
#16390=CARTESIAN_POINT ( 'NONE',  ( 10.00000000000000711, 207.0476921513415220, 93.99886208192144466 ) ) ;
#16392=CARTESIAN_POINT ( 'NONE',  ( -3.753561863808878130, 218.3979405102790281, 36.09886208192143187 ) ) ;
#16394=CARTESIAN_POINT ( 'NONE',  ( -10.00000000000000711, 207.0476921513413515, 51.50113791807857666 ) ) ;
#16397=CARTESIAN_POINT ( 'NONE',  ( -6.444103211790928043, 202.2591342207265939, 11.19886208192143506 ) ) ;
#16400=CARTESIAN_POINT ( 'NONE',  ( 4.984841277089891776, 200.2242689037093726, 97.44886208192143329 ) ) ;
#16402=CARTESIAN_POINT ( 'NONE',  ( -8.000000000000008882, 207.0476921513413515, 42.50113791807857666 ) ) ;
#16407=CARTESIAN_POINT ( 'NONE',  ( 3.044812012439969795, 216.5253028482143520, 54.39886208192143613 ) ) ;
#16410=CARTESIAN_POINT ( 'NONE',  ( -2.517493886308901807, 199.4062855549015012, 95.90113791807857524 ) ) ;
#16413=CARTESIAN_POINT ( 'NONE',  ( 4.984841277089891776, 200.2242689037093726, 76.44886208192143329 ) ) ;
#16417=CARTESIAN_POINT ( 'NONE',  ( 6.220909254589536808, 215.4770327129947987, 10.55113791807856494 ) ) ;
#16422=CARTESIAN_POINT ( 'NONE',  ( 3.662846001190051659, 195.5725841191953691, 80.60113791807857808 ) ) ;
#16424=CARTESIAN_POINT ( 'NONE',  ( 3.044812012440130555, 197.4746971517856764, 101.6011379180785781 ) ) ;
#16427=CARTESIAN_POINT ( 'NONE',  ( -12.00000000000000711, 206.9523078486584780, 104.4988620819214304 ) ) ;
#16428=CARTESIAN_POINT ( 'NONE',  ( 3.662846001189864698, 218.4274158808046593, 63.39886208192144323 ) ) ;
#16429=CARTESIAN_POINT ( 'NONE',  ( 6.139770520408223575, 215.5359834540460611, 66.54886208192144181 ) ) ;
#16430=CARTESIAN_POINT ( 'NONE',  ( -12.01549611932659722, 210.8513442034533227, 5.648862081921434353 ) ) ;
#16432=CARTESIAN_POINT ( 'NONE',  ( 3.135527875058820690, 216.4958274776887492, 19.40113791807856813 ) ) ;
#16434=CARTESIAN_POINT ( 'NONE',  ( 10.01549611932659545, 203.7984951890123853, 91.14886208192140771 ) ) ;
#16440=CARTESIAN_POINT ( 'NONE',  ( 8.015496119326595448, 204.4483345814782638, 64.14886208192143613 ) ) ;
#16443=ORIENTED_EDGE ( 'NONE', *, *, #6230, .T. ) ;
#16448=CARTESIAN_POINT ( 'NONE',  ( 2.517493886308900919, 214.5937144450984420, 67.40113791807856103 ) ) ;
#16449=( NAMED_UNIT ( * ) PLANE_ANGLE_UNIT ( ) SI_UNIT ( $, .RADIAN. ) );
#16452=CARTESIAN_POINT ( 'NONE',  ( 6.500168698208244500, 202.3363017425938324, 46.29886208192144892 ) ) ;
#16453=CARTESIAN_POINT ( 'NONE',  ( 9.984503880673470277, 203.7031108863295401, 80.15113791807858945 ) ) ;
#16454=CARTESIAN_POINT ( 'NONE',  ( 0.05014649552810505201, 217.5146222423826714, 70.25113791807858377 ) ) ;
#16458=CARTESIAN_POINT ( 'NONE',  ( -6.500168698208129925, 202.3363017425936050, 24.20113791807856529 ) ) ;
#16462=CARTESIAN_POINT ( 'NONE',  ( 12.01549611932652972, 210.8513442034534933, 46.85113791807857098 ) ) ;
#16464=CARTESIAN_POINT ( 'NONE',  ( 6.220909254589536808, 215.4770327129947702, 91.55113791807858092 ) ) ;
#16466=CARTESIAN_POINT ( 'NONE',  ( 9.984503880673473830, 203.7031108863295401, 71.15113791807857524 ) ) ;
#16467=CARTESIAN_POINT ( 'NONE',  ( 3.662846001189864698, 218.4274158808046593, 30.39886208192143613 ) ) ;
#16468=CARTESIAN_POINT ( 'NONE',  ( 8.062137200540822946, 212.9164362838583315, 36.69886208192143329 ) ) ;
#16471=CARTESIAN_POINT ( 'NONE',  ( 3.753561863808689836, 218.3979405102790565, 79.40113791807858945 ) ) ;
#16472=CARTESIAN_POINT ( 'NONE',  ( 6.500168698208129925, 211.6636982574063381, 97.70113791807858661 ) ) ;
#16474=CARTESIAN_POINT ( 'NONE',  ( -3.135527875058982783, 216.4958274776886924, 57.09886208192143187 ) ) ;
#16477=ORIENTED_EDGE ( 'NONE', *, *, #25823, .F. ) ;
#16478=CARTESIAN_POINT ( 'NONE',  ( 3.753561863808876797, 195.6020594897209719, 58.59886208192143897 ) ) ;
#16480=CARTESIAN_POINT ( 'NONE',  ( -6.444103211790928043, 202.2591342207265939, 35.19886208192144039 ) ) ;
#16486=CARTESIAN_POINT ( 'NONE',  ( -6.500168698208129925, 202.3363017425936050, 48.20113791807858661 ) ) ;
#16488=CARTESIAN_POINT ( 'NONE',  ( 8.062137200540822946, 212.9164362838583315, 36.69886208192143329 ) ) ;
#16495=CARTESIAN_POINT ( 'NONE',  ( 6.444103211790928043, 211.7408657792734061, 18.69886208192143684 ) ) ;
#16496=CARTESIAN_POINT ( 'NONE',  ( 8.118202686958039038, 212.8392687619912635, 52.70113791807857240 ) ) ;
#16498=CARTESIAN_POINT ( 'NONE',  ( -9.984503880673473830, 210.2968891136704315, 36.65113791807855392 ) ) ;
#16502=CARTESIAN_POINT ( 'NONE',  ( -7.984503880673422316, 204.3529502787951628, 104.3488620819214532 ) ) ;
#16506=CARTESIAN_POINT ( 'NONE',  ( 3.753561863808689836, 218.3979405102790565, 19.40113791807856813 ) ) ;
#16509=CARTESIAN_POINT ( 'NONE',  ( -10.01549611932653860, 203.7984951890123284, 63.35113791807857098 ) ) ;
#16510=CARTESIAN_POINT ( 'NONE',  ( -3.135527875058821579, 197.5041725223112223, 38.90113791807857524 ) ) ;
#16513=CARTESIAN_POINT ( 'NONE',  ( -12.01549611932659722, 210.8513442034533227, 5.648862081921434353 ) ) ;
#16514=CARTESIAN_POINT ( 'NONE',  ( 0.05014649552828275014, 196.4853777576173002, 7.748862081921435774 ) ) ;
#16517=CARTESIAN_POINT ( 'NONE',  ( -12.00000000000000711, 207.0476921513413515, 48.50113791807856956 ) ) ;
#16518=CARTESIAN_POINT ( 'NONE',  ( -7.984503880673488041, 209.6470497212046098, 69.65113791807856103 ) ) ;
#16520=CARTESIAN_POINT ( 'NONE',  ( 10.00000000000000711, 207.0476921513415220, 21.99886208192143755 ) ) ;
#16524=CARTESIAN_POINT ( 'NONE',  ( -8.062137200540920645, 212.9164362838581894, 84.80113791807856671 ) ) ;
#16529=CARTESIAN_POINT ( 'NONE',  ( -8.000000000000008882, 207.0476921513413515, 21.50113791807856956 ) ) ;
#16532=CARTESIAN_POINT ( 'NONE',  ( 3.044812012439969795, 216.5253028482143520, 6.398862081921435241 ) ) ;
#16540=CARTESIAN_POINT ( 'NONE',  ( -6.139770520408224463, 198.4640165459539389, 92.04886208192139918 ) ) ;
#16542=CARTESIAN_POINT ( 'NONE',  ( -8.118202686958039038, 201.1607312380087080, 24.20113791807856884 ) ) ;
#16544=CARTESIAN_POINT ( 'NONE',  ( 11.98450388067341876, 210.9467285061363953, 75.84886208192143897 ) ) ;
#16549=CARTESIAN_POINT ( 'NONE',  ( 10.01549611932653860, 210.2015048109876716, 91.85113791807853545 ) ) ;
#16553=CARTESIAN_POINT ( 'NONE',  ( 0.05014649552810505201, 217.5146222423826714, 37.25113791807855534 ) ) ;
#16558=CARTESIAN_POINT ( 'NONE',  ( -3.662846001190052991, 218.4274158808045740, 16.10113791807856742 ) ) ;
#16563=CARTESIAN_POINT ( 'NONE',  ( 7.456977232089471386, 196.8216656703012006, 31.44886208192143684 ) ) ;
#16564=CARTESIAN_POINT ( 'NONE',  ( -10.08243921202409688, 207.8094824920489714, 102.5360034692371869 ) ) ;
#16566=CARTESIAN_POINT ( 'NONE',  ( 3.135527875058820690, 216.4958274776887492, 49.40113791807857524 ) ) ;
#16568=CARTESIAN_POINT ( 'NONE',  ( 2.517493886309087436, 199.4062855549015865, 13.59886208192143719 ) ) ;
#16573=CARTESIAN_POINT ( 'NONE',  ( -8.000000000000008882, 206.9523078486584780, 98.49886208192143044 ) ) ;
#16574=CARTESIAN_POINT ( 'NONE',  ( 8.015496119326531499, 209.5516654185219636, 40.85113791807856387 ) ) ;
#16578=CARTESIAN_POINT ( 'NONE',  ( 10.00000000000000711, 207.0476921513415220, 57.99886208192143044 ) ) ;
#16581=CARTESIAN_POINT ( 'NONE',  ( 7.984503880673485376, 204.3529502787953902, 98.15113791807856103 ) ) ;
#16584=CARTESIAN_POINT ( 'NONE',  ( -7.984503880673422316, 204.3529502787951628, 68.34886208192142476 ) ) ;
#16587=CARTESIAN_POINT ( 'NONE',  ( -3.135527875058821579, 197.5041725223112223, 14.90113791807856636 ) ) ;
#16592=CARTESIAN_POINT ( 'NONE',  ( -3.753561863808691168, 195.6020594897209435, 77.90113791807856103 ) ) ;
#16593=CARTESIAN_POINT ( 'NONE',  ( -8.118202686958039038, 201.1607312380087080, 99.20113791807858661 ) ) ;
#16597=CARTESIAN_POINT ( 'NONE',  ( -0.05014649552828403384, 217.5146222423826714, 6.248862081921433109 ) ) ;
#16598=CARTESIAN_POINT ( 'NONE',  ( -9.736236675708031640, 214.0148392665760753, 62.79886208192144892 ) ) ;
#16599=CARTESIAN_POINT ( 'NONE',  ( -10.01549611932659545, 210.2015048109875011, 62.64886208192144323 ) ) ;
#16600=CARTESIAN_POINT ( 'NONE',  ( 12.01549611932659367, 203.1486557965466773, 4.148862081921434353 ) ) ;
#16602=CARTESIAN_POINT ( 'NONE',  ( -3.044812012440131443, 216.5253028482142952, 19.10113791807856742 ) ) ;
#16603=CARTESIAN_POINT ( 'NONE',  ( -8.062137200540822946, 201.0835637161416400, 92.19886208192143329 ) ) ;
#16610=CARTESIAN_POINT ( 'NONE',  ( 2.517493886309087436, 199.4062855549015865, 73.59886208192142476 ) ) ;
#16614=DIRECTION ( 'NONE',  ( -0.5526942671207061286, -0.1536855300543007730, -0.8190908404712107238 ) ) ;
#16617=CARTESIAN_POINT ( 'NONE',  ( 4.984841277089725686, 213.7757310962907411, 70.55113791807856671 ) ) ;
#16622=CARTESIAN_POINT ( 'NONE',  ( -7.984503880673422316, 204.3529502787951628, 47.34886208192143897 ) ) ;
#16624=CARTESIAN_POINT ( 'NONE',  ( -3.135527875058821579, 197.5041725223112223, 86.90113791807857524 ) ) ;
#16625=CARTESIAN_POINT ( 'NONE',  ( 10.01549611932653860, 210.2015048109876716, 64.85113791807857808 ) ) ;
#16627=CARTESIAN_POINT ( 'NONE',  ( -4.984841277089726574, 200.2242689037092305, 21.05113791807857027 ) ) ;
#16631=CARTESIAN_POINT ( 'NONE',  ( 0.05014649552807549926, 219.6175466908591716, 52.25113791807857666 ) ) ;
#16633=CARTESIAN_POINT ( 'NONE',  ( 6.139770520408368348, 198.4640165459539674, 92.45113791807857240 ) ) ;
#16634=CARTESIAN_POINT ( 'NONE',  ( -3.044812012440131443, 216.5253028482142952, 73.10113791807857808 ) ) ;
#16635=CARTESIAN_POINT ( 'NONE',  ( 7.375838497908012492, 217.2372850707501186, 30.54886208192144181 ) ) ;
#16636=CARTESIAN_POINT ( 'NONE',  ( 6.220909254589680693, 198.5229672870052582, 34.44886208192143329 ) ) ;
#16638=CARTESIAN_POINT ( 'NONE',  ( 7.375838497908181246, 196.7627149292499666, 77.45113791807855819 ) ) ;
#16639=CARTESIAN_POINT ( 'NONE',  ( 10.00000000000000711, 206.9523078486586201, -0.9988620819214343305 ) ) ;
#16640=CARTESIAN_POINT ( 'NONE',  ( 6.139770520408223575, 215.5359834540460611, 57.54886208192142050 ) ) ;
#16642=CARTESIAN_POINT ( 'NONE',  ( -12.01549611932659722, 210.8513442034533227, 65.64886208192142192 ) ) ;
#16645=CARTESIAN_POINT ( 'NONE',  ( -8.000000000000008882, 206.9523078486584780, 44.49886208192143755 ) ) ;
#16653=DIRECTION ( 'NONE',  ( 0.5526942671207055735, 0.1536855300543024383, 0.8190908404712107238 ) ) ;
#16654=CARTESIAN_POINT ( 'NONE',  ( -6.500168698208129925, 202.3363017425936050, 51.20113791807857240 ) ) ;
#16656=B_SPLINE_CURVE_WITH_KNOTS ( 'NONE', 3,
 ( #30580, #25633, #7243, #31376 ),
 .UNSPECIFIED., .F., .F.,
 ( 4, 4 ),
 ( 0.001859822337438910272, 0.001914709330258871581 ),
 .UNSPECIFIED. ) ;
#16657=CARTESIAN_POINT ( 'NONE',  ( -8.062137200540822946, 201.0835637161416400, 32.19886208192143329 ) ) ;
#16664=CARTESIAN_POINT ( 'NONE',  ( -0.05014649552828365914, 215.4116977939061144, 15.24886208192143577 ) ) ;
#16666=CARTESIAN_POINT ( 'NONE',  ( 6.220909254589536808, 215.4770327129947702, 61.55113791807858092 ) ) ;
#16667=CARTESIAN_POINT ( 'NONE',  ( -0.05014649552810635652, 196.4853777576173002, 32.75113791807856956 ) ) ;
#16670=CARTESIAN_POINT ( 'NONE',  ( 7.984503880673422316, 209.6470497212048372, 102.8488620819214390 ) ) ;
#16674=CARTESIAN_POINT ( 'NONE',  ( 12.00000000000000711, 206.9523078486586485, 23.00113791807856600 ) ) ;
#16676=CARTESIAN_POINT ( 'NONE',  ( 6.220909254589536808, 215.4770327129947702, 70.55113791807856671 ) ) ;
#16677=CARTESIAN_POINT ( 'NONE',  ( 9.984503880673473830, 203.7031108863295401, 41.15113791807856813 ) ) ;
#16679=DIRECTION ( 'NONE',  ( 0.9366133782696128840, 0.000000000000000000, 0.3503646381220332229 ) ) ;
#16681=CARTESIAN_POINT ( 'NONE',  ( -0.05014649552828442242, 219.6175466908591716, 6.248862081921433997 ) ) ;
#16682=CARTESIAN_POINT ( 'NONE',  ( -6.139770520408224463, 198.4640165459539105, 5.048862081921435596 ) ) ;
#16685=CARTESIAN_POINT ( 'NONE',  ( 7.375838497908181246, 196.7627149292499666, 50.45113791807855819 ) ) ;
#16686=CARTESIAN_POINT ( 'NONE',  ( -2.517493886308901807, 199.4062855549015012, 65.90113791807856103 ) ) ;
#16688=CARTESIAN_POINT ( 'NONE',  ( 8.118202686958138514, 201.1607312380088501, 34.29886208192143471 ) ) ;
#16692=CARTESIAN_POINT ( 'NONE',  ( 9.984503880673470277, 203.7031108863295401, 80.15113791807858945 ) ) ;
#16697=CARTESIAN_POINT ( 'NONE',  ( -7.984503880673488041, 209.6470497212046098, 24.65113791807857169 ) ) ;
#16701=CARTESIAN_POINT ( 'NONE',  ( -10.01549611932659722, 210.2015048109875011, 8.648862081921436129 ) ) ;
#16705=CARTESIAN_POINT ( 'NONE',  ( -8.015496119326531499, 204.4483345814780364, 51.35113791807857098 ) ) ;
#16708=CARTESIAN_POINT ( 'NONE',  ( 10.01549611932659545, 203.7984951890123853, 88.14886208192143613 ) ) ;
#16710=CARTESIAN_POINT ( 'NONE',  ( 8.118202686958039038, 212.8392687619912635, 25.70113791807856529 ) ) ;
#16712=CARTESIAN_POINT ( 'NONE',  ( 9.736236675708031640, 199.9851607334238963, 76.29886208192142760 ) ) ;
#16717=CARTESIAN_POINT ( 'NONE',  ( 3.135527875058820690, 216.4958274776887492, 97.40113791807858945 ) ) ;
#16720=CARTESIAN_POINT ( 'NONE',  ( 3.044812012440130555, 197.4746971517856764, 41.60113791807857808 ) ) ;
#16725=CARTESIAN_POINT ( 'NONE',  ( 3.662846001190051659, 195.5725841191953691, 17.60113791807856742 ) ) ;
#16731=CARTESIAN_POINT ( 'NONE',  ( 0.05014649552828288198, 194.3824533091408000, 46.74886208192143755 ) ) ;
#16733=CARTESIAN_POINT ( 'NONE',  ( -8.062137200540920645, 212.9164362838581894, 54.80113791807857382 ) ) ;
#16735=VECTOR ( 'NONE', #24594, 1000.000000000000114 ) ;
#16736=CARTESIAN_POINT ( 'NONE',  ( -0.05014649552828365914, 215.4116977939061144, 18.24886208192143755 ) ) ;
#16740=CARTESIAN_POINT ( 'NONE',  ( 4.984841277089891776, 200.2242689037093726, 103.4488620819214475 ) ) ;
#16742=CARTESIAN_POINT ( 'NONE',  ( 6.444103211791042618, 202.2591342207267644, 44.30113791807857382 ) ) ;
#16746=CIRCLE ( 'NONE', #2079, 1.000000000000000222 ) ;
#16747=CARTESIAN_POINT ( 'NONE',  ( 8.118202686958138514, 201.1607312380088501, 64.29886208192144181 ) ) ;
#16750=CARTESIAN_POINT ( 'NONE',  ( 4.984841277089725686, 213.7757310962907411, 97.55113791807858092 ) ) ;
#16752=ADVANCED_FACE ( 'NONE', ( #29308 ), #11250, .T. ) ;
#16754=COLOUR_RGB ( '', 0.08235294, 0.09019608, 0.10196078) ;
#16757=CARTESIAN_POINT ( 'NONE',  ( -2.426778023690076225, 199.3768101843759553, 76.89886208192143613 ) ) ;
#16762=CARTESIAN_POINT ( 'NONE',  ( 6.220909254589536808, 215.4770327129947987, 19.55113791807856671 ) ) ;
#16764=DIRECTION ( 'NONE',  ( 0.000000000000000000, 0.9988620819214357738, 0.04769215134144196705 ) ) ;
#16766=CARTESIAN_POINT ( 'NONE',  ( 3.753561863808689836, 218.3979405102790565, 91.40113791807857524 ) ) ;
#16767=CARTESIAN_POINT ( 'NONE',  ( 10.00000000000000711, 206.9523078486586201, 95.00113791807856956 ) ) ;
#16770=CARTESIAN_POINT ( 'NONE',  ( -0.05014649552828403384, 217.5146222423826714, 3.248862081921433997 ) ) ;
#16771=CARTESIAN_POINT ( 'NONE',  ( -7.456977232089471386, 217.1783343296987709, 56.94886208192144039 ) ) ;
#16772=CARTESIAN_POINT ( 'NONE',  ( 0.05014649552828275014, 196.4853777576173002, 79.74886208192143044 ) ) ;
#16773=CARTESIAN_POINT ( 'NONE',  ( -7.456977232089471386, 217.1783343296987709, 2.948862081921434175 ) ) ;
#16776=CARTESIAN_POINT ( 'NONE',  ( 6.220909254589536808, 215.4770327129947702, 19.55113791807856671 ) ) ;
#16777=CARTESIAN_POINT ( 'NONE',  ( -6.220909254589682469, 215.4770327129946850, 92.94886208192143329 ) ) ;
#16782=CARTESIAN_POINT ( 'NONE',  ( 4.903702542908435547, 213.8346818373419751, 69.54886208192141339 ) ) ;
#16787=CARTESIAN_POINT ( 'NONE',  ( 0.05014649552807626948, 215.4116977939061144, 67.25113791807856956 ) ) ;
#16791=CARTESIAN_POINT ( 'NONE',  ( 0.05014649552828262524, 198.5883022060938572, 46.74886208192144466 ) ) ;
#16793=CARTESIAN_POINT ( 'NONE',  ( -10.00000000000000711, 207.0476921513413515, 90.50113791807858377 ) ) ;
#16794=CARTESIAN_POINT ( 'NONE',  ( 8.062137200540920645, 201.0835637161417822, 74.30113791807858092 ) ) ;
#16801=CARTESIAN_POINT ( 'NONE',  ( -0.05014649552807705357, 194.3824533091408000, 50.75113791807857666 ) ) ;
#16803=CARTESIAN_POINT ( 'NONE',  ( 0.05014649552810505201, 217.5146222423826714, 94.25113791807855534 ) ) ;
#16804=CARTESIAN_POINT ( 'NONE',  ( -9.984503880673475606, 210.2968891136704315, 66.65113791807857524 ) ) ;
#16806=CARTESIAN_POINT ( 'NONE',  ( -11.98450388067341876, 203.0532714938636047, 32.34886208192142476 ) ) ;
#16807=CARTESIAN_POINT ( 'NONE',  ( 9.984503880673420539, 210.2968891136705736, 51.84886208192143897 ) ) ;
#16810=CARTESIAN_POINT ( 'NONE',  ( 0.05014649552807549926, 219.6175466908591716, 73.25113791807858377 ) ) ;
#16811=CARTESIAN_POINT ( 'NONE',  ( 7.984503880673485376, 204.3529502787953902, 98.15113791807856103 ) ) ;
#16813=CARTESIAN_POINT ( 'NONE',  ( 6.139770520408223575, 215.5359834540460611, 63.54886208192144181 ) ) ;
#16816=CARTESIAN_POINT ( 'NONE',  ( 7.375838497908012492, 217.2372850707501186, 63.54886208192144181 ) ) ;
#16819=CARTESIAN_POINT ( 'NONE',  ( -0.05014649552828365914, 215.4116977939061144, 45.24886208192144466 ) ) ;
#16820=CIRCLE ( 'NONE', #2151, 0.9999999999999941158 ) ;
#16825=CARTESIAN_POINT ( 'NONE',  ( -9.000000000000005329, 207.1715159932409733, 103.3438395974723818 ) ) ;
#16826=CARTESIAN_POINT ( 'NONE',  ( -0.05014649552807731031, 198.5883022060938572, 53.75113791807857666 ) ) ;
#16829=CARTESIAN_POINT ( 'NONE',  ( 0.05014649552828275708, 196.4853777576173002, 31.74886208192143044 ) ) ;
#16835=CARTESIAN_POINT ( 'NONE',  ( -8.015496119326597224, 209.5516654185217362, 14.64886208192143258 ) ) ;
#16836=CARTESIAN_POINT ( 'NONE',  ( 0.05014649552810505201, 217.5146222423826714, 58.25113791807856245 ) ) ;
#16837=CARTESIAN_POINT ( 'NONE',  ( -3.044812012440131443, 216.5253028482142952, 34.10113791807857808 ) ) ;
#16840=CARTESIAN_POINT ( 'NONE',  ( -8.000000000000008882, 207.0476921513413515, 0.5011379180785658916 ) ) ;
#16844=CARTESIAN_POINT ( 'NONE',  ( 12.00000000000000711, 206.9523078486586485, 20.00113791807856956 ) ) ;
#16848=CARTESIAN_POINT ( 'NONE',  ( 6.220909254589536808, 215.4770327129947702, 61.55113791807858092 ) ) ;
#16849=CARTESIAN_POINT ( 'NONE',  ( 6.220909254589536808, 215.4770327129947987, 40.55113791807856671 ) ) ;
#16852=CARTESIAN_POINT ( 'NONE',  ( 0.05014649552828288198, 194.3824533091408000, 1.748862081921433775 ) ) ;
#16853=CARTESIAN_POINT ( 'NONE',  ( 9.984503880673420539, 210.2968891136705736, 6.848862081921434530 ) ) ;
#16856=CARTESIAN_POINT ( 'NONE',  ( -7.456977232089304408, 196.8216656703010301, 48.05113791807856671 ) ) ;
#16857=CARTESIAN_POINT ( 'NONE',  ( -8.015496119326531499, 204.4483345814780364, 72.35113791807857808 ) ) ;
#16859=CARTESIAN_POINT ( 'NONE',  ( -6.139770520408224463, 198.4640165459539389, 29.04886208192143471 ) ) ;
#16862=CARTESIAN_POINT ( 'NONE',  ( 10.01549611932653860, 210.2015048109876716, 85.85113791807857808 ) ) ;
#16868=CARTESIAN_POINT ( 'NONE',  ( 6.500168698208129925, 211.6636982574063381, 22.70113791807856529 ) ) ;
#16870=CARTESIAN_POINT ( 'NONE',  ( 8.118202686958138514, 201.1607312380088501, 1.298862081921434486 ) ) ;
#16872=VERTEX_POINT ( 'NONE', #29646 ) ;
#16873=CARTESIAN_POINT ( 'NONE',  ( 4.903702542908601636, 200.1653181626581102, 50.45113791807857240 ) ) ;
#16876=CARTESIAN_POINT ( 'NONE',  ( -10.00000000000000711, 206.9523078486584495, 89.49886208192144466 ) ) ;
#16878=CARTESIAN_POINT ( 'NONE',  ( -0.05014649552810635652, 196.4853777576173002, 32.75113791807856956 ) ) ;
#16880=CARTESIAN_POINT ( 'NONE',  ( -12.01549611932659722, 210.8513442034533227, 83.64886208192143613 ) ) ;
#16884=CARTESIAN_POINT ( 'NONE',  ( 8.062137200540920645, 201.0835637161417822, 95.30113791807858092 ) ) ;
#16887=CARTESIAN_POINT ( 'NONE',  ( 8.118202686958039038, 212.8392687619912635, 37.70113791807857240 ) ) ;
#16894=CARTESIAN_POINT ( 'NONE',  ( -11.98450388067348804, 210.9467285061362247, 21.65113791807856813 ) ) ;
#16899=CARTESIAN_POINT ( 'NONE',  ( 3.662846001189864698, 218.4274158808046593, 39.39886208192143613 ) ) ;
#16900=CARTESIAN_POINT ( 'NONE',  ( -10.01549611932653860, 203.7984951890123284, 3.351137918078566091 ) ) ;
#16901=CARTESIAN_POINT ( 'NONE',  ( 8.118202686958039038, 212.8392687619912635, 52.70113791807857240 ) ) ;
#16902=CARTESIAN_POINT ( 'NONE',  ( 4.903702542908435547, 213.8346818373419751, 15.54886208192143826 ) ) ;
#16907=CARTESIAN_POINT ( 'NONE',  ( -2.426778023690076225, 199.3768101843759553, 100.8988620819214361 ) ) ;
#16909=CARTESIAN_POINT ( 'NONE',  ( 4.903702542908601636, 200.1653181626581102, 44.45113791807857240 ) ) ;
#16914=CARTESIAN_POINT ( 'NONE',  ( -10.00000000000000711, 206.9523078486584495, 65.49886208192143044 ) ) ;
#16917=CARTESIAN_POINT ( 'NONE',  ( 6.220909254589536808, 215.4770327129947702, 4.551137918078564937 ) ) ;
#16920=CARTESIAN_POINT ( 'NONE',  ( 7.984503880673422316, 209.6470497212048372, 84.84886208192142476 ) ) ;
#16926=CARTESIAN_POINT ( 'NONE',  ( -8.118202686958039038, 201.1607312380087080, 24.20113791807856884 ) ) ;
#16931=CARTESIAN_POINT ( 'NONE',  ( -7.456977232089304408, 196.8216656703010301, 87.05113791807856671 ) ) ;
#16935=CARTESIAN_POINT ( 'NONE',  ( -11.98450388067341876, 203.0532714938636047, 68.34886208192142476 ) ) ;
#16936=CARTESIAN_POINT ( 'NONE',  ( -9.984503880673420539, 203.7031108863293980, 77.34886208192143897 ) ) ;
#16937=CARTESIAN_POINT ( 'NONE',  ( -0.05014649552828442242, 219.6175466908591716, 15.24886208192143577 ) ) ;
#16939=CARTESIAN_POINT ( 'NONE',  ( 8.062137200540920645, 201.0835637161417822, 20.30113791807856671 ) ) ;
#16940=CARTESIAN_POINT ( 'NONE',  ( 10.01549611932659545, 203.7984951890123853, 88.14886208192143613 ) ) ;
#16946=CARTESIAN_POINT ( 'NONE',  ( 6.444103211790928043, 211.7408657792734061, 75.69886208192143329 ) ) ;
#16955=CARTESIAN_POINT ( 'NONE',  ( 7.984503880673485376, 204.3529502787953902, 65.15113791807856103 ) ) ;
#16960=CARTESIAN_POINT ( 'NONE',  ( 2.517493886309087436, 199.4062855549015865, 49.59886208192143897 ) ) ;
#16961=CARTESIAN_POINT ( 'NONE',  ( -8.062137200540920645, 212.9164362838581894, 75.80113791807858092 ) ) ;
#16966=CARTESIAN_POINT ( 'NONE',  ( -12.00000000000000711, 207.0476921513413515, 57.50113791807856956 ) ) ;
#16968=CARTESIAN_POINT ( 'NONE',  ( 12.00000000000000711, 206.9523078486586485, 5.001137918078565114 ) ) ;
#16969=CARTESIAN_POINT ( 'NONE',  ( -3.044812012440131443, 216.5253028482142952, 76.10113791807856387 ) ) ;
#16970=CARTESIAN_POINT ( 'NONE',  ( 12.00000000000000711, 207.0476921513415220, 36.99886208192143044 ) ) ;
#16971=CARTESIAN_POINT ( 'NONE',  ( 10.01549611932659367, 203.7984951890124421, 52.14886208192142902 ) ) ;
#16973=CARTESIAN_POINT ( 'NONE',  ( -9.680171189290831535, 214.0920067884431148, 84.80113791807858092 ) ) ;
#16974=CARTESIAN_POINT ( 'NONE',  ( -2.517493886308901807, 199.4062855549015012, 95.90113791807857524 ) ) ;
#16975=CARTESIAN_POINT ( 'NONE',  ( -10.01549611932659722, 210.2015048109875011, 59.64886208192143613 ) ) ;
#16978=CARTESIAN_POINT ( 'NONE',  ( 9.736236675708031640, 199.9851607334238963, 58.29886208192143471 ) ) ;
#16982=CARTESIAN_POINT ( 'NONE',  ( -0.05014649552828365914, 215.4116977939061144, 42.24886208192143755 ) ) ;
#16987=DIRECTION ( 'NONE',  ( -0.2649168722799616349, 0.9642688156137669830, -0.002168413296787739895 ) ) ;
#16990=CARTESIAN_POINT ( 'NONE',  ( 8.000000000000008882, 206.9523078486586485, 59.00113791807857666 ) ) ;
#16992=CARTESIAN_POINT ( 'NONE',  ( -6.220909254589682469, 215.4770327129946850, 44.94886208192143329 ) ) ;
#16997=( LENGTH_UNIT ( ) NAMED_UNIT ( * ) SI_UNIT ( .MILLI., .METRE. ) );
#17000=CARTESIAN_POINT ( 'NONE',  ( 2.426778023690075337, 214.6231898156240447, 15.39886208192143613 ) ) ;
#17001=CARTESIAN_POINT ( 'NONE',  ( -9.984503880673473830, 210.2968891136704315, 60.65113791807856103 ) ) ;
#17002=CARTESIAN_POINT ( 'NONE',  ( -10.01549611932653860, 203.7984951890123284, 42.35113791807855677 ) ) ;
#17005=CARTESIAN_POINT ( 'NONE',  ( -3.135527875058821579, 197.5041725223112223, 14.90113791807856636 ) ) ;
#17006=CARTESIAN_POINT ( 'NONE',  ( -8.015496119326531499, 204.4483345814780364, 0.3511379180785659249 ) ) ;
#17011=CARTESIAN_POINT ( 'NONE',  ( -9.736236675707914401, 199.9851607334237542, 30.20113791807856529 ) ) ;
#17015=CARTESIAN_POINT ( 'NONE',  ( 6.139770520408368348, 198.4640165459539674, 77.45113791807854398 ) ) ;
#17016=CARTESIAN_POINT ( 'NONE',  ( -6.139770520408368348, 215.5359834540460042, 36.95113791807857240 ) ) ;
#17019=CARTESIAN_POINT ( 'NONE',  ( 9.736236675708031640, 199.9851607334238963, 1.298862081921434264 ) ) ;
#17020=CARTESIAN_POINT ( 'NONE',  ( -10.00000000000000711, 206.9523078486584495, 14.49886208192143577 ) ) ;
#17023=CARTESIAN_POINT ( 'NONE',  ( 12.01549611932652972, 210.8513442034534933, 49.85113791807857808 ) ) ;
#17024=CARTESIAN_POINT ( 'NONE',  ( -4.903702542908602524, 213.8346818373418898, 69.95113791807858661 ) ) ;
#17025=CARTESIAN_POINT ( 'NONE',  ( -8.062137200540822946, 201.0835637161416400, 35.19886208192143329 ) ) ;
#17030=CARTESIAN_POINT ( 'NONE',  ( 3.135527875058820690, 216.4958274776887492, 94.40113791807857524 ) ) ;
#17036=CARTESIAN_POINT ( 'NONE',  ( -4.984841277089726574, 200.2242689037092305, 27.05113791807857027 ) ) ;
#17039=CARTESIAN_POINT ( 'NONE',  ( 10.01549611932659545, 203.7984951890123853, 10.14886208192143613 ) ) ;
#17042=CARTESIAN_POINT ( 'NONE',  ( -2.426778023690262742, 214.6231898156240163, 46.10113791807857098 ) ) ;
#17046=CARTESIAN_POINT ( 'NONE',  ( -10.00000000000000711, 206.9523078486584495, 92.49886208192144466 ) ) ;
#17048=CARTESIAN_POINT ( 'NONE',  ( 6.139770520408368348, 198.4640165459539674, 32.45113791807856529 ) ) ;
#17051=CARTESIAN_POINT ( 'NONE',  ( -3.135527875058821579, 197.5041725223112223, 17.90113791807856458 ) ) ;
#17057=CARTESIAN_POINT ( 'NONE',  ( -10.01549611932653860, 203.7984951890123284, 90.35113791807857808 ) ) ;
#17061=CARTESIAN_POINT ( 'NONE',  ( 3.044812012440130555, 197.4746971517856764, 50.60113791807857808 ) ) ;
#17068=CARTESIAN_POINT ( 'NONE',  ( 11.98450388067348271, 203.0532714938637753, 23.15113791807856458 ) ) ;
#17076=CARTESIAN_POINT ( 'NONE',  ( 7.375838497908012492, 217.2372850707501186, 39.54886208192143471 ) ) ;
#17077=CARTESIAN_POINT ( 'NONE',  ( 10.01549611932653860, 210.2015048109876716, 4.851137918078563871 ) ) ;
#17078=CARTESIAN_POINT ( 'NONE',  ( -6.139770520408369237, 215.5359834540460042, 63.95113791807857950 ) ) ;
#17079=CARTESIAN_POINT ( 'NONE',  ( -4.903702542908436435, 200.1653181626580249, 26.04886208192144181 ) ) ;
#17083=CARTESIAN_POINT ( 'NONE',  ( -4.903702542908436435, 200.1653181626580249, 101.0488620819214276 ) ) ;
#17087=CARTESIAN_POINT ( 'NONE',  ( -7.984503880673488041, 209.6470497212046098, 42.65113791807857524 ) ) ;
#17088=DIRECTION ( 'NONE',  ( 0.5526942671207023539, 0.1536855300543050473, 0.8190908404712123891 ) ) ;
#17094=CARTESIAN_POINT ( 'NONE',  ( -3.044812012439970683, 197.4746971517856196, 58.89886208192143613 ) ) ;
#17099=CARTESIAN_POINT ( 'NONE',  ( -8.062137200540920645, 212.9164362838581894, 6.801137918078565825 ) ) ;
#17103=CARTESIAN_POINT ( 'NONE',  ( -4.984841277089891776, 213.7757310962905990, 80.94886208192143329 ) ) ;
#17108=CARTESIAN_POINT ( 'NONE',  ( -3.135527875058821579, 197.5041725223112223, 17.90113791807856458 ) ) ;
#17112=CARTESIAN_POINT ( 'NONE',  ( -9.736236675707914401, 199.9851607334237542, 90.20113791807857240 ) ) ;
#17115=CARTESIAN_POINT ( 'NONE',  ( 3.662846001189864698, 218.4274158808046593, 69.39886208192143613 ) ) ;
#17116=CARTESIAN_POINT ( 'NONE',  ( 8.118202686958138514, 201.1607312380088501, 76.29886208192144181 ) ) ;
#17118=CARTESIAN_POINT ( 'NONE',  ( -12.00000000000000711, 206.9523078486584780, 17.49886208192143400 ) ) ;
#17120=CARTESIAN_POINT ( 'NONE',  ( 10.01549611932653860, 210.2015048109876716, 28.85113791807855677 ) ) ;
#17121=DIRECTION ( 'NONE',  ( -0.2649168722799636333, 0.9642688156137663169, -0.002168413296789690158 ) ) ;
#17122=CARTESIAN_POINT ( 'NONE',  ( 3.044812012439969795, 216.5253028482143520, 90.39886208192143613 ) ) ;
#17126=CARTESIAN_POINT ( 'NONE',  ( -8.015496119326597224, 209.5516654185217362, 71.64886208192143613 ) ) ;
#17133=CARTESIAN_POINT ( 'NONE',  ( 7.984503880673485376, 204.3529502787953902, 74.15113791807857524 ) ) ;
#17136=CARTESIAN_POINT ( 'NONE',  ( -8.015496119326597224, 209.5516654185217362, 50.64886208192145034 ) ) ;
#17142=CARTESIAN_POINT ( 'NONE',  ( -11.98450388067348804, 210.9467285061362247, 60.65113791807856813 ) ) ;
#17144=CARTESIAN_POINT ( 'NONE',  ( -12.00000000000000711, 207.0476921513413515, 0.5011379180785653364 ) ) ;
#17145=CARTESIAN_POINT ( 'NONE',  ( 9.984503880673473830, 203.7031108863295401, 74.15113791807856103 ) ) ;
#17146=CARTESIAN_POINT ( 'NONE',  ( -11.98450388067341876, 203.0532714938636047, 38.34886208192142476 ) ) ;
#17147=CARTESIAN_POINT ( 'NONE',  ( 6.220909254589680693, 198.5229672870052582, 43.44886208192143329 ) ) ;
#17149=CARTESIAN_POINT ( 'NONE',  ( 0.05014649552807549926, 219.6175466908591716, 91.25113791807856956 ) ) ;
#17150=CARTESIAN_POINT ( 'NONE',  ( -2.517493886308901807, 199.4062855549015012, 98.90113791807858945 ) ) ;
#17151=CARTESIAN_POINT ( 'NONE',  ( -8.062137200540822946, 201.0835637161416400, 59.19886208192144039 ) ) ;
#17153=VERTEX_POINT ( 'NONE', #19503 ) ;
#17154=CARTESIAN_POINT ( 'NONE',  ( 12.01549611932659367, 203.1486557965466773, 67.14886208192143613 ) ) ;
#17157=CARTESIAN_POINT ( 'NONE',  ( -8.015496119326597224, 209.5516654185217362, 44.64886208192143613 ) ) ;
#17163=CARTESIAN_POINT ( 'NONE',  ( -2.517493886308901807, 199.4062855549015012, 56.90113791807858235 ) ) ;
#17165=CARTESIAN_POINT ( 'NONE',  ( 6.139770520408223575, 215.5359834540460611, 42.54886208192142050 ) ) ;
#17168=SURFACE_STYLE_FILL_AREA ( #30122 ) ;
#17171=CARTESIAN_POINT ( 'NONE',  ( 8.015496119326595448, 204.4483345814782638, 22.14886208192143613 ) ) ;
#17172=CARTESIAN_POINT ( 'NONE',  ( 9.984503880673470277, 203.7031108863295401, 65.15113791807856103 ) ) ;
#17174=CARTESIAN_POINT ( 'NONE',  ( -3.044812012440131443, 216.5253028482142952, 49.10113791807857808 ) ) ;
#17177=CARTESIAN_POINT ( 'NONE',  ( -6.139770520408369237, 215.5359834540460042, 15.95113791807856884 ) ) ;
#17178=CARTESIAN_POINT ( 'NONE',  ( -4.903702542908602524, 213.8346818373418898, 3.951137918078566624 ) ) ;
#17182=CARTESIAN_POINT ( 'NONE',  ( -12.00000000000000711, 207.0476921513413515, 24.50113791807856600 ) ) ;
#17184=CARTESIAN_POINT ( 'NONE',  ( -9.984503880673473830, 210.2968891136704315, 72.65113791807857524 ) ) ;
#17185=CARTESIAN_POINT ( 'NONE',  ( 3.044812012440130555, 197.4746971517856764, 53.60113791807857098 ) ) ;
#17188=CARTESIAN_POINT ( 'NONE',  ( 7.375838497908012492, 217.2372850707501186, 15.54886208192143826 ) ) ;
#17189=CARTESIAN_POINT ( 'NONE',  ( 0.05014649552828275014, 196.4853777576173002, 16.74886208192143400 ) ) ;
#17192=CARTESIAN_POINT ( 'NONE',  ( 0.05014649552807549926, 219.6175466908591716, 61.25113791807856245 ) ) ;
#17193=CARTESIAN_POINT ( 'NONE',  ( -4.903702542908602524, 213.8346818373418898, 66.95113791807857240 ) ) ;
#17194=CARTESIAN_POINT ( 'NONE',  ( -6.220909254589682469, 215.4770327129946850, 35.94886208192141908 ) ) ;
#17197=ORIENTED_EDGE ( 'NONE', *, *, #4602, .T. ) ;
#17199=CARTESIAN_POINT ( 'NONE',  ( 10.00000000000000711, 206.9523078486586201, 89.00113791807858377 ) ) ;
#17204=CARTESIAN_POINT ( 'NONE',  ( 4.903702542908601636, 200.1653181626581102, 35.45113791807857240 ) ) ;
#17206=CARTESIAN_POINT ( 'NONE',  ( 3.044812012439969795, 216.5253028482143520, 9.398862081921436129 ) ) ;
#17209=CARTESIAN_POINT ( 'NONE',  ( -4.984841277089726574, 200.2242689037092305, 54.05113791807856671 ) ) ;
#17212=CARTESIAN_POINT ( 'NONE',  ( 3.044812012439969795, 216.5253028482143520, 99.39886208192145034 ) ) ;
#17214=CARTESIAN_POINT ( 'NONE',  ( -6.139770520408369237, 215.5359834540460042, 33.95113791807855108 ) ) ;
#17217=CARTESIAN_POINT ( 'NONE',  ( -3.044812012440131443, 216.5253028482142952, 16.10113791807856742 ) ) ;
#17223=CARTESIAN_POINT ( 'NONE',  ( 3.662846001190051659, 195.5725841191953691, 2.601137918078566091 ) ) ;
#17226=CARTESIAN_POINT ( 'NONE',  ( 3.135527875058820690, 216.4958274776887492, 46.40113791807857524 ) ) ;
#17234=CARTESIAN_POINT ( 'NONE',  ( 9.736236675707914401, 214.0148392665762458, 31.70113791807856529 ) ) ;
#17238=CARTESIAN_POINT ( 'NONE',  ( -7.456977232089471386, 217.1783343296987709, 44.94886208192144039 ) ) ;
#17239=CARTESIAN_POINT ( 'NONE',  ( 8.118202686958039038, 212.8392687619912635, 4.701137918078565292 ) ) ;
#17240=CARTESIAN_POINT ( 'NONE',  ( -6.220909254589537696, 198.5229672870051161, 57.05113791807857382 ) ) ;
#17242=CARTESIAN_POINT ( 'NONE',  ( 2.426778023690075337, 214.6231898156240447, 27.39886208192143613 ) ) ;
#17246=CARTESIAN_POINT ( 'NONE',  ( -0.05014649552807731031, 198.5883022060938572, -0.2488620819214341084 ) ) ;
#17249=CARTESIAN_POINT ( 'NONE',  ( 3.662846001189864698, 218.4274158808046593, 87.39886208192143613 ) ) ;
#17256=CARTESIAN_POINT ( 'NONE',  ( -10.00000000000000711, 206.9523078486584495, 59.49886208192143755 ) ) ;
#17259=CARTESIAN_POINT ( 'NONE',  ( 9.984503880673470277, 203.7031108863295401, 2.151137918078565914 ) ) ;
#17263=CARTESIAN_POINT ( 'NONE',  ( -7.984503880673422316, 204.3529502787951628, 86.34886208192143897 ) ) ;
#17267=CARTESIAN_POINT ( 'NONE',  ( 12.01549611932659367, 203.1486557965466773, 85.14886208192143613 ) ) ;
#17269=CARTESIAN_POINT ( 'NONE',  ( -10.01549611932653860, 203.7984951890123000, 21.35113791807856387 ) ) ;
#17274=CARTESIAN_POINT ( 'NONE',  ( -7.456977232089304408, 196.8216656703010301, 84.05113791807858092 ) ) ;
#17277=CARTESIAN_POINT ( 'NONE',  ( -10.00000000000019362, 205.9534653805592654, 104.4507591396482127 ) ) ;
#17280=CARTESIAN_POINT ( 'NONE',  ( 7.375838497908012492, 217.2372850707501186, 66.54886208192144181 ) ) ;
#17281=CARTESIAN_POINT ( 'NONE',  ( 0.05014649552828275014, 196.4853777576173002, 73.74886208192144466 ) ) ;
#17282=CARTESIAN_POINT ( 'NONE',  ( 7.456977232089471386, 196.8216656703012006, 16.44886208192143684 ) ) ;
#17284=CARTESIAN_POINT ( 'NONE',  ( 10.01549611932653860, 210.2015048109876716, 34.85113791807856387 ) ) ;
#17288=CARTESIAN_POINT ( 'NONE',  ( -10.01549611932659722, 210.2015048109875011, 101.6488620819214361 ) ) ;
#17291=CARTESIAN_POINT ( 'NONE',  ( -1.474514954580286030E-14, 206.9977241638431167, -6.000000000000014211 ) ) ;
#17292=CARTESIAN_POINT ( 'NONE',  ( 8.015496119326595448, 204.4483345814782638, 82.14886208192143613 ) ) ;
#17303=CARTESIAN_POINT ( 'NONE',  ( 2.517493886308900919, 214.5937144450984420, 79.40113791807858945 ) ) ;
#17307=CARTESIAN_POINT ( 'NONE',  ( -8.015496119326597224, 209.5516654185217362, 53.64886208192143613 ) ) ;
#17313=CARTESIAN_POINT ( 'NONE',  ( -3.662846001190052991, 218.4274158808045740, 55.10113791807857808 ) ) ;
#17314=DIRECTION ( 'NONE',  ( -0.2649168722799616349, 0.9642688156137669830, -0.002168413296787739895 ) ) ;
#17316=CARTESIAN_POINT ( 'NONE',  ( -3.753561863808691168, 195.6020594897209435, 2.901137918078565470 ) ) ;
#17317=CARTESIAN_POINT ( 'NONE',  ( -3.044812012440131443, 216.5253028482142952, 82.10113791807857808 ) ) ;
#17319=CARTESIAN_POINT ( 'NONE',  ( 0.05014649552828288198, 194.3824533091408000, 37.74886208192143755 ) ) ;
#17320=CARTESIAN_POINT ( 'NONE',  ( -8.118202686958138514, 212.8392687619910930, 44.79886208192143471 ) ) ;
#17322=CARTESIAN_POINT ( 'NONE',  ( -3.753561863808691168, 195.6020594897209435, 86.90113791807857524 ) ) ;
#17324=CARTESIAN_POINT ( 'NONE',  ( -0.05014649552810635652, 196.4853777576173002, -0.2488620819214343305 ) ) ;
#17325=CARTESIAN_POINT ( 'NONE',  ( 3.135527875058981895, 197.5041725223112792, 73.59886208192143897 ) ) ;
#17329=CARTESIAN_POINT ( 'NONE',  ( -7.375838497908014268, 196.7627149292498530, 71.04886208192142760 ) ) ;
#17332=CARTESIAN_POINT ( 'NONE',  ( -4.903702542908436435, 200.1653181626580249, 47.04886208192144892 ) ) ;
#17340=AXIS2_PLACEMENT_3D ( 'NONE', #23955, #289, #13389 ) ;
#17341=CARTESIAN_POINT ( 'NONE',  ( 6.220909254589681581, 198.5229672870052582, 43.44886208192143329 ) ) ;
#17342=ORIENTED_EDGE ( 'NONE', *, *, #7897, .T. ) ;
#17347=CARTESIAN_POINT ( 'NONE',  ( 8.000000000000008882, 207.0476921513415220, 27.99886208192144110 ) ) ;
#17348=CARTESIAN_POINT ( 'NONE',  ( 9.984503880673470277, 203.7031108863295401, 59.15113791807858235 ) ) ;
#17349=CARTESIAN_POINT ( 'NONE',  ( -3.135527875058821579, 197.5041725223112223, 47.90113791807857524 ) ) ;
#17353=CARTESIAN_POINT ( 'NONE',  ( -6.220909254589537696, 198.5229672870051161, 18.05113791807856671 ) ) ;
#17354=CARTESIAN_POINT ( 'NONE',  ( 4.984841277089725686, 213.7757310962907411, 1.551137918078566047 ) ) ;
#17357=CARTESIAN_POINT ( 'NONE',  ( 11.98450388067348271, 203.0532714938637753, 32.15113791807856103 ) ) ;
#17359=CARTESIAN_POINT ( 'NONE',  ( 8.118202686958039038, 212.8392687619912635, 79.70113791807857240 ) ) ;
#17360=CARTESIAN_POINT ( 'NONE',  ( -3.044812012440131443, 216.5253028482142952, 46.10113791807857098 ) ) ;
#17363=CARTESIAN_POINT ( 'NONE',  ( 12.01549611932659367, 203.1486557965466773, 13.14886208192143613 ) ) ;
#17364=CARTESIAN_POINT ( 'NONE',  ( 6.139770520408223575, 215.5359834540460611, 18.54886208192143826 ) ) ;
#17367=CARTESIAN_POINT ( 'NONE',  ( 11.98450388067348271, 203.0532714938637753, 62.15113791807858945 ) ) ;
#17369=CARTESIAN_POINT ( 'NONE',  ( -0.05014649552807731031, 198.5883022060938572, 74.75113791807856956 ) ) ;
#17370=CARTESIAN_POINT ( 'NONE',  ( 3.044812012439969795, 216.5253028482143520, 33.39886208192143613 ) ) ;
#17379=CARTESIAN_POINT ( 'NONE',  ( 2.517493886308900919, 214.5937144450984420, 31.40113791807857879 ) ) ;
#17381=CARTESIAN_POINT ( 'NONE',  ( -0.05014649552828403384, 217.5146222423826714, 12.24886208192143755 ) ) ;
#17384=CARTESIAN_POINT ( 'NONE',  ( 2.517493886308900919, 214.5937144450984420, 49.40113791807856813 ) ) ;
#17388=CARTESIAN_POINT ( 'NONE',  ( -8.118202686958138514, 212.8392687619910930, 98.79886208192144181 ) ) ;
#17390=CARTESIAN_POINT ( 'NONE',  ( -6.139770520408369237, 215.5359834540460042, 36.95113791807857240 ) ) ;
#17391=CARTESIAN_POINT ( 'NONE',  ( -8.062137200540920645, 212.9164362838581894, 15.80113791807856849 ) ) ;
#17396=CARTESIAN_POINT ( 'NONE',  ( 8.062137200540920645, 201.0835637161417822, 101.3011379180785809 ) ) ;
#17399=CARTESIAN_POINT ( 'NONE',  ( 10.01549611932653860, 210.2015048109876716, 43.85113791807854966 ) ) ;
#17406=CARTESIAN_POINT ( 'NONE',  ( 9.680171189290831535, 199.9079932115568852, 29.30113791807857027 ) ) ;
#17408=CARTESIAN_POINT ( 'NONE',  ( 8.118202686958138514, 201.1607312380088501, 4.298862081921434708 ) ) ;
#17409=CARTESIAN_POINT ( 'NONE',  ( -9.658740382312574368, 207.9902050807892522, 102.7419814567561360 ) ) ;
#17411=CARTESIAN_POINT ( 'NONE',  ( 9.984503880673470277, 203.7031108863295401, 5.151137918078567246 ) ) ;
#17412=CARTESIAN_POINT ( 'NONE',  ( 3.044812012440130555, 197.4746971517856764, 65.60113791807857808 ) ) ;
#17413=CARTESIAN_POINT ( 'NONE',  ( 6.444103211790928043, 211.7408657792734061, 27.69886208192143684 ) ) ;
#17417=CARTESIAN_POINT ( 'NONE',  ( 4.903702542908601636, 200.1653181626581102, -0.5488620819214340418 ) ) ;
#17419=CARTESIAN_POINT ( 'NONE',  ( 9.680171189290716072, 214.0920067884432854, 90.69886208192143329 ) ) ;
#17426=CARTESIAN_POINT ( 'NONE',  ( -10.01549611932659722, 210.2015048109875011, 71.64886208192143613 ) ) ;
#17429=CARTESIAN_POINT ( 'NONE',  ( 10.01549611932653860, 210.2015048109876716, 7.851137918078566535 ) ) ;
#17432=CARTESIAN_POINT ( 'NONE',  ( 8.118202686958039038, 212.8392687619912635, 85.70113791807858661 ) ) ;
#17437=CARTESIAN_POINT ( 'NONE',  ( -11.98450388067341876, 203.0532714938636047, 89.34886208192143897 ) ) ;
#17439=CARTESIAN_POINT ( 'NONE',  ( -10.01549611932653860, 203.7984951890123000, 24.35113791807856387 ) ) ;
#17443=CARTESIAN_POINT ( 'NONE',  ( 12.00000000000000711, 206.9523078486586485, 86.00113791807856956 ) ) ;
#17448=CARTESIAN_POINT ( 'NONE',  ( 9.680171189290716072, 214.0920067884432854, 69.69886208192143329 ) ) ;
#17449=CARTESIAN_POINT ( 'NONE',  ( -6.139770520408224463, 198.4640165459539105, 74.04886208192144181 ) ) ;
#17450=CARTESIAN_POINT ( 'NONE',  ( -9.680171189290716072, 199.9079932115567146, 14.19886208192143684 ) ) ;
#17452=CARTESIAN_POINT ( 'NONE',  ( -6.139770520408369237, 215.5359834540460042, 36.95113791807857240 ) ) ;
#17454=CARTESIAN_POINT ( 'NONE',  ( 3.135527875058981895, 197.5041725223112792, 94.59886208192143897 ) ) ;
#17459=CARTESIAN_POINT ( 'NONE',  ( -6.500168698208244500, 211.6636982574061676, 83.79886208192144181 ) ) ;
#17466=CARTESIAN_POINT ( 'NONE',  ( -6.500168698208129925, 202.3363017425936050, 75.20113791807857240 ) ) ;
#17470=CARTESIAN_POINT ( 'NONE',  ( 8.015496119326595448, 204.4483345814782638, 49.14886208192145034 ) ) ;
#17477=CARTESIAN_POINT ( 'NONE',  ( -11.98450388067348804, 210.9467285061362247, 57.65113791807858945 ) ) ;
#17479=CARTESIAN_POINT ( 'NONE',  ( -3.044812012440131443, 216.5253028482142952, 100.1011379180785781 ) ) ;
#17480=CARTESIAN_POINT ( 'NONE',  ( 8.118202686958039038, 212.8392687619912635, 82.70113791807857240 ) ) ;
#17481=CARTESIAN_POINT ( 'NONE',  ( 9.736236675708031640, 199.9851607334238963, 46.29886208192144181 ) ) ;
#17482=CARTESIAN_POINT ( 'NONE',  ( 8.062137200540822946, 212.9164362838583315, 45.69886208192143329 ) ) ;
#17484=CARTESIAN_POINT ( 'NONE',  ( -12.01549611932652972, 203.1486557965464499, 87.35113791807857808 ) ) ;
#17486=CARTESIAN_POINT ( 'NONE',  ( -3.135527875058821579, 197.5041725223112223, 2.901137918078565914 ) ) ;
#17487=CARTESIAN_POINT ( 'NONE',  ( -8.062137200540822946, 201.0835637161416400, 71.19886208192144750 ) ) ;
#17489=ORIENTED_EDGE ( 'NONE', *, *, #21478, .T. ) ;
#17490=CARTESIAN_POINT ( 'NONE',  ( -0.05014649552828442242, 219.6175466908591716, 72.24886208192143044 ) ) ;
#17494=CARTESIAN_POINT ( 'NONE',  ( 4.903702542908435547, 213.8346818373419751, 51.54886208192144181 ) ) ;
#17504=CARTESIAN_POINT ( 'NONE',  ( -9.984503880673420539, 203.7031108863293980, 44.34886208192142476 ) ) ;
#17509=CARTESIAN_POINT ( 'NONE',  ( 2.517493886309087436, 199.4062855549015865, 28.59886208192143897 ) ) ;
#17510=CARTESIAN_POINT ( 'NONE',  ( -6.220909254589537696, 198.5229672870051161, 72.05113791807853829 ) ) ;
#17513=CARTESIAN_POINT ( 'NONE',  ( 0.05014649552810505201, 217.5146222423826714, 43.25113791807856956 ) ) ;
#17515=CARTESIAN_POINT ( 'NONE',  ( -10.01549611932653860, 203.7984951890123284, 18.35113791807856742 ) ) ;
#17517=CARTESIAN_POINT ( 'NONE',  ( 6.500168698208129925, 211.6636982574063381, 1.701137918078565958 ) ) ;
#17520=CARTESIAN_POINT ( 'NONE',  ( -7.456977232089304408, 196.8216656703010301, 30.05113791807857027 ) ) ;
#17523=CARTESIAN_POINT ( 'NONE',  ( 6.139770520408368348, 198.4640165459539674, 80.45113791807857240 ) ) ;
#17524=CARTESIAN_POINT ( 'NONE',  ( 8.062137200540920645, 201.0835637161417822, 47.30113791807857382 ) ) ;
#17528=CARTESIAN_POINT ( 'NONE',  ( -7.375838497908014268, 196.7627149292498530, 14.04886208192143471 ) ) ;
#17529=CARTESIAN_POINT ( 'NONE',  ( -6.220909254589682469, 215.4770327129947134, 20.94886208192143684 ) ) ;
#17533=CARTESIAN_POINT ( 'NONE',  ( 9.680171189290831535, 199.9079932115568852, 59.30113791807857382 ) ) ;
#17534=CARTESIAN_POINT ( 'NONE',  ( -2.426778023690262742, 214.6231898156240163, 79.10113791807857808 ) ) ;
#17535=CARTESIAN_POINT ( 'NONE',  ( -6.220909254589682469, 215.4770327129946850, 41.94886208192144039 ) ) ;
#17544=CARTESIAN_POINT ( 'NONE',  ( 8.000000000000008882, 206.9523078486586485, 35.00113791807857666 ) ) ;
#17545=CARTESIAN_POINT ( 'NONE',  ( 6.139770520408223575, 215.5359834540460611, 9.548862081921431155 ) ) ;
#17548=CARTESIAN_POINT ( 'NONE',  ( 8.000000000000008882, 206.9523078486586485, 56.00113791807857666 ) ) ;
#17553=CARTESIAN_POINT ( 'NONE',  ( -6.220909254589682469, 215.4770327129946850, 95.94886208192143329 ) ) ;
#17556=CARTESIAN_POINT ( 'NONE',  ( -6.220909254589537696, 198.5229672870051161, 36.05113791807857382 ) ) ;
#17558=CARTESIAN_POINT ( 'NONE',  ( 9.984503880673470277, 203.7031108863295401, 14.15113791807856458 ) ) ;
#17563=CARTESIAN_POINT ( 'NONE',  ( -11.98450388067348804, 210.9467285061362247, 0.6511379180785656917 ) ) ;
#17566=CARTESIAN_POINT ( 'NONE',  ( 6.220909254589536808, 215.4770327129947702, 46.55113791807856671 ) ) ;
#17573=CARTESIAN_POINT ( 'NONE',  ( 3.662846001190051659, 195.5725841191953691, 32.60113791807857098 ) ) ;
#17575=CARTESIAN_POINT ( 'NONE',  ( -0.05014649552828403384, 217.5146222423826714, 9.248862081921432221 ) ) ;
#17577=ORIENTED_EDGE ( 'NONE', *, *, #6042, .F. ) ;
#17579=CARTESIAN_POINT ( 'NONE',  ( -3.135527875058821579, 197.5041725223112223, 2.901137918078565914 ) ) ;
#17580=CARTESIAN_POINT ( 'NONE',  ( -8.062137200540920645, 212.9164362838581894, 57.80113791807857382 ) ) ;
#17583=CARTESIAN_POINT ( 'NONE',  ( -8.000000000000008882, 206.9523078486584780, 23.49886208192144110 ) ) ;
#17587=CARTESIAN_POINT ( 'NONE',  ( 6.500168698208129925, 211.6636982574063381, 4.701137918078565292 ) ) ;
#17589=CARTESIAN_POINT ( 'NONE',  ( -7.456977232089471386, 217.1783343296987709, 86.94886208192144750 ) ) ;
#17594=CARTESIAN_POINT ( 'NONE',  ( -0.05014649552810635652, 196.4853777576173002, 2.751137918078565114 ) ) ;
#17596=CARTESIAN_POINT ( 'NONE',  ( -10.00000000000000711, 206.9523078486584495, 74.49886208192144466 ) ) ;
#17599=CARTESIAN_POINT ( 'NONE',  ( 8.062137200540920645, 201.0835637161417822, 2.301137918078566269 ) ) ;
#17603=CARTESIAN_POINT ( 'NONE',  ( 8.062137200540920645, 201.0835637161417822, 92.30113791807858092 ) ) ;
#17606=CARTESIAN_POINT ( 'NONE',  ( 6.220909254589536808, 215.4770327129947702, 79.55113791807855250 ) ) ;
#17609=DIRECTION ( 'NONE',  ( -0.9891821073486152249, -0.1466927349985424900, -2.962715634069391535E-17 ) ) ;
#17610=CARTESIAN_POINT ( 'NONE',  ( -3.753561863808878130, 218.3979405102790281, 84.09886208192143897 ) ) ;
#17614=CARTESIAN_POINT ( 'NONE',  ( 10.01549611932653860, 210.2015048109876716, 25.85113791807856742 ) ) ;
#17618=CARTESIAN_POINT ( 'NONE',  ( 7.456977232089302632, 217.1783343296989131, 97.55113791807858092 ) ) ;
#17621=CARTESIAN_POINT ( 'NONE',  ( 10.01549611932659367, 203.7984951890124421, 82.14886208192143613 ) ) ;
#17622=CARTESIAN_POINT ( 'NONE',  ( -7.375838497908014268, 196.7627149292498530, 17.04886208192143471 ) ) ;
#17624=CARTESIAN_POINT ( 'NONE',  ( -3.135527875058821579, 197.5041725223112223, 35.90113791807856813 ) ) ;
#17626=CARTESIAN_POINT ( 'NONE',  ( -6.220909254589682469, 215.4770327129946850, 98.94886208192140487 ) ) ;
#17631=CARTESIAN_POINT ( 'NONE',  ( 8.015496119326595448, 204.4483345814782638, 76.14886208192143613 ) ) ;
#17640=CARTESIAN_POINT ( 'NONE',  ( -2.426778023690262742, 214.6231898156240163, 76.10113791807854966 ) ) ;
#17644=CARTESIAN_POINT ( 'NONE',  ( 0.05014649552828262524, 198.5883022060938572, 49.74886208192144466 ) ) ;
#17651=CARTESIAN_POINT ( 'NONE',  ( -3.662846001190052991, 218.4274158808045740, 61.10113791807857808 ) ) ;
#17653=CARTESIAN_POINT ( 'NONE',  ( -11.98450388067348804, 210.9467285061362247, 12.65113791807856636 ) ) ;
#17654=CARTESIAN_POINT ( 'NONE',  ( 10.01549611932653860, 210.2015048109876716, 76.85113791807857808 ) ) ;
#17656=CARTESIAN_POINT ( 'NONE',  ( 7.456977232089471386, 196.8216656703012006, 40.44886208192144039 ) ) ;
#17657=CARTESIAN_POINT ( 'NONE',  ( 3.044812012439969795, 216.5253028482143520, 60.39886208192143613 ) ) ;
#17659=CARTESIAN_POINT ( 'NONE',  ( -12.01549611932652972, 203.1486557965464499, 84.35113791807857808 ) ) ;
#17661=CARTESIAN_POINT ( 'NONE',  ( 9.984503880673470277, 203.7031108863295401, 8.151137918078564581 ) ) ;
#17662=CARTESIAN_POINT ( 'NONE',  ( -9.984503880673420539, 203.7031108863293980, 68.34886208192143897 ) ) ;
#17665=CARTESIAN_POINT ( 'NONE',  ( -7.456977232089471386, 217.1783343296987709, 68.94886208192144750 ) ) ;
#17669=CARTESIAN_POINT ( 'NONE',  ( 0.05014649552828262524, 198.5883022060938572, 55.74886208192144466 ) ) ;
#17678=CARTESIAN_POINT ( 'NONE',  ( 10.01549611932659545, 203.7984951890123853, 46.14886208192143613 ) ) ;
#17684=CARTESIAN_POINT ( 'NONE',  ( -8.015496119326597224, 209.5516654185217362, 20.64886208192143613 ) ) ;
#17685=CARTESIAN_POINT ( 'NONE',  ( -10.01549611932653860, 203.7984951890123284, 66.35113791807853545 ) ) ;
#17687=CARTESIAN_POINT ( 'NONE',  ( -8.118202686958039038, 201.1607312380087080, 51.20113791807857240 ) ) ;
#17689=CARTESIAN_POINT ( 'NONE',  ( 8.118202686958039038, 212.8392687619912635, 16.70113791807856529 ) ) ;
#17690=CARTESIAN_POINT ( 'NONE',  ( -4.903702542908602524, 213.8346818373418898, 6.951137918078566180 ) ) ;
#17693=CARTESIAN_POINT ( 'NONE',  ( 11.98450388067348271, 203.0532714938637753, 26.15113791807857169 ) ) ;
#17695=CARTESIAN_POINT ( 'NONE',  ( -6.220909254589537696, 198.5229672870051161, 72.05113791807853829 ) ) ;
#17696=CARTESIAN_POINT ( 'NONE',  ( -0.05014649552810635652, 196.4853777576173002, 53.75113791807857666 ) ) ;
#17698=DIRECTION ( 'NONE',  ( -0.9891821073486152249, -0.1466927349985424900, -2.962715634069391535E-17 ) ) ;
#17699=CARTESIAN_POINT ( 'NONE',  ( -7.456977232089471386, 217.1783343296987709, 14.94886208192143506 ) ) ;
#17700=CARTESIAN_POINT ( 'NONE',  ( -9.984503880673420539, 203.7031108863293980, 20.34886208192143187 ) ) ;
#17703=CARTESIAN_POINT ( 'NONE',  ( 7.375838497908181246, 196.7627149292499666, 56.45113791807857240 ) ) ;
#17704=CARTESIAN_POINT ( 'NONE',  ( -2.517493886308901807, 199.4062855549015012, 74.90113791807856103 ) ) ;
#17706=CARTESIAN_POINT ( 'NONE',  ( -8.062137200540822946, 201.0835637161416400, 44.19886208192143329 ) ) ;
#17717=CARTESIAN_POINT ( 'NONE',  ( 8.000000000000008882, 206.9523078486586485, 32.00113791807856956 ) ) ;
#17720=CARTESIAN_POINT ( 'NONE',  ( -8.062137200540822946, 201.0835637161416400, 11.19886208192143506 ) ) ;
#17723=CARTESIAN_POINT ( 'NONE',  ( 6.500168698208129925, 211.6636982574063381, 55.70113791807857240 ) ) ;
#17727=CARTESIAN_POINT ( 'NONE',  ( 9.984503880673420539, 210.2968891136705167, 102.8488620819214390 ) ) ;
#17729=CARTESIAN_POINT ( 'NONE',  ( -6.139770520408369237, 215.5359834540460042, 42.95113791807856529 ) ) ;
#17731=CARTESIAN_POINT ( 'NONE',  ( 9.984503880673470277, 203.7031108863295401, 17.15113791807856103 ) ) ;
#17732=CARTESIAN_POINT ( 'NONE',  ( -6.139770520408224463, 198.4640165459539105, 101.0488620819214276 ) ) ;
#17736=CARTESIAN_POINT ( 'NONE',  ( -0.05014649552807705357, 194.3824533091408000, -0.2488620819214344970 ) ) ;
#17739=CARTESIAN_POINT ( 'NONE',  ( 6.220909254589536808, 215.4770327129947702, 49.55113791807855250 ) ) ;
#17744=ORIENTED_EDGE ( 'NONE', *, *, #4518, .F. ) ;
#17745=CARTESIAN_POINT ( 'NONE',  ( 3.753561863808689836, 218.3979405102790565, 31.40113791807856813 ) ) ;
#17747=CARTESIAN_POINT ( 'NONE',  ( 6.139770520408223575, 215.5359834540460611, 9.548862081921431155 ) ) ;
#17750=CARTESIAN_POINT ( 'NONE',  ( -3.044812012440131443, 216.5253028482142952, 10.10113791807856565 ) ) ;
#17751=CARTESIAN_POINT ( 'NONE',  ( -10.00000000000000711, 207.0476921513413515, 57.50113791807856956 ) ) ;
#17753=CARTESIAN_POINT ( 'NONE',  ( -4.903702542908436435, 200.1653181626580249, 23.04886208192143826 ) ) ;
#17756=CARTESIAN_POINT ( 'NONE',  ( 7.984503880673485376, 204.3529502787953902, 2.151137918078566802 ) ) ;
#17757=CARTESIAN_POINT ( 'NONE',  ( 12.01549611932659367, 203.1486557965466773, 88.14886208192143613 ) ) ;
#17762=CARTESIAN_POINT ( 'NONE',  ( -3.135527875058821579, 197.5041725223112223, 2.901137918078565914 ) ) ;
#17764=CARTESIAN_POINT ( 'NONE',  ( -10.01549611932659722, 210.2015048109875011, 68.64886208192143613 ) ) ;
#17767=CARTESIAN_POINT ( 'NONE',  ( 3.044812012440130555, 197.4746971517856764, 14.60113791807856565 ) ) ;
#17771=CARTESIAN_POINT ( 'NONE',  ( -6.220909254589537696, 198.5229672870051161, 87.05113791807856671 ) ) ;
#17773=CARTESIAN_POINT ( 'NONE',  ( 3.044812012440130555, 197.4746971517856764, 77.60113791807857808 ) ) ;
#17776=CARTESIAN_POINT ( 'NONE',  ( 0.05014649552828288198, 194.3824533091408000, 91.74886208192144466 ) ) ;
#17778=CARTESIAN_POINT ( 'NONE',  ( -6.139770520408368348, 215.5359834540460042, 27.95113791807856529 ) ) ;
#17782=CARTESIAN_POINT ( 'NONE',  ( 7.375838497908181246, 196.7627149292499666, 92.45113791807857240 ) ) ;
#17787=CARTESIAN_POINT ( 'NONE',  ( -3.044812012439970683, 197.4746971517856196, 85.89886208192143613 ) ) ;
#17788=CARTESIAN_POINT ( 'NONE',  ( -11.98450388067341876, 203.0532714938636047, 23.34886208192143542 ) ) ;
#17790=CARTESIAN_POINT ( 'NONE',  ( -6.139770520408369237, 215.5359834540460042, 33.95113791807855108 ) ) ;
#17792=CARTESIAN_POINT ( 'NONE',  ( 3.044812012439969795, 216.5253028482143520, 102.3988620819214361 ) ) ;
#17797=CARTESIAN_POINT ( 'NONE',  ( 6.444103211790928043, 211.7408657792734061, 84.69886208192144750 ) ) ;
#17803=CARTESIAN_POINT ( 'NONE',  ( -8.000000000000008882, 207.0476921513413515, 60.50113791807857666 ) ) ;
#17807=CARTESIAN_POINT ( 'NONE',  ( 0.05014649552807626948, 215.4116977939061144, 79.25113791807856956 ) ) ;
#17811=CARTESIAN_POINT ( 'NONE',  ( 0.05014649552828262524, 198.5883022060938572, 67.74886208192143044 ) ) ;
#17812=CARTESIAN_POINT ( 'NONE',  ( -10.01549611932653860, 203.7984951890123000, 3.351137918078566091 ) ) ;
#17817=CARTESIAN_POINT ( 'NONE',  ( 9.736236675707914401, 214.0148392665762458, 70.70113791807857240 ) ) ;
#17818=CARTESIAN_POINT ( 'NONE',  ( 9.680171189290831535, 199.9079932115568852, 11.30113791807856671 ) ) ;
#17819=CARTESIAN_POINT ( 'NONE',  ( -10.01549611932653860, 203.7984951890123000, 84.35113791807856387 ) ) ;
#17820=CARTESIAN_POINT ( 'NONE',  ( 9.680171189290716072, 214.0920067884432854, 51.69886208192144039 ) ) ;
#17821=CARTESIAN_POINT ( 'NONE',  ( -8.062137200540822946, 201.0835637161416400, 62.19886208192143329 ) ) ;
#17823=CARTESIAN_POINT ( 'NONE',  ( 7.375838497908181246, 196.7627149292499666, 98.45113791807858661 ) ) ;
#17825=CARTESIAN_POINT ( 'NONE',  ( -8.118202686958039038, 201.1607312380087080, 0.2011379180785657361 ) ) ;
#17826=CARTESIAN_POINT ( 'NONE',  ( -8.118202686958138514, 212.8392687619910930, 65.79886208192144181 ) ) ;
#17830=CARTESIAN_POINT ( 'NONE',  ( 7.375838497908012492, 217.2372850707501186, 72.54886208192141339 ) ) ;
#17832=CARTESIAN_POINT ( 'NONE',  ( -8.062137200540920645, 212.9164362838581894, 93.80113791807858092 ) ) ;
#17835=CARTESIAN_POINT ( 'NONE',  ( -4.903702542908436435, 200.1653181626580249, 53.04886208192144181 ) ) ;
#17845=CARTESIAN_POINT ( 'NONE',  ( 8.062137200540822946, 212.9164362838583315, 54.69886208192143329 ) ) ;
#17853=CARTESIAN_POINT ( 'NONE',  ( -0.05014649552828365914, 215.4116977939061144, 21.24886208192143755 ) ) ;
#17855=CARTESIAN_POINT ( 'NONE',  ( -10.01549611932653860, 203.7984951890123284, 69.35113791807857808 ) ) ;
#17857=CARTESIAN_POINT ( 'NONE',  ( -3.044812012440131443, 216.5253028482142952, 52.10113791807857808 ) ) ;
#17859=CARTESIAN_POINT ( 'NONE',  ( 6.139770520408368348, 198.4640165459539674, 26.45113791807856884 ) ) ;
#17860=CARTESIAN_POINT ( 'NONE',  ( -0.05014649552807731031, 198.5883022060938572, 5.751137918078564226 ) ) ;
#17864=CARTESIAN_POINT ( 'NONE',  ( -12.00000000000000711, 207.0476921513413515, 36.50113791807857666 ) ) ;
#17868=CARTESIAN_POINT ( 'NONE',  ( 6.220909254589536808, 215.4770327129947702, 82.55113791807858092 ) ) ;
#17869=CARTESIAN_POINT ( 'NONE',  ( -10.01549611932653860, 203.7984951890123000, 51.35113791807857808 ) ) ;
#17870=AXIS2_PLACEMENT_3D ( 'NONE', #27529, #4536, #17314 ) ;
#17872=CARTESIAN_POINT ( 'NONE',  ( 0.05014649552828288198, 194.3824533091408000, 16.74886208192143755 ) ) ;
#17873=CARTESIAN_POINT ( 'NONE',  ( 6.139770520408223575, 215.5359834540460611, 30.54886208192143826 ) ) ;
#17876=CARTESIAN_POINT ( 'NONE',  ( 0.05014649552807549926, 219.6175466908591716, 58.25113791807856245 ) ) ;
#17877=CARTESIAN_POINT ( 'NONE',  ( 6.444103211791042618, 202.2591342207267644, 83.30113791807858092 ) ) ;
#17879=CARTESIAN_POINT ( 'NONE',  ( -0.05014649552828403384, 217.5146222423826714, 42.24886208192143755 ) ) ;
#17882=CARTESIAN_POINT ( 'NONE',  ( 12.01549611932659367, 203.1486557965466773, 46.14886208192143613 ) ) ;
#17891=CARTESIAN_POINT ( 'NONE',  ( 8.015496119326531499, 209.5516654185219636, 37.85113791807857098 ) ) ;
#17893=CARTESIAN_POINT ( 'NONE',  ( -0.05014649552828403384, 217.5146222423826714, 24.24886208192143044 ) ) ;
#17896=CARTESIAN_POINT ( 'NONE',  ( 4.984841277089725686, 213.7757310962907411, 61.55113791807858092 ) ) ;
#17900=CARTESIAN_POINT ( 'NONE',  ( 6.220909254589681581, 198.5229672870052582, 103.4488620819214049 ) ) ;
#17902=CARTESIAN_POINT ( 'NONE',  ( -0.05014649552810635652, 196.4853777576173002, 41.75113791807855534 ) ) ;
#17905=CARTESIAN_POINT ( 'NONE',  ( -10.00000000000000711, 207.0476921513413515, 30.50113791807856600 ) ) ;
#17906=CARTESIAN_POINT ( 'NONE',  ( 6.139770520408223575, 215.5359834540460611, 99.54886208192144181 ) ) ;
#17908=CARTESIAN_POINT ( 'NONE',  ( 2.426778023690075337, 214.6231898156240447, 87.39886208192143613 ) ) ;
#17912=CARTESIAN_POINT ( 'NONE',  ( -9.680171189290831535, 214.0920067884431148, 3.801137918078565825 ) ) ;
#17917=CARTESIAN_POINT ( 'NONE',  ( 3.135527875058820690, 216.4958274776887492, 55.40113791807857524 ) ) ;
#17922=CARTESIAN_POINT ( 'NONE',  ( -6.220909254589682469, 215.4770327129947134, 2.948862081921434619 ) ) ;
#17925=CARTESIAN_POINT ( 'NONE',  ( 7.375838497908181246, 196.7627149292499666, 26.45113791807857240 ) ) ;
#17927=CARTESIAN_POINT ( 'NONE',  ( -0.05014649552828403384, 217.5146222423826714, 15.24886208192143044 ) ) ;
#17930=VERTEX_POINT ( 'NONE', #13021 ) ;
#17932=CARTESIAN_POINT ( 'NONE',  ( -0.05014649552810635652, 196.4853777576173002, 11.75113791807856778 ) ) ;
#17933=CARTESIAN_POINT ( 'NONE',  ( 3.044812012440130555, 197.4746971517856764, 71.60113791807857808 ) ) ;
#17935=CARTESIAN_POINT ( 'NONE',  ( -8.015496119326597224, 209.5516654185217362, 29.64886208192143968 ) ) ;
#17938=CARTESIAN_POINT ( 'NONE',  ( 4.984841277089725686, 213.7757310962907411, 4.551137918078565825 ) ) ;
#17940=CARTESIAN_POINT ( 'NONE',  ( 12.00000000000000711, 207.0476921513415220, 87.99886208192144466 ) ) ;
#17945=CARTESIAN_POINT ( 'NONE',  ( 0.05014649552810505201, 217.5146222423826714, 4.251137918078566003 ) ) ;
#17946=CARTESIAN_POINT ( 'NONE',  ( -6.220909254589682469, 215.4770327129946850, 74.94886208192143329 ) ) ;
#17949=CARTESIAN_POINT ( 'NONE',  ( 8.118202686958039038, 212.8392687619912635, 10.70113791807856529 ) ) ;
#17953=CARTESIAN_POINT ( 'NONE',  ( 3.135527875058820690, 216.4958274776887492, 100.4011379180785752 ) ) ;
#17955=CARTESIAN_POINT ( 'NONE',  ( -9.984503880673473830, 210.2968891136704315, 72.65113791807857524 ) ) ;
#17959=CARTESIAN_POINT ( 'NONE',  ( -3.662846001189865142, 195.5725841191952838, 82.89886208192143613 ) ) ;
#17964=CARTESIAN_POINT ( 'NONE',  ( -0.05014649552807705357, 194.3824533091408000, 95.75113791807856956 ) ) ;
#17967=CARTESIAN_POINT ( 'NONE',  ( 8.062137200540822946, 212.9164362838583315, 87.69886208192144750 ) ) ;
#17968=CARTESIAN_POINT ( 'NONE',  ( 7.375838497908012492, 217.2372850707501186, 27.54886208192144181 ) ) ;
#17970=CARTESIAN_POINT ( 'NONE',  ( 3.135527875058820690, 216.4958274776887492, 43.40113791807856813 ) ) ;
#17972=CARTESIAN_POINT ( 'NONE',  ( 8.062137200540822946, 212.9164362838583315, 102.6988620819214475 ) ) ;
#17975=CARTESIAN_POINT ( 'NONE',  ( 2.426778023690075337, 214.6231898156240447, 84.39886208192143613 ) ) ;
#17980=CARTESIAN_POINT ( 'NONE',  ( -4.903702542908602524, 213.8346818373418898, 63.95113791807857240 ) ) ;
#17983=CARTESIAN_POINT ( 'NONE',  ( 0.05014649552807626948, 215.4116977939061144, 85.25113791807856956 ) ) ;
#17987=CARTESIAN_POINT ( 'NONE',  ( 6.500168698208244500, 202.3363017425938324, 61.29886208192144892 ) ) ;
#17996=CARTESIAN_POINT ( 'NONE',  ( -3.662846001190052991, 218.4274158808045740, 70.10113791807857808 ) ) ;
#17997=CARTESIAN_POINT ( 'NONE',  ( 10.00000000000000888, 206.9523078486588474, -0.9988620819213797075 ) ) ;
#17998=CARTESIAN_POINT ( 'NONE',  ( 11.98450388067348271, 203.0532714938637753, 14.15113791807856991 ) ) ;
#17999=CARTESIAN_POINT ( 'NONE',  ( 10.00000000000000711, 206.9523078486586201, 86.00113791807858377 ) ) ;
#18000=CARTESIAN_POINT ( 'NONE',  ( -12.00000000000000711, 206.9523078486584780, 56.49886208192144466 ) ) ;
#18001=CARTESIAN_POINT ( 'NONE',  ( 3.044812012439969795, 216.5253028482143520, 54.39886208192143613 ) ) ;
#18003=CARTESIAN_POINT ( 'NONE',  ( 7.375838497908181246, 196.7627149292499666, 92.45113791807857240 ) ) ;
#18005=CARTESIAN_POINT ( 'NONE',  ( -6.139770520408369237, 215.5359834540460042, 0.9511379180785658471 ) ) ;
#18006=CARTESIAN_POINT ( 'NONE',  ( 10.01549611932659545, 203.7984951890123853, 70.14886208192139350 ) ) ;
#18008=CARTESIAN_POINT ( 'NONE',  ( -0.05014649552828442242, 219.6175466908591716, 81.24886208192143044 ) ) ;
#18009=CARTESIAN_POINT ( 'NONE',  ( -9.984503880673473830, 210.2968891136704315, 93.65113791807857524 ) ) ;
#18012=CARTESIAN_POINT ( 'NONE',  ( 8.000000000000008882, 207.0476921513415220, 54.99886208192145176 ) ) ;
#18020=CARTESIAN_POINT ( 'NONE',  ( -3.135527875058982783, 216.4958274776886924, 48.09886208192143187 ) ) ;
#18024=CARTESIAN_POINT ( 'NONE',  ( -0.05014649552828365914, 215.4116977939061144, 39.24886208192144466 ) ) ;
#18025=CARTESIAN_POINT ( 'NONE',  ( 6.220909254589536808, 215.4770327129947702, 67.55113791807853829 ) ) ;
#18027=CARTESIAN_POINT ( 'NONE',  ( 6.139770520408368348, 198.4640165459539674, 56.45113791807857950 ) ) ;
#18028=CARTESIAN_POINT ( 'NONE',  ( 6.220909254589536808, 215.4770327129947702, 31.55113791807857382 ) ) ;
#18029=CARTESIAN_POINT ( 'NONE',  ( 6.500168698208129925, 211.6636982574063381, 13.70113791807856707 ) ) ;
#18033=CARTESIAN_POINT ( 'NONE',  ( 9.680171189290831535, 199.9079932115568852, 35.30113791807856671 ) ) ;
#18035=CARTESIAN_POINT ( 'NONE',  ( -8.062137200540920645, 212.9164362838581894, 81.80113791807858092 ) ) ;
#18037=CARTESIAN_POINT ( 'NONE',  ( -8.062137200540920645, 212.9164362838581894, 57.80113791807857382 ) ) ;
#18039=CARTESIAN_POINT ( 'NONE',  ( -9.736236675708031640, 214.0148392665760753, 26.79886208192143826 ) ) ;
#18040=CARTESIAN_POINT ( 'NONE',  ( 3.135527875058981895, 197.5041725223112792, 31.59886208192143187 ) ) ;
#18043=CARTESIAN_POINT ( 'NONE',  ( -9.736236675707914401, 199.9851607334237542, 63.20113791807857240 ) ) ;
#18044=CARTESIAN_POINT ( 'NONE',  ( -2.426778023690262742, 214.6231898156240163, 76.10113791807854966 ) ) ;
#18045=CARTESIAN_POINT ( 'NONE',  ( 8.062137200540822946, 212.9164362838583315, 36.69886208192143329 ) ) ;
#18049=CARTESIAN_POINT ( 'NONE',  ( -11.98450388067341876, 203.0532714938636047, 53.34886208192144608 ) ) ;
#18055=CARTESIAN_POINT ( 'NONE',  ( -8.000000000000008882, 207.0476921513413515, 39.50113791807857666 ) ) ;
#18057=CARTESIAN_POINT ( 'NONE',  ( 3.044812012439969795, 216.5253028482143520, 21.39886208192143613 ) ) ;
#18062=CARTESIAN_POINT ( 'NONE',  ( 2.517493886309087436, 199.4062855549015865, 1.598862081921434974 ) ) ;
#18064=CARTESIAN_POINT ( 'NONE',  ( -10.00000000000000711, 207.0476921513413515, 42.50113791807856956 ) ) ;
#18067=CARTESIAN_POINT ( 'NONE',  ( 3.044812012440130555, 197.4746971517856764, 29.60113791807856742 ) ) ;
#18070=CARTESIAN_POINT ( 'NONE',  ( -4.984841277089891776, 213.7757310962905990, 77.94886208192143329 ) ) ;
#18075=CARTESIAN_POINT ( 'NONE',  ( -11.98450388067348804, 210.9467285061362247, 12.65113791807856636 ) ) ;
#18078=CARTESIAN_POINT ( 'NONE',  ( -9.984503880673473830, 210.2968891136704315, 57.65113791807858235 ) ) ;
#18082=CARTESIAN_POINT ( 'NONE',  ( 9.984503880673420539, 210.2968891136705736, 3.848862081921434086 ) ) ;
#18085=CARTESIAN_POINT ( 'NONE',  ( -7.456977232089304408, 196.8216656703010301, 39.05113791807855961 ) ) ;
#18087=CARTESIAN_POINT ( 'NONE',  ( 6.220909254589681581, 198.5229672870052582, 7.448862081921433287 ) ) ;
#18092=CARTESIAN_POINT ( 'NONE',  ( -3.135527875058821579, 197.5041725223112223, 11.90113791807856636 ) ) ;
#18093=CARTESIAN_POINT ( 'NONE',  ( 0.05014649552810505201, 217.5146222423826714, 70.25113791807858377 ) ) ;
#18095=CARTESIAN_POINT ( 'NONE',  ( 7.984503880673422316, 209.6470497212048372, 30.84886208192143542 ) ) ;
#18099=CARTESIAN_POINT ( 'NONE',  ( -2.426778023690262742, 214.6231898156240163, 16.10113791807856742 ) ) ;
#18102=CARTESIAN_POINT ( 'NONE',  ( -12.00000000000000711, 206.9523078486584780, 98.49886208192143044 ) ) ;
#18107=CARTESIAN_POINT ( 'NONE',  ( 9.984503880673470277, 203.7031108863295401, 11.15113791807856636 ) ) ;
#18108=CARTESIAN_POINT ( 'NONE',  ( 6.220909254589681581, 198.5229672870052582, 79.44886208192143329 ) ) ;
#18111=CARTESIAN_POINT ( 'NONE',  ( -6.139770520408369237, 215.5359834540460042, 9.951137918078567068 ) ) ;
#18113=AXIS2_PLACEMENT_3D ( 'NONE', #11414, #27076, #16679 ) ;
#18115=CARTESIAN_POINT ( 'NONE',  ( 8.062137200540920645, 201.0835637161417822, 95.30113791807858092 ) ) ;
#18117=CARTESIAN_POINT ( 'NONE',  ( -8.062137200540920645, 212.9164362838581894, 84.80113791807856671 ) ) ;
#18120=CARTESIAN_POINT ( 'NONE',  ( 9.680171189290716072, 214.0920067884432854, 96.69886208192144750 ) ) ;
#18126=CARTESIAN_POINT ( 'NONE',  ( 12.00000000000000711, 206.9523078486586485, 95.00113791807856956 ) ) ;
#18128=CARTESIAN_POINT ( 'NONE',  ( -10.98061573408523195, 206.7617422472766009, 103.7067083923456039 ) ) ;
#18130=CARTESIAN_POINT ( 'NONE',  ( 3.135527875058981895, 197.5041725223112792, 88.59886208192143897 ) ) ;
#18131=CARTESIAN_POINT ( 'NONE',  ( -3.662846001189865142, 195.5725841191952838, 25.89886208192143613 ) ) ;
#18133=CARTESIAN_POINT ( 'NONE',  ( 6.220909254589536808, 215.4770327129947702, 37.55113791807856671 ) ) ;
#18135=CARTESIAN_POINT ( 'NONE',  ( -0.05014649552828365914, 215.4116977939061144, 6.248862081921434886 ) ) ;
#18138=AXIS2_PLACEMENT_3D ( 'NONE', #1967, #9627, #25303 ) ;
#18141=CARTESIAN_POINT ( 'NONE',  ( -4.984841277089891776, 213.7757310962905990, 89.94886208192144750 ) ) ;
#18145=CARTESIAN_POINT ( 'NONE',  ( -4.984841277089726574, 200.2242689037092305, 30.05113791807857027 ) ) ;
#18151=EDGE_CURVE ( 'NONE', #11012, #28735, #16243, .T. ) ;
#18154=CARTESIAN_POINT ( 'NONE',  ( -8.015496119326531499, 204.4483345814780364, 90.35113791807857808 ) ) ;
#18158=CARTESIAN_POINT ( 'NONE',  ( -6.500168698208244500, 211.6636982574061676, 62.79886208192144892 ) ) ;
#18162=CARTESIAN_POINT ( 'NONE',  ( -6.220909254589537696, 198.5229672870051445, 3.051137918078565381 ) ) ;
#18166=CARTESIAN_POINT ( 'NONE',  ( 0.05014649552807549926, 219.6175466908591716, 67.25113791807856956 ) ) ;
#18167=LINE ( 'NONE', #17997, #24406 ) ;
#18168=CARTESIAN_POINT ( 'NONE',  ( 3.662846001190051659, 195.5725841191953691, 5.601137918078566535 ) ) ;
#18169=CARTESIAN_POINT ( 'NONE',  ( -3.044812012440131443, 216.5253028482142952, 91.10113791807857808 ) ) ;
#18170=CARTESIAN_POINT ( 'NONE',  ( 3.662846001189864698, 218.4274158808046593, 51.39886208192144323 ) ) ;
#18171=CARTESIAN_POINT ( 'NONE',  ( -3.044812012439970683, 197.4746971517856196, 55.89886208192143613 ) ) ;
#18173=CARTESIAN_POINT ( 'NONE',  ( 0.05014649552807549926, 219.6175466908591716, 100.2511379180785696 ) ) ;
#18175=CARTESIAN_POINT ( 'NONE',  ( -3.135527875058821579, 197.5041725223112223, 17.90113791807856458 ) ) ;
#18177=CARTESIAN_POINT ( 'NONE',  ( 6.220909254589681581, 198.5229672870052582, 76.44886208192143329 ) ) ;
#18179=CARTESIAN_POINT ( 'NONE',  ( 9.736236675708031640, 199.9851607334238963, 79.29886208192144181 ) ) ;
#18180=CARTESIAN_POINT ( 'NONE',  ( -0.05014649552810635652, 196.4853777576173002, 95.75113791807856956 ) ) ;
#18183=CARTESIAN_POINT ( 'NONE',  ( -2.426778023690076225, 199.3768101843759553, 52.89886208192144323 ) ) ;
#18190=CARTESIAN_POINT ( 'NONE',  ( -3.044812012439970683, 197.4746971517856196, 52.89886208192143613 ) ) ;
#18196=CARTESIAN_POINT ( 'NONE',  ( 8.000000000000008882, 207.0476921513415220, 30.99886208192143400 ) ) ;
#18198=CARTESIAN_POINT ( 'NONE',  ( 0.05014649552810505201, 217.5146222423826714, 73.25113791807855534 ) ) ;
#18200=CARTESIAN_POINT ( 'NONE',  ( -3.044812012440131443, 216.5253028482142952, 58.10113791807857808 ) ) ;
#18201=CARTESIAN_POINT ( 'NONE',  ( -8.062137200540920645, 212.9164362838581894, 27.80113791807856671 ) ) ;
#18202=CARTESIAN_POINT ( 'NONE',  ( 6.444103211791042618, 202.2591342207267644, 17.30113791807856671 ) ) ;
#18206=CARTESIAN_POINT ( 'NONE',  ( 12.01549611932652972, 210.8513442034534933, 34.85113791807856387 ) ) ;
#18208=CARTESIAN_POINT ( 'NONE',  ( 6.139770520408368348, 198.4640165459539674, 83.45113791807858661 ) ) ;
#18209=CARTESIAN_POINT ( 'NONE',  ( 10.00000000000000711, 206.9523078486586201, 56.00113791807856956 ) ) ;
#18211=CARTESIAN_POINT ( 'NONE',  ( 3.662846001189864698, 218.4274158808046593, 24.39886208192143258 ) ) ;
#18212=CARTESIAN_POINT ( 'NONE',  ( 6.139770520408223575, 215.5359834540460611, 24.54886208192143471 ) ) ;
#18214=CARTESIAN_POINT ( 'NONE',  ( 12.01549611932652972, 210.8513442034534933, 64.85113791807857808 ) ) ;
#18215=CARTESIAN_POINT ( 'NONE',  ( -6.444103211791042618, 211.7408657792732356, 87.80113791807858092 ) ) ;
#18216=CARTESIAN_POINT ( 'NONE',  ( 6.220909254589681581, 198.5229672870052582, 40.44886208192141908 ) ) ;
#18219=VERTEX_POINT ( 'NONE', #11463 ) ;
#18220=CARTESIAN_POINT ( 'NONE',  ( 12.01549611932659367, 203.1486557965466773, 55.14886208192143613 ) ) ;
#18226=CARTESIAN_POINT ( 'NONE',  ( 4.903702542908601636, 200.1653181626581102, 41.45113791807857240 ) ) ;
#18229=CARTESIAN_POINT ( 'NONE',  ( 10.00000000000000711, 207.0476921513415220, 21.99886208192143755 ) ) ;
#18235=CARTESIAN_POINT ( 'NONE',  ( 8.000000000000008882, 207.0476921513415220, 6.998862081921435774 ) ) ;
#18236=CARTESIAN_POINT ( 'NONE',  ( 3.044812012440130555, 197.4746971517856764, 41.60113791807857808 ) ) ;
#18238=CARTESIAN_POINT ( 'NONE',  ( 0.05014649552810505201, 217.5146222423826714, 28.25113791807855890 ) ) ;
#18241=CARTESIAN_POINT ( 'NONE',  ( -2.426778023690076225, 199.3768101843759553, 94.89886208192145034 ) ) ;
#18245=CARTESIAN_POINT ( 'NONE',  ( -3.753561863808691168, 195.6020594897209435, 8.901137918078566358 ) ) ;
#18248=CARTESIAN_POINT ( 'NONE',  ( -3.135527875058821579, 197.5041725223112223, 53.90113791807857524 ) ) ;
#18254=CARTESIAN_POINT ( 'NONE',  ( -9.680171189290831535, 214.0920067884431148, 39.80113791807857382 ) ) ;
#18256=CARTESIAN_POINT ( 'NONE',  ( -3.135527875058982783, 216.4958274776886924, 12.09886208192143542 ) ) ;
#18259=CARTESIAN_POINT ( 'NONE',  ( 3.135527875058820690, 216.4958274776887492, 67.40113791807857524 ) ) ;
#18261=CARTESIAN_POINT ( 'NONE',  ( 4.903702542908435547, 213.8346818373419751, 36.54886208192144892 ) ) ;
#18263=ORIENTED_EDGE ( 'NONE', *, *, #30736, .F. ) ;
#18264=CARTESIAN_POINT ( 'NONE',  ( 8.015496119326531499, 209.5516654185219636, 16.85113791807856742 ) ) ;
#18267=CARTESIAN_POINT ( 'NONE',  ( -12.00000000000000711, 206.9523078486584780, 95.49886208192144466 ) ) ;
#18272=CARTESIAN_POINT ( 'NONE',  ( 9.984503880673470277, 203.7031108863295401, 8.151137918078564581 ) ) ;
#18273=CARTESIAN_POINT ( 'NONE',  ( -0.05014649552828403384, 217.5146222423826714, 78.24886208192144466 ) ) ;
#18276=CARTESIAN_POINT ( 'NONE',  ( 6.220909254589536808, 215.4770327129947702, 16.55113791807857027 ) ) ;
#18280=CARTESIAN_POINT ( 'NONE',  ( -0.05014649552810635652, 196.4853777576173002, 98.75113791807854113 ) ) ;
#18282=CARTESIAN_POINT ( 'NONE',  ( -0.05014649552810635652, 196.4853777576173002, 83.75113791807856956 ) ) ;
#18285=CARTESIAN_POINT ( 'NONE',  ( -7.375838497908014268, 196.7627149292498530, 101.0488620819214276 ) ) ;
#18290=CARTESIAN_POINT ( 'NONE',  ( 0.05014649552807549926, 219.6175466908591716, 100.2511379180785696 ) ) ;
#18294=CARTESIAN_POINT ( 'NONE',  ( -8.118202686958138514, 212.8392687619910930, 83.79886208192144181 ) ) ;
#18295=CARTESIAN_POINT ( 'NONE',  ( 3.662846001189864698, 218.4274158808046593, 24.39886208192143258 ) ) ;
#18297=CARTESIAN_POINT ( 'NONE',  ( -3.044812012440131443, 216.5253028482142952, 46.10113791807857098 ) ) ;
#18298=ADVANCED_FACE ( 'NONE', ( #29862 ), #30711, .T. ) ;
#18300=CARTESIAN_POINT ( 'NONE',  ( -6.444103211790928043, 202.2591342207265939, 8.198862081921436840 ) ) ;
#18304=CARTESIAN_POINT ( 'NONE',  ( 7.984503880673422316, 209.6470497212048372, 90.84886208192142476 ) ) ;
#18306=CARTESIAN_POINT ( 'NONE',  ( -6.500168698208129925, 202.3363017425936050, 27.20113791807857240 ) ) ;
#18313=CARTESIAN_POINT ( 'NONE',  ( -8.015496119326531499, 204.4483345814780364, 87.35113791807857808 ) ) ;
#18316=CARTESIAN_POINT ( 'NONE',  ( 0.05014649552828262524, 198.5883022060938572, 64.74886208192143044 ) ) ;
#18321=CARTESIAN_POINT ( 'NONE',  ( 10.00000000000000711, 206.9523078486586201, 5.001137918078565114 ) ) ;
#18325=CARTESIAN_POINT ( 'NONE',  ( -12.01549611932652972, 203.1486557965464499, 66.35113791807857808 ) ) ;
#18327=CARTESIAN_POINT ( 'NONE',  ( 0.05014649552807549926, 219.6175466908591716, 13.25113791807856423 ) ) ;
#18329=CARTESIAN_POINT ( 'NONE',  ( 10.00000000000000711, 206.9523078486586201, 92.00113791807858377 ) ) ;
#18332=CARTESIAN_POINT ( 'NONE',  ( 9.680171189290716072, 214.0920067884432854, 48.69886208192144039 ) ) ;
#18333=CARTESIAN_POINT ( 'NONE',  ( -3.135527875058982783, 216.4958274776886924, 60.09886208192143897 ) ) ;
#18334=CARTESIAN_POINT ( 'NONE',  ( 11.98450388067348271, 203.0532714938637753, 101.1511379180785895 ) ) ;
#18336=CARTESIAN_POINT ( 'NONE',  ( -10.00000000000000711, 207.0476921513413515, 15.50113791807856600 ) ) ;
#18337=EDGE_CURVE ( 'NONE', #17930, #16872, #1284, .T. ) ;
#18338=CARTESIAN_POINT ( 'NONE',  ( 8.062137200540822946, 212.9164362838583315, 78.69886208192143329 ) ) ;
#18340=CARTESIAN_POINT ( 'NONE',  ( -7.456977232089471386, 217.1783343296987709, 80.94886208192143329 ) ) ;
#18341=CARTESIAN_POINT ( 'NONE',  ( 10.00000000000000711, 206.9523078486586201, 98.00113791807856956 ) ) ;
#18344=CARTESIAN_POINT ( 'NONE',  ( -8.000000000000008882, 206.9523078486584780, 62.49886208192144466 ) ) ;
#18353=CARTESIAN_POINT ( 'NONE',  ( -6.220909254589682469, 215.4770327129946850, 47.94886208192144039 ) ) ;
#18360=CARTESIAN_POINT ( 'NONE',  ( 7.984503880673422316, 209.6470497212048372, 30.84886208192143542 ) ) ;
#18361=CARTESIAN_POINT ( 'NONE',  ( 8.118202686958039038, 212.8392687619912635, 82.70113791807857240 ) ) ;
#18363=CARTESIAN_POINT ( 'NONE',  ( 3.044812012440130555, 197.4746971517856764, 53.60113791807857098 ) ) ;
#18364=EDGE_CURVE ( 'NONE', #16076, #33380, #24656, .T. ) ;
#18365=CARTESIAN_POINT ( 'NONE',  ( -3.135527875058821579, 197.5041725223112223, 29.90113791807856813 ) ) ;
#18366=CARTESIAN_POINT ( 'NONE',  ( 2.517493886308900919, 214.5937144450984420, 10.40113791807856636 ) ) ;
#18370=CARTESIAN_POINT ( 'NONE',  ( 12.01549611932652972, 210.8513442034534933, 37.85113791807856387 ) ) ;
#18373=CARTESIAN_POINT ( 'NONE',  ( 3.044812012440130555, 197.4746971517856764, 89.60113791807857808 ) ) ;
#18374=CARTESIAN_POINT ( 'NONE',  ( -6.139770520408368348, 215.5359834540460042, 57.95113791807855819 ) ) ;
#18376=CARTESIAN_POINT ( 'NONE',  ( -7.375838497908014268, 196.7627149292498530, 26.04886208192144181 ) ) ;
#18377=CARTESIAN_POINT ( 'NONE',  ( -6.139770520408224463, 198.4640165459539105, 32.04886208192143471 ) ) ;
#18379=CARTESIAN_POINT ( 'NONE',  ( 9.736236675707914401, 214.0148392665762458, 70.70113791807857240 ) ) ;
#18380=CARTESIAN_POINT ( 'NONE',  ( -4.903702542908602524, 213.8346818373418898, 90.95113791807855819 ) ) ;
#18381=CARTESIAN_POINT ( 'NONE',  ( 0.05014649552828275708, 196.4853777576173002, 52.74886208192143044 ) ) ;
#18385=CARTESIAN_POINT ( 'NONE',  ( 0.05014649552828288198, 194.3824533091408000, 52.74886208192143755 ) ) ;
#18390=CARTESIAN_POINT ( 'NONE',  ( 6.500168698208129925, 211.6636982574063381, 46.70113791807857240 ) ) ;
#18394=CARTESIAN_POINT ( 'NONE',  ( -0.05014649552828403384, 217.5146222423826714, 27.24886208192142689 ) ) ;
#18400=CARTESIAN_POINT ( 'NONE',  ( -4.903702542908436435, 200.1653181626580249, 5.048862081921433820 ) ) ;
#18401=CARTESIAN_POINT ( 'NONE',  ( -9.984503880673473830, 210.2968891136704315, 45.65113791807855392 ) ) ;
#18403=CARTESIAN_POINT ( 'NONE',  ( 6.220909254589536808, 215.4770327129947702, 25.55113791807856671 ) ) ;
#18404=CARTESIAN_POINT ( 'NONE',  ( -0.05014649552828402690, 217.5146222423826714, 99.24886208192144466 ) ) ;
#18407=CARTESIAN_POINT ( 'NONE',  ( -6.500168698208244500, 211.6636982574061676, 89.79886208192142760 ) ) ;
#18411=CARTESIAN_POINT ( 'NONE',  ( -7.456977232089304408, 196.8216656703010301, 12.05113791807856849 ) ) ;
#18414=CARTESIAN_POINT ( 'NONE',  ( -6.139770520408369237, 215.5359834540460042, 51.95113791807857950 ) ) ;
#18415=CARTESIAN_POINT ( 'NONE',  ( -8.062137200540920645, 212.9164362838581894, 30.80113791807856671 ) ) ;
#18418=CARTESIAN_POINT ( 'NONE',  ( 10.00000000000000711, 207.0476921513415220, 0.9988620819214341084 ) ) ;
#18421=CARTESIAN_POINT ( 'NONE',  ( -11.98450388067348804, 210.9467285061362247, 42.65113791807856813 ) ) ;
#18425=CARTESIAN_POINT ( 'NONE',  ( 6.220909254589681581, 198.5229672870052582, 22.44886208192143329 ) ) ;
#18429=CARTESIAN_POINT ( 'NONE',  ( 9.984503880673470277, 203.7031108863295401, 71.15113791807857524 ) ) ;
#18435=CARTESIAN_POINT ( 'NONE',  ( 2.426778023690261410, 199.3768101843759837, 17.60113791807856742 ) ) ;
#18436=CARTESIAN_POINT ( 'NONE',  ( 0.05014649552828288198, 194.3824533091408000, 100.7488620819214304 ) ) ;
#18441=CARTESIAN_POINT ( 'NONE',  ( -6.139770520408369237, 215.5359834540460042, 12.95113791807856352 ) ) ;
#18443=CARTESIAN_POINT ( 'NONE',  ( 6.220909254589681581, 198.5229672870052582, 85.44886208192140487 ) ) ;
#18446=CARTESIAN_POINT ( 'NONE',  ( -8.062137200540920645, 212.9164362838581894, 12.80113791807856671 ) ) ;
#18451=CARTESIAN_POINT ( 'NONE',  ( 3.044812012440130555, 197.4746971517856764, 95.60113791807857808 ) ) ;
#18453=CARTESIAN_POINT ( 'NONE',  ( -8.118202686958039038, 201.1607312380087080, 87.20113791807858661 ) ) ;
#18456=CARTESIAN_POINT ( 'NONE',  ( 7.375838497908012492, 217.2372850707501186, 93.54886208192142760 ) ) ;
#18460=DIRECTION ( 'NONE',  ( 0.5526942671207055735, 0.1536855300543024383, 0.8190908404712107238 ) ) ;
#18462=CARTESIAN_POINT ( 'NONE',  ( -7.375838497908014268, 196.7627149292498530, 2.048862081921434264 ) ) ;
#18466=CARTESIAN_POINT ( 'NONE',  ( 0.05014649552828275014, 196.4853777576173002, 94.74886208192141623 ) ) ;
#18467=CARTESIAN_POINT ( 'NONE',  ( -3.753561863808878130, 218.3979405102790281, 27.09886208192143897 ) ) ;
#18471=CARTESIAN_POINT ( 'NONE',  ( -10.00000000000000711, 207.0476921513413515, 45.50113791807857666 ) ) ;
#18473=CARTESIAN_POINT ( 'NONE',  ( 8.118202686958138514, 201.1607312380088501, 103.2988620819214418 ) ) ;
#18477=CARTESIAN_POINT ( 'NONE',  ( 7.984503880673422316, 209.6470497212048372, 93.84886208192143897 ) ) ;
#18478=CARTESIAN_POINT ( 'NONE',  ( 4.903702542908601636, 200.1653181626581102, 26.45113791807857240 ) ) ;
#18484=CARTESIAN_POINT ( 'NONE',  ( -2.517493886308901807, 199.4062855549015012, 92.90113791807857524 ) ) ;
#18487=CARTESIAN_POINT ( 'NONE',  ( -4.903702542908436435, 200.1653181626580249, 62.04886208192144181 ) ) ;
#18492=CARTESIAN_POINT ( 'NONE',  ( -8.118202686958039038, 201.1607312380087080, 9.201137918078565292 ) ) ;
#18496=CARTESIAN_POINT ( 'NONE',  ( -3.753561863808691168, 195.6020594897209435, 71.90113791807856103 ) ) ;
#18498=CARTESIAN_POINT ( 'NONE',  ( -6.220909254589537696, 198.5229672870051445, 90.05113791807858092 ) ) ;
#18502=CARTESIAN_POINT ( 'NONE',  ( -9.736236675708031640, 214.0148392665760753, 47.79886208192143471 ) ) ;
#18503=CARTESIAN_POINT ( 'NONE',  ( -10.00000000000000711, 206.9523078486584495, 62.49886208192143755 ) ) ;
#18504=CARTESIAN_POINT ( 'NONE',  ( 9.680171189290831535, 199.9079932115568852, 95.30113791807858092 ) ) ;
#18507=CARTESIAN_POINT ( 'NONE',  ( 3.044812012440130555, 197.4746971517856764, 11.60113791807856742 ) ) ;
#18508=CARTESIAN_POINT ( 'NONE',  ( -8.118202686958138514, 212.8392687619910930, 74.79886208192144181 ) ) ;
#18510=CARTESIAN_POINT ( 'NONE',  ( -10.00000000000000711, 207.0476921513413515, 99.50113791807856956 ) ) ;
#18514=CARTESIAN_POINT ( 'NONE',  ( -4.984841277089891776, 213.7757310962905990, 62.94886208192144039 ) ) ;
#18520=UNCERTAINTY_MEASURE_WITH_UNIT (LENGTH_MEASURE( 1.000000000000000082E-05 ), #23960, 'distance_accuracy_value', 'NONE');
#18523=CARTESIAN_POINT ( 'NONE',  ( -4.984841277089726574, 200.2242689037092305, 63.05113791807858092 ) ) ;
#18527=CARTESIAN_POINT ( 'NONE',  ( -4.984841277089891776, 213.7757310962905990, 35.94886208192144039 ) ) ;
#18528=CARTESIAN_POINT ( 'NONE',  ( 3.135527875058820690, 216.4958274776887492, 79.40113791807857524 ) ) ;
#18530=CARTESIAN_POINT ( 'NONE',  ( -10.00000000000000711, 207.0476921513413515, 57.50113791807856956 ) ) ;
#18532=CARTESIAN_POINT ( 'NONE',  ( -9.984503880673473830, 210.2968891136704315, 24.65113791807856103 ) ) ;
#18533=CARTESIAN_POINT ( 'NONE',  ( -0.05014649552807731031, 198.5883022060938572, 14.75113791807856600 ) ) ;
#18537=CARTESIAN_POINT ( 'NONE',  ( -3.662846001190052991, 218.4274158808045740, 40.10113791807856387 ) ) ;
#18539=CARTESIAN_POINT ( 'NONE',  ( -3.135527875058821579, 197.5041725223112223, 80.90113791807858945 ) ) ;
#18540=CARTESIAN_POINT ( 'NONE',  ( -10.01549611932653860, 203.7984951890123000, 60.35113791807857808 ) ) ;
#18541=CARTESIAN_POINT ( 'NONE',  ( 3.753561863808876797, 195.6020594897209719, 19.59886208192143897 ) ) ;
#18542=CARTESIAN_POINT ( 'NONE',  ( 3.135527875058981895, 197.5041725223112792, 28.59886208192143897 ) ) ;
#18544=CARTESIAN_POINT ( 'NONE',  ( 3.753561863808689836, 218.3979405102790565, 64.40113791807856103 ) ) ;
#18545=CARTESIAN_POINT ( 'NONE',  ( 0.05014649552807626948, 215.4116977939061144, 91.25113791807856956 ) ) ;
#18546=CARTESIAN_POINT ( 'NONE',  ( -3.135527875058982783, 216.4958274776886924, 54.09886208192143897 ) ) ;
#18549=CARTESIAN_POINT ( 'NONE',  ( 9.680171189290716072, 214.0920067884432854, 48.69886208192144039 ) ) ;
#18557=CARTESIAN_POINT ( 'NONE',  ( -2.426778023690262742, 214.6231898156240163, 40.10113791807857098 ) ) ;
#18561=CARTESIAN_POINT ( 'NONE',  ( 6.220909254589681581, 198.5229672870052582, 22.44886208192143329 ) ) ;
#18567=CARTESIAN_POINT ( 'NONE',  ( 6.500168698208244500, 202.3363017425938324, 10.29886208192143471 ) ) ;
#18568=CARTESIAN_POINT ( 'NONE',  ( 6.220909254589536808, 215.4770327129947702, 52.55113791807858092 ) ) ;
#18570=CARTESIAN_POINT ( 'NONE',  ( 6.220909254589536808, 215.4770327129947702, 28.55113791807855961 ) ) ;
#18574=CARTESIAN_POINT ( 'NONE',  ( 8.015496119326595448, 204.4483345814782638, 91.14886208192143613 ) ) ;
#18578=CARTESIAN_POINT ( 'NONE',  ( 12.01549611932652972, 210.8513442034534933, 13.85113791807856742 ) ) ;
#18581=CARTESIAN_POINT ( 'NONE',  ( 10.00000000000000711, 206.9523078486586201, 53.00113791807857666 ) ) ;
#18582=CARTESIAN_POINT ( 'NONE',  ( -0.05014649552810635652, 196.4853777576173002, 32.75113791807856956 ) ) ;
#18585=CARTESIAN_POINT ( 'NONE',  ( 10.00000000000000711, 207.0476921513415220, 3.998862081921434442 ) ) ;
#18588=CARTESIAN_POINT ( 'NONE',  ( 9.736236675707914401, 214.0148392665762458, 43.70113791807857240 ) ) ;
#18590=CARTESIAN_POINT ( 'NONE',  ( 10.00000000000000711, 207.0476921513415220, 24.99886208192143400 ) ) ;
#18594=CARTESIAN_POINT ( 'NONE',  ( 0.05014649552810505201, 217.5146222423826714, 73.25113791807855534 ) ) ;
#18600=CARTESIAN_POINT ( 'NONE',  ( 6.500168698208129925, 211.6636982574063381, 13.70113791807856707 ) ) ;
#18602=CARTESIAN_POINT ( 'NONE',  ( -11.98450388067341876, 203.0532714938636047, 101.3488620819214390 ) ) ;
#18607=CARTESIAN_POINT ( 'NONE',  ( -0.05014649552810635652, 196.4853777576173002, 5.751137918078563338 ) ) ;
#18609=CARTESIAN_POINT ( 'NONE',  ( -6.220909254589682469, 215.4770327129946850, 83.94886208192143329 ) ) ;
#18611=CARTESIAN_POINT ( 'NONE',  ( -10.00000000000000711, 207.0476921513413515, 24.50113791807856600 ) ) ;
#18614=CARTESIAN_POINT ( 'NONE',  ( 10.00000000000000711, 206.9523078486586201, 101.0011379180785696 ) ) ;
#18616=CARTESIAN_POINT ( 'NONE',  ( -3.135527875058821579, 197.5041725223112223, 89.90113791807857524 ) ) ;
#18619=CARTESIAN_POINT ( 'NONE',  ( 12.00000000000000711, 207.0476921513415220, 96.99886208192143044 ) ) ;
#18627=CARTESIAN_POINT ( 'NONE',  ( 10.01549611932659367, 203.7984951890124421, 91.14886208192142192 ) ) ;
#18629=CARTESIAN_POINT ( 'NONE',  ( -0.05014649552828442242, 219.6175466908591716, 33.24886208192143755 ) ) ;
#18631=CARTESIAN_POINT ( 'NONE',  ( 6.139770520408368348, 198.4640165459539674, 38.45113791807855819 ) ) ;
#18634=CARTESIAN_POINT ( 'NONE',  ( -6.139770520408224463, 198.4640165459539389, 104.0488620819214276 ) ) ;
#18637=CARTESIAN_POINT ( 'NONE',  ( 2.426778023690075337, 214.6231898156240447, 87.39886208192143613 ) ) ;
#18638=CARTESIAN_POINT ( 'NONE',  ( -6.500168698208129925, 202.3363017425936050, 33.20113791807857240 ) ) ;
#18645=CARTESIAN_POINT ( 'NONE',  ( 8.000000000000008882, 206.9523078486586485, 86.00113791807856956 ) ) ;
#18650=CARTESIAN_POINT ( 'NONE',  ( 8.015496119326595448, 204.4483345814782638, 73.14886208192142192 ) ) ;
#18654=CARTESIAN_POINT ( 'NONE',  ( 3.044812012440130555, 197.4746971517856764, 11.60113791807856742 ) ) ;
#18658=CARTESIAN_POINT ( 'NONE',  ( 12.01549611932652972, 210.8513442034534933, 73.85113791807857808 ) ) ;
#18660=CARTESIAN_POINT ( 'NONE',  ( -10.01549611932653860, 203.7984951890123000, 96.35113791807856387 ) ) ;
#18662=ORIENTED_EDGE ( 'NONE', *, *, #21677, .T. ) ;
#18663=CARTESIAN_POINT ( 'NONE',  ( 7.375838497908012492, 217.2372850707501186, 60.54886208192144181 ) ) ;
#18665=CARTESIAN_POINT ( 'NONE',  ( 6.220909254589680693, 198.5229672870052582, 64.44886208192141908 ) ) ;
#18666=CARTESIAN_POINT ( 'NONE',  ( 9.736236675708031640, 199.9851607334238963, 1.298862081921434264 ) ) ;
#18668=CARTESIAN_POINT ( 'NONE',  ( 10.01549611932653860, 210.2015048109876716, 16.85113791807856032 ) ) ;
#18669=CARTESIAN_POINT ( 'NONE',  ( 3.135527875058981895, 197.5041725223112792, 82.59886208192143897 ) ) ;
#18675=CARTESIAN_POINT ( 'NONE',  ( 8.000000000000008882, 207.0476921513415220, 63.99886208192143044 ) ) ;
#18684=CARTESIAN_POINT ( 'NONE',  ( 8.000000000000008882, 206.9523078486586485, 62.00113791807856956 ) ) ;
#18685=SURFACE_SIDE_STYLE ('',( #31954 ) ) ;
#18687=CARTESIAN_POINT ( 'NONE',  ( -9.638035089578760761, 206.0123451664802587, 104.4144579948609390 ) ) ;
#18691=CARTESIAN_POINT ( 'NONE',  ( -8.000000000000008882, 206.9523078486584780, 44.49886208192143755 ) ) ;
#18692=CARTESIAN_POINT ( 'NONE',  ( -3.044812012440131443, 216.5253028482142952, 85.10113791807857808 ) ) ;
#18694=CARTESIAN_POINT ( 'NONE',  ( 3.135527875058820690, 216.4958274776887492, 67.40113791807857524 ) ) ;
#18697=CARTESIAN_POINT ( 'NONE',  ( -4.903702542908602524, 213.8346818373418898, 15.95113791807856707 ) ) ;
#18702=CARTESIAN_POINT ( 'NONE',  ( -12.00000000000000711, 207.0476921513413515, 48.50113791807856956 ) ) ;
#18705=CARTESIAN_POINT ( 'NONE',  ( -10.01549611932653860, 203.7984951890123284, 99.35113791807857808 ) ) ;
#18706=CARTESIAN_POINT ( 'NONE',  ( 10.00000000000000711, 206.9523078486586201, 62.00113791807856956 ) ) ;
#18708=CARTESIAN_POINT ( 'NONE',  ( 11.98450388067341876, 210.9467285061363953, 18.84886208192143187 ) ) ;
#18709=CARTESIAN_POINT ( 'NONE',  ( -6.139770520408224463, 198.4640165459539105, 38.04886208192143471 ) ) ;
#18712=CARTESIAN_POINT ( 'NONE',  ( 12.01549611932652972, 210.8513442034534933, 76.85113791807856387 ) ) ;
#18713=CARTESIAN_POINT ( 'NONE',  ( -8.015496119326531499, 204.4483345814780364, 93.35113791807857808 ) ) ;
#18715=CARTESIAN_POINT ( 'NONE',  ( -6.220909254589682469, 215.4770327129946850, 50.94886208192141908 ) ) ;
#18718=CARTESIAN_POINT ( 'NONE',  ( 12.01549611932659367, 203.1486557965466773, 52.14886208192143613 ) ) ;
#18725=CARTESIAN_POINT ( 'NONE',  ( 0.05014649552807626948, 215.4116977939061144, 55.25113791807857666 ) ) ;
#18727=CARTESIAN_POINT ( 'NONE',  ( 6.220909254589681581, 198.5229672870052582, 31.44886208192142263 ) ) ;
#18732=CARTESIAN_POINT ( 'NONE',  ( 2.426778023690075337, 214.6231898156240447, 6.398862081921435241 ) ) ;
#18733=CARTESIAN_POINT ( 'NONE',  ( -0.05014649552810635652, 196.4853777576173002, 50.75113791807856956 ) ) ;
#18735=CARTESIAN_POINT ( 'NONE',  ( 6.139770520408368348, 198.4640165459539674, 35.45113791807857240 ) ) ;
#18738=CARTESIAN_POINT ( 'NONE',  ( 2.426778023690075337, 214.6231898156240447, 90.39886208192143613 ) ) ;
#18741=CARTESIAN_POINT ( 'NONE',  ( -9.680171189290831535, 214.0920067884431148, 12.80113791807856849 ) ) ;
#18745=CARTESIAN_POINT ( 'NONE',  ( -6.139770520408369237, 215.5359834540460042, 63.95113791807857950 ) ) ;
#18747=CARTESIAN_POINT ( 'NONE',  ( 0.05014649552810506589, 217.5146222423826714, 28.25113791807856245 ) ) ;
#18750=CARTESIAN_POINT ( 'NONE',  ( 6.139770520408223575, 215.5359834540460611, 9.548862081921432932 ) ) ;
#18754=CARTESIAN_POINT ( 'NONE',  ( -0.05014649552807705357, 194.3824533091408000, 38.75113791807856245 ) ) ;
#18757=CARTESIAN_POINT ( 'NONE',  ( 10.01549611932659545, 203.7984951890123853, 19.14886208192142902 ) ) ;
#18760=CARTESIAN_POINT ( 'NONE',  ( -8.062137200540920645, 212.9164362838581894, 81.80113791807858092 ) ) ;
#18766=CARTESIAN_POINT ( 'NONE',  ( -8.015496119326531499, 204.4483345814780364, 15.35113791807856387 ) ) ;
#18768=CARTESIAN_POINT ( 'NONE',  ( 9.680171189290716072, 214.0920067884432854, 99.69886208192144750 ) ) ;
#18774=CARTESIAN_POINT ( 'NONE',  ( -10.01549611932659722, 210.2015048109875011, 77.64886208192143613 ) ) ;
#18776=CARTESIAN_POINT ( 'NONE',  ( 3.044812012440130555, 197.4746971517856764, 23.60113791807857098 ) ) ;
#18781=CARTESIAN_POINT ( 'NONE',  ( -3.135527875058821579, 197.5041725223112223, 83.90113791807857524 ) ) ;
#18784=CARTESIAN_POINT ( 'NONE',  ( 3.662846001189864698, 218.4274158808046593, 99.39886208192146455 ) ) ;
#18793=CARTESIAN_POINT ( 'NONE',  ( -10.01549611932659545, 210.2015048109875011, 92.64886208192143613 ) ) ;
#18794=CARTESIAN_POINT ( 'NONE',  ( -9.680171189290716072, 199.9079932115567146, 29.19886208192143684 ) ) ;
#18796=CARTESIAN_POINT ( 'NONE',  ( 8.062137200540920645, 201.0835637161417822, 50.30113791807857382 ) ) ;
#18798=CARTESIAN_POINT ( 'NONE',  ( 4.984841277089891776, 200.2242689037093726, 7.448862081921436840 ) ) ;
#18801=CARTESIAN_POINT ( 'NONE',  ( -2.426778023690076225, 199.3768101843759553, 85.89886208192143613 ) ) ;
#18802=CARTESIAN_POINT ( 'NONE',  ( 6.444103211791042618, 202.2591342207267644, 29.30113791807857027 ) ) ;
#18808=CARTESIAN_POINT ( 'NONE',  ( 2.517493886308900919, 214.5937144450984420, 100.4011379180785895 ) ) ;
#18811=CARTESIAN_POINT ( 'NONE',  ( 4.903702542908435547, 213.8346818373419751, 69.54886208192141339 ) ) ;
#18812=FACE_OUTER_BOUND ( 'NONE', #1194, .T. ) ;
#18814=CARTESIAN_POINT ( 'NONE',  ( -10.01549611932653860, 203.7984951890123000, 12.35113791807856387 ) ) ;
#18819=CARTESIAN_POINT ( 'NONE',  ( 7.456977232089302632, 217.1783343296989131, 76.55113791807858092 ) ) ;
#18821=CARTESIAN_POINT ( 'NONE',  ( 9.984503880673473830, 203.7031108863295401, 98.15113791807858945 ) ) ;
#18825=CARTESIAN_POINT ( 'NONE',  ( 12.00000000000000711, 207.0476921513415220, 63.99886208192143044 ) ) ;
#18826=CARTESIAN_POINT ( 'NONE',  ( 3.044812012439969795, 216.5253028482143520, 66.39886208192143613 ) ) ;
#18827=CARTESIAN_POINT ( 'NONE',  ( -11.89830997168683702, 232.6342992855866783, 103.4854814124441447 ) ) ;
#18829=CARTESIAN_POINT ( 'NONE',  ( 10.01549611932653860, 210.2015048109876716, 22.85113791807856742 ) ) ;
#18830=CARTESIAN_POINT ( 'NONE',  ( -6.139770520408224463, 198.4640165459539389, 83.04886208192144181 ) ) ;
#18836=CARTESIAN_POINT ( 'NONE',  ( -0.05014649552828365914, 215.4116977939061144, 57.24886208192145887 ) ) ;
#18844=CARTESIAN_POINT ( 'NONE',  ( 0.05014649552807626948, 215.4116977939061144, 73.25113791807858377 ) ) ;
#18848=CARTESIAN_POINT ( 'NONE',  ( 8.000000000000008882, 207.0476921513415220, 48.99886208192144466 ) ) ;
#18849=CARTESIAN_POINT ( 'NONE',  ( 3.044812012440130555, 197.4746971517856764, 77.60113791807857808 ) ) ;
#18850=CARTESIAN_POINT ( 'NONE',  ( -10.00000000000000711, 207.0476921513413515, 69.50113791807856956 ) ) ;
#18852=FACE_OUTER_BOUND ( 'NONE', #15464, .T. ) ;
#18853=CARTESIAN_POINT ( 'NONE',  ( -8.015496119326531499, 204.4483345814780364, 21.35113791807856742 ) ) ;
#18857=CARTESIAN_POINT ( 'NONE',  ( 3.753561863808689836, 218.3979405102790565, 49.40113791807856813 ) ) ;
#18859=CARTESIAN_POINT ( 'NONE',  ( -0.05014649552810635652, 196.4853777576173002, 92.75113791807858377 ) ) ;
#18860=CARTESIAN_POINT ( 'NONE',  ( -3.044812012440131443, 216.5253028482142952, 70.10113791807857808 ) ) ;
#18861=CARTESIAN_POINT ( 'NONE',  ( 7.456977232089471386, 196.8216656703012006, 31.44886208192143684 ) ) ;
#18862=CARTESIAN_POINT ( 'NONE',  ( -3.044812012439970683, 197.4746971517856196, 34.89886208192143613 ) ) ;
#18864=CARTESIAN_POINT ( 'NONE',  ( 9.680171189290831535, 199.9079932115568852, 74.30113791807858092 ) ) ;
#18865=CARTESIAN_POINT ( 'NONE',  ( -8.000000000000008882, 207.0476921513413515, 90.50113791807858377 ) ) ;
#18866=CARTESIAN_POINT ( 'NONE',  ( 10.00000000000000711, 207.0476921513415220, 45.99886208192143755 ) ) ;
#18871=CARTESIAN_POINT ( 'NONE',  ( 3.662846001189864698, 218.4274158808046593, 66.39886208192143613 ) ) ;
#18874=CARTESIAN_POINT ( 'NONE',  ( 4.984841277089891776, 200.2242689037093726, 34.44886208192144039 ) ) ;
#18882=CARTESIAN_POINT ( 'NONE',  ( 6.500168698208129925, 211.6636982574063381, 52.70113791807857240 ) ) ;
#18884=CARTESIAN_POINT ( 'NONE',  ( -6.139770520408224463, 198.4640165459539389, 35.04886208192144181 ) ) ;
#18888=CARTESIAN_POINT ( 'NONE',  ( -6.444103211790928043, 202.2591342207265939, 20.19886208192143684 ) ) ;
#18890=CARTESIAN_POINT ( 'NONE',  ( -10.00000000000000711, 207.0476921513413515, 51.50113791807857666 ) ) ;
#18892=CARTESIAN_POINT ( 'NONE',  ( 10.01549611932653860, 210.2015048109876716, 34.85113791807856387 ) ) ;
#18896=CARTESIAN_POINT ( 'NONE',  ( 6.444103211790928043, 211.7408657792734061, 93.69886208192144750 ) ) ;
#18900=CARTESIAN_POINT ( 'NONE',  ( -12.00000000000000711, 207.0476921513413515, 15.50113791807856600 ) ) ;
#18904=CARTESIAN_POINT ( 'NONE',  ( 6.139770520408368348, 198.4640165459539674, 68.45113791807858661 ) ) ;
#18905=CARTESIAN_POINT ( 'NONE',  ( 10.01549611932653860, 210.2015048109876716, 37.85113791807856387 ) ) ;
#18909=CARTESIAN_POINT ( 'NONE',  ( 6.139770520408223575, 215.5359834540460611, 6.548862081921434708 ) ) ;
#18912=CARTESIAN_POINT ( 'NONE',  ( 11.98450388067348271, 203.0532714938637753, 44.15113791807856813 ) ) ;
#18914=CARTESIAN_POINT ( 'NONE',  ( -10.00000000000000711, 206.9523078486584495, 23.49886208192143755 ) ) ;
#18917=CARTESIAN_POINT ( 'NONE',  ( -3.135527875058821579, 197.5041725223112223, 77.90113791807857524 ) ) ;
#18925=CARTESIAN_POINT ( 'NONE',  ( -8.000000000000008882, 207.0476921513413515, 24.50113791807856600 ) ) ;
#18928=CARTESIAN_POINT ( 'NONE',  ( -10.00000000000000711, 206.9523078486584495, 2.498862081921433997 ) ) ;
#18936=CARTESIAN_POINT ( 'NONE',  ( 6.139770520408223575, 215.5359834540460611, 90.54886208192144181 ) ) ;
#18938=CARTESIAN_POINT ( 'NONE',  ( -10.01549611932653860, 203.7984951890123284, 21.35113791807855677 ) ) ;
#18941=CARTESIAN_POINT ( 'NONE',  ( 12.01549611932659367, 203.1486557965466773, 82.14886208192143613 ) ) ;
#18945=CARTESIAN_POINT ( 'NONE',  ( 10.00000000000000711, 206.9523078486586201, 98.00113791807856956 ) ) ;
#18950=CARTESIAN_POINT ( 'NONE',  ( 3.135527875058820690, 216.4958274776887492, 40.40113791807857524 ) ) ;
#18956=CARTESIAN_POINT ( 'NONE',  ( 3.753561863808689836, 218.3979405102790565, 22.40113791807856813 ) ) ;
#18961=CARTESIAN_POINT ( 'NONE',  ( -10.00000000000000711, 206.9523078486584495, 98.49886208192143044 ) ) ;
#18962=CARTESIAN_POINT ( 'NONE',  ( 7.456977232089471386, 196.8216656703012006, 37.44886208192143329 ) ) ;
#18963=CARTESIAN_POINT ( 'NONE',  ( -9.996365641501871124, 207.8097375604742467, 102.5363179372327096 ) ) ;
#18964=CARTESIAN_POINT ( 'NONE',  ( -9.984503880673473830, 210.2968891136704315, 48.65113791807858235 ) ) ;
#18966=CARTESIAN_POINT ( 'NONE',  ( 0.05014649552828262524, 198.5883022060938572, 13.74886208192143577 ) ) ;
#18969=CARTESIAN_POINT ( 'NONE',  ( 4.903702542908435547, 213.8346818373419751, 99.54886208192144181 ) ) ;
#18973=CARTESIAN_POINT ( 'NONE',  ( 2.517493886308900919, 214.5937144450984420, 37.40113791807856813 ) ) ;
#18978=CARTESIAN_POINT ( 'NONE',  ( -6.139770520408224463, 198.4640165459539389, 56.04886208192142050 ) ) ;
#18982=CARTESIAN_POINT ( 'NONE',  ( 8.015496119326531499, 209.5516654185219636, 100.8511379180785781 ) ) ;
#18987=CARTESIAN_POINT ( 'NONE',  ( 2.426778023690075337, 214.6231898156240447, 72.39886208192143613 ) ) ;
#18990=CARTESIAN_POINT ( 'NONE',  ( -10.01549611932653860, 203.7984951890123000, 6.351137918078565647 ) ) ;
#18994=CARTESIAN_POINT ( 'NONE',  ( -7.375838497908182134, 217.2372850707499765, 72.95113791807857240 ) ) ;
#18996=CARTESIAN_POINT ( 'NONE',  ( 8.062137200540920645, 201.0835637161417822, 95.30113791807858092 ) ) ;
#18999=CARTESIAN_POINT ( 'NONE',  ( 3.662846001189864698, 218.4274158808046593, 102.3988620819214361 ) ) ;
#19000=CARTESIAN_POINT ( 'NONE',  ( -12.01549611932659722, 210.8513442034533227, 59.64886208192143613 ) ) ;
#19001=CARTESIAN_POINT ( 'NONE',  ( 3.135527875058981895, 197.5041725223112792, 64.59886208192143897 ) ) ;
#19002=CARTESIAN_POINT ( 'NONE',  ( 7.375838497908012492, 217.2372850707501186, 3.548862081921434264 ) ) ;
#19004=CARTESIAN_POINT ( 'NONE',  ( 10.00000000000000711, 206.9523078486586201, 20.00113791807856600 ) ) ;
#19005=CARTESIAN_POINT ( 'NONE',  ( -0.05014649552828403384, 217.5146222423826714, 90.24886208192141623 ) ) ;
#19007=DIRECTION ( 'NONE',  ( -0.9891821073486152249, -0.1466927349985428231, 0.000000000000000000 ) ) ;
#19011=CARTESIAN_POINT ( 'NONE',  ( -6.444103211790928043, 202.2591342207265939, 62.19886208192144750 ) ) ;
#19018=CARTESIAN_POINT ( 'NONE',  ( 7.984503880673485376, 204.3529502787953902, 68.15113791807856103 ) ) ;
#19022=CARTESIAN_POINT ( 'NONE',  ( -6.444103211790928043, 202.2591342207265939, 44.19886208192144750 ) ) ;
#19023=CARTESIAN_POINT ( 'NONE',  ( -6.220909254589537696, 198.5229672870051161, 81.05113791807856671 ) ) ;
#19024=CARTESIAN_POINT ( 'NONE',  ( -9.984503880673473830, 210.2968891136704315, 69.65113791807854682 ) ) ;
#19025=CARTESIAN_POINT ( 'NONE',  ( -10.00000000000000178, 205.7704093527941893, 108.2846756197957490 ) ) ;
#19026=CARTESIAN_POINT ( 'NONE',  ( 4.903702542908601636, 200.1653181626581102, 20.45113791807856529 ) ) ;
#19030=CARTESIAN_POINT ( 'NONE',  ( 3.662846001190051659, 195.5725841191953691, 47.60113791807857808 ) ) ;
#19031=CARTESIAN_POINT ( 'NONE',  ( -1.472725187932624030E-14, 206.9977241638431167, -6.000000000000014211 ) ) ;
#19032=CARTESIAN_POINT ( 'NONE',  ( -3.044812012440131443, 216.5253028482142952, 97.10113791807857808 ) ) ;
#19033=CARTESIAN_POINT ( 'NONE',  ( 3.044812012440130555, 197.4746971517856764, 71.60113791807857808 ) ) ;
#19034=CARTESIAN_POINT ( 'NONE',  ( 3.753561863808876797, 195.6020594897209719, 34.59886208192143187 ) ) ;
#19035=CARTESIAN_POINT ( 'NONE',  ( -6.220909254589682469, 215.4770327129947134, 35.94886208192142618 ) ) ;
#19037=CARTESIAN_POINT ( 'NONE',  ( -7.456977232089304408, 196.8216656703010301, 78.05113791807858092 ) ) ;
#19038=CARTESIAN_POINT ( 'NONE',  ( 8.015496119326531499, 209.5516654185219636, 94.85113791807856387 ) ) ;
#19039=CARTESIAN_POINT ( 'NONE',  ( 3.135527875058981895, 197.5041725223112792, 46.59886208192143187 ) ) ;
#19042=CARTESIAN_POINT ( 'NONE',  ( -7.375838497908014268, 196.7627149292498530, 59.04886208192144181 ) ) ;
#19044=CARTESIAN_POINT ( 'NONE',  ( -4.903702542908436435, 200.1653181626580249, 32.04886208192144181 ) ) ;
#19050=CARTESIAN_POINT ( 'NONE',  ( -4.903702542908602524, 213.8346818373418898, 48.95113791807857240 ) ) ;
#19052=CARTESIAN_POINT ( 'NONE',  ( -6.139770520408224463, 198.4640165459539389, 32.04886208192143471 ) ) ;
#19054=ORIENTED_EDGE ( 'NONE', *, *, #20368, .F. ) ;
#19058=CARTESIAN_POINT ( 'NONE',  ( -6.444103211790928043, 202.2591342207265939, 17.19886208192143684 ) ) ;
#19059=CARTESIAN_POINT ( 'NONE',  ( -10.00000000000000711, 207.0476921513413515, 54.50113791807857666 ) ) ;
#19063=CARTESIAN_POINT ( 'NONE',  ( 9.984503880673470277, 203.7031108863295401, 41.15113791807855392 ) ) ;
#19065=CARTESIAN_POINT ( 'NONE',  ( -6.444103211790928043, 202.2591342207265939, 104.1988620819214475 ) ) ;
#19069=CARTESIAN_POINT ( 'NONE',  ( -12.00000000000000711, 207.0476921513413515, 21.50113791807856956 ) ) ;
#19072=CARTESIAN_POINT ( 'NONE',  ( 8.062137200540920645, 201.0835637161417822, 65.30113791807858092 ) ) ;
#19073=CARTESIAN_POINT ( 'NONE',  ( 6.139770520408367460, 198.4640165459539389, 35.45113791807857240 ) ) ;
#19076=CARTESIAN_POINT ( 'NONE',  ( 12.01549611932659367, 203.1486557965466773, 4.148862081921434353 ) ) ;
#19077=CARTESIAN_POINT ( 'NONE',  ( 3.044812012439969795, 216.5253028482143520, 6.398862081921435241 ) ) ;
#19081=CARTESIAN_POINT ( 'NONE',  ( 12.01549611932652972, 210.8513442034534933, 43.85113791807856387 ) ) ;
#19082=CARTESIAN_POINT ( 'NONE',  ( 8.000000000000008882, 206.9523078486586485, 74.00113791807856956 ) ) ;
#19084=CARTESIAN_POINT ( 'NONE',  ( 8.062137200540822946, 212.9164362838583315, 24.69886208192143684 ) ) ;
#19087=CARTESIAN_POINT ( 'NONE',  ( -3.044812012440131443, 216.5253028482142952, 85.10113791807857808 ) ) ;
#19092=CARTESIAN_POINT ( 'NONE',  ( -8.000000000000008882, 207.0476921513413515, 18.50113791807856956 ) ) ;
#19095=CARTESIAN_POINT ( 'NONE',  ( 8.062137200540822946, 212.9164362838583315, 6.698862081921435063 ) ) ;
#19103=CARTESIAN_POINT ( 'NONE',  ( -3.044812012439970683, 197.4746971517856196, 88.89886208192143613 ) ) ;
#19105=CARTESIAN_POINT ( 'NONE',  ( -6.220909254589537696, 198.5229672870051161, 27.05113791807856671 ) ) ;
#19108=CARTESIAN_POINT ( 'NONE',  ( 7.375838497908012492, 217.2372850707501186, 81.54886208192144181 ) ) ;
#19111=CARTESIAN_POINT ( 'NONE',  ( -8.118202686958039038, 201.1607312380087080, 96.20113791807857240 ) ) ;
#19114=CARTESIAN_POINT ( 'NONE',  ( -8.118202686958039038, 201.1607312380087080, 36.20113791807857240 ) ) ;
#19120=CARTESIAN_POINT ( 'NONE',  ( -7.456977232089304408, 196.8216656703010301, 21.05113791807857027 ) ) ;
#19125=CARTESIAN_POINT ( 'NONE',  ( 9.736236675708031640, 199.9851607334238963, 31.29886208192143826 ) ) ;
#19127=CARTESIAN_POINT ( 'NONE',  ( 10.01549611932653860, 210.2015048109876716, 52.85113791807854966 ) ) ;
#19130=CARTESIAN_POINT ( 'NONE',  ( -6.500168698208244500, 211.6636982574061676, 11.79886208192143648 ) ) ;
#19133=CARTESIAN_POINT ( 'NONE',  ( 6.444103211790928043, 211.7408657792734061, 99.69886208192144750 ) ) ;
#19134=CARTESIAN_POINT ( 'NONE',  ( -8.015496119326531499, 204.4483345814780364, 36.35113791807857098 ) ) ;
#19138=CARTESIAN_POINT ( 'NONE',  ( 8.062137200540822946, 212.9164362838583315, 60.69886208192143329 ) ) ;
#19141=CARTESIAN_POINT ( 'NONE',  ( 6.444103211791042618, 202.2591342207267644, 98.30113791807858092 ) ) ;
#19143=CARTESIAN_POINT ( 'NONE',  ( -0.05014649552828365914, 215.4116977939061144, 72.24886208192143044 ) ) ;
#19147=CARTESIAN_POINT ( 'NONE',  ( 3.044812012440130555, 197.4746971517856764, 14.60113791807856565 ) ) ;
#19152=CARTESIAN_POINT ( 'NONE',  ( 9.680171189290831535, 199.9079932115568852, 77.30113791807858092 ) ) ;
#19155=CARTESIAN_POINT ( 'NONE',  ( -8.062137200540920645, 212.9164362838581894, 99.80113791807858092 ) ) ;
#19158=CARTESIAN_POINT ( 'NONE',  ( 10.00000000000000711, 207.0476921513415220, 3.998862081921434442 ) ) ;
#19159=CARTESIAN_POINT ( 'NONE',  ( -3.753561863808878130, 218.3979405102790281, 66.09886208192142476 ) ) ;
#19160=CARTESIAN_POINT ( 'NONE',  ( 6.139770520408223575, 215.5359834540460611, 63.54886208192144181 ) ) ;
#19161=CARTESIAN_POINT ( 'NONE',  ( -12.00000000000000711, 207.0476921513413515, 102.5011379180785696 ) ) ;
#19163=CARTESIAN_POINT ( 'NONE',  ( 8.118202686958039038, 212.8392687619912635, 19.70113791807856884 ) ) ;
#19166=CARTESIAN_POINT ( 'NONE',  ( 3.135527875058981895, 197.5041725223112792, 91.59886208192143897 ) ) ;
#19172=CARTESIAN_POINT ( 'NONE',  ( -6.500168698208244500, 211.6636982574061676, 68.79886208192144181 ) ) ;
#19181=CARTESIAN_POINT ( 'NONE',  ( 7.984503880673485376, 204.3529502787953902, 71.15113791807857524 ) ) ;
#19182=DIRECTION ( 'NONE',  ( 0.000000000000000000, 0.9988620819214349966, -0.04769215134146094492 ) ) ;
#19186=CARTESIAN_POINT ( 'NONE',  ( -8.000000000000008882, 206.9523078486584780, 41.49886208192143755 ) ) ;
#19187=CARTESIAN_POINT ( 'NONE',  ( -3.135527875058821579, 197.5041725223112223, 89.90113791807857524 ) ) ;
#19188=CARTESIAN_POINT ( 'NONE',  ( 0.05014649552810505201, 217.5146222423826714, 64.25113791807856956 ) ) ;
#19191=CARTESIAN_POINT ( 'NONE',  ( 8.015496119326531499, 209.5516654185219636, 25.85113791807856742 ) ) ;
#19195=CARTESIAN_POINT ( 'NONE',  ( 9.736236675707914401, 214.0148392665762458, 49.70113791807856529 ) ) ;
#19197=CARTESIAN_POINT ( 'NONE',  ( 8.062137200540920645, 201.0835637161417822, 98.30113791807858092 ) ) ;
#19198=CARTESIAN_POINT ( 'NONE',  ( -9.984503880673475606, 210.2968891136704315, 72.65113791807857524 ) ) ;
#19199=CARTESIAN_POINT ( 'NONE',  ( -3.753561863808878130, 218.3979405102790281, 36.09886208192143187 ) ) ;
#19200=CARTESIAN_POINT ( 'NONE',  ( 3.135527875058981895, 197.5041725223112792, 40.59886208192143187 ) ) ;
#19203=CARTESIAN_POINT ( 'NONE',  ( 7.375838497908181246, 196.7627149292499666, 74.45113791807855819 ) ) ;
#19204=CARTESIAN_POINT ( 'NONE',  ( 2.517493886308900919, 214.5937144450984420, 100.4011379180785895 ) ) ;
#19206=CARTESIAN_POINT ( 'NONE',  ( 10.00000000000000711, 207.0476921513415220, 63.99886208192143044 ) ) ;
#19209=CARTESIAN_POINT ( 'NONE',  ( -3.662846001189865142, 195.5725841191952838, 61.89886208192143613 ) ) ;
#19212=CARTESIAN_POINT ( 'NONE',  ( 8.015496119326595448, 204.4483345814782638, 43.14886208192144323 ) ) ;
#19218=CARTESIAN_POINT ( 'NONE',  ( 2.426778023690261410, 199.3768101843759837, 47.60113791807857808 ) ) ;
#19221=CARTESIAN_POINT ( 'NONE',  ( -0.05014649552828403384, 217.5146222423826714, 36.24886208192143755 ) ) ;
#19228=CARTESIAN_POINT ( 'NONE',  ( -2.426778023690076225, 199.3768101843759553, 10.89886208192143613 ) ) ;
#19230=CARTESIAN_POINT ( 'NONE',  ( 0.05014649552810505201, 217.5146222423826714, 55.25113791807858377 ) ) ;
#19231=CARTESIAN_POINT ( 'NONE',  ( -3.135527875058821579, 197.5041725223112223, 38.90113791807857524 ) ) ;
#19235=CARTESIAN_POINT ( 'NONE',  ( 8.015496119326595448, 204.4483345814782638, 100.1488620819214646 ) ) ;
#19239=CARTESIAN_POINT ( 'NONE',  ( -3.753561863808691168, 195.6020594897209435, 20.90113791807856813 ) ) ;
#19241=CARTESIAN_POINT ( 'NONE',  ( -10.01549611932653860, 203.7984951890123284, 69.35113791807857808 ) ) ;
#19242=CARTESIAN_POINT ( 'NONE',  ( 0.05014649552810506589, 217.5146222423826714, 43.25113791807858377 ) ) ;
#19245=CARTESIAN_POINT ( 'NONE',  ( -12.01549611932659722, 210.8513442034533227, 2.648862081921433909 ) ) ;
#19246=CARTESIAN_POINT ( 'NONE',  ( -3.044812012439970683, 197.4746971517856196, 7.898862081921434353 ) ) ;
#19249=CARTESIAN_POINT ( 'NONE',  ( 9.680171189290831535, 199.9079932115568852, 50.30113791807857382 ) ) ;
#19250=CARTESIAN_POINT ( 'NONE',  ( 4.903702542908601636, 200.1653181626581102, 68.45113791807857240 ) ) ;
#19252=CARTESIAN_POINT ( 'NONE',  ( 3.044812012439969795, 216.5253028482143520, 30.39886208192143613 ) ) ;
#19255=CARTESIAN_POINT ( 'NONE',  ( 10.00000000000000711, 206.9523078486586201, 80.00113791807856956 ) ) ;
#19262=CARTESIAN_POINT ( 'NONE',  ( -4.903702542908602524, 213.8346818373418898, 24.95113791807856884 ) ) ;
#19264=CARTESIAN_POINT ( 'NONE',  ( 8.062137200540822946, 212.9164362838583315, 3.698862081921434619 ) ) ;
#19271=CARTESIAN_POINT ( 'NONE',  ( -3.044812012439970683, 197.4746971517856196, 91.89886208192143613 ) ) ;
#19273=CARTESIAN_POINT ( 'NONE',  ( -10.00000000000000711, 207.0476921513413515, 18.50113791807856956 ) ) ;
#19275=CARTESIAN_POINT ( 'NONE',  ( -7.456977232089471386, 217.1783343296987709, 80.94886208192143329 ) ) ;
#19280=CARTESIAN_POINT ( 'NONE',  ( 10.01549611932653860, 210.2015048109876716, 94.85113791807857808 ) ) ;
#19283=CARTESIAN_POINT ( 'NONE',  ( 8.118202686958039038, 212.8392687619912635, 34.70113791807857240 ) ) ;
#19288=CARTESIAN_POINT ( 'NONE',  ( -11.98450388067348804, 210.9467285061362247, 15.65113791807856636 ) ) ;
#19293=CARTESIAN_POINT ( 'NONE',  ( 3.662846001189864698, 218.4274158808046593, 45.39886208192143613 ) ) ;
#19295=CARTESIAN_POINT ( 'NONE',  ( -10.01549611932653860, 203.7984951890123284, 48.35113791807855677 ) ) ;
#19297=CARTESIAN_POINT ( 'NONE',  ( -7.984503880673422316, 204.3529502787951628, 17.34886208192143187 ) ) ;
#19302=CARTESIAN_POINT ( 'NONE',  ( 2.426778023690075337, 214.6231898156240447, 102.3988620819214361 ) ) ;
#19304=CARTESIAN_POINT ( 'NONE',  ( -2.517493886308901807, 199.4062855549015012, 41.90113791807856813 ) ) ;
#19309=CARTESIAN_POINT ( 'NONE',  ( 8.062137200540822946, 212.9164362838583315, 63.69886208192143329 ) ) ;
#19312=CARTESIAN_POINT ( 'NONE',  ( -7.984503880673488041, 209.6470497212046098, 93.65113791807857524 ) ) ;
#19315=CARTESIAN_POINT ( 'NONE',  ( 2.517493886309087436, 199.4062855549015865, 76.59886208192142476 ) ) ;
#19320=CARTESIAN_POINT ( 'NONE',  ( 10.00000000000000711, 206.9523078486586201, 23.00113791807856600 ) ) ;
#19324=CARTESIAN_POINT ( 'NONE',  ( 11.98450388067348271, 203.0532714938637753, 74.15113791807857524 ) ) ;
#19326=CARTESIAN_POINT ( 'NONE',  ( -3.044812012440131443, 216.5253028482142952, 94.10113791807857808 ) ) ;
#19329=CARTESIAN_POINT ( 'NONE',  ( 12.00000000000000711, 207.0476921513415220, 102.9988620819214304 ) ) ;
#19330=CARTESIAN_POINT ( 'NONE',  ( -11.98450388067341876, 203.0532714938636047, 59.34886208192144608 ) ) ;
#19331=CARTESIAN_POINT ( 'NONE',  ( 9.984503880673420539, 210.2968891136705736, 72.84886208192143897 ) ) ;
#19332=CARTESIAN_POINT ( 'NONE',  ( 12.01549611932659367, 203.1486557965466773, 7.148862081921435241 ) ) ;
#19334=CARTESIAN_POINT ( 'NONE',  ( 0.05014649552810505201, 217.5146222423826714, 22.25113791807856956 ) ) ;
#19335=CARTESIAN_POINT ( 'NONE',  ( -10.01549611932659722, 210.2015048109875011, 89.64886208192143613 ) ) ;
#19338=CARTESIAN_POINT ( 'NONE',  ( -1.472725187932624030E-14, 206.9977241638431167, -6.000000000000014211 ) ) ;
#19339=CARTESIAN_POINT ( 'NONE',  ( -8.015496119326597224, 209.5516654185217362, 74.64886208192143613 ) ) ;
#19347=CARTESIAN_POINT ( 'NONE',  ( -8.015496119326531499, 204.4483345814780364, 72.35113791807857808 ) ) ;
#19352=CARTESIAN_POINT ( 'NONE',  ( 2.517493886309087436, 199.4062855549015865, 40.59886208192143897 ) ) ;
#19353=CARTESIAN_POINT ( 'NONE',  ( -9.984503880673473830, 210.2968891136704315, 87.65113791807854682 ) ) ;
#19355=CARTESIAN_POINT ( 'NONE',  ( 6.220909254589536808, 215.4770327129947702, 70.55113791807856671 ) ) ;
#19360=CARTESIAN_POINT ( 'NONE',  ( -3.753561863808691168, 195.6020594897209435, 47.90113791807857524 ) ) ;
#19363=CARTESIAN_POINT ( 'NONE',  ( 10.00000000000000711, 206.9523078486586201, 98.00113791807856956 ) ) ;
#19364=CARTESIAN_POINT ( 'NONE',  ( 10.00000000000000711, 206.9523078486586201, 68.00113791807856956 ) ) ;
#19365=CARTESIAN_POINT ( 'NONE',  ( 3.753561863808876797, 195.6020594897209719, 28.59886208192143897 ) ) ;
#19366=CARTESIAN_POINT ( 'NONE',  ( 3.044812012439969795, 216.5253028482143520, 42.39886208192143613 ) ) ;
#19368=CARTESIAN_POINT ( 'NONE',  ( -12.00000000000000711, 207.0476921513413515, 78.50113791807856956 ) ) ;
#19369=CARTESIAN_POINT ( 'NONE',  ( -8.015496119326531499, 204.4483345814780364, 96.35113791807857808 ) ) ;
#19370=CARTESIAN_POINT ( 'NONE',  ( -0.05014649552828403384, 217.5146222423826714, 60.24886208192142334 ) ) ;
#19373=CARTESIAN_POINT ( 'NONE',  ( 0.05014649552828288198, 194.3824533091408000, 64.74886208192143044 ) ) ;
#19376=CARTESIAN_POINT ( 'NONE',  ( 7.984503880673422316, 209.6470497212048372, 39.84886208192144608 ) ) ;
#19382=CARTESIAN_POINT ( 'NONE',  ( -7.984503880673488041, 209.6470497212046098, 51.65113791807857524 ) ) ;
#19385=CARTESIAN_POINT ( 'NONE',  ( -9.984503880673420539, 203.7031108863293980, 35.34886208192142476 ) ) ;
#19392=CARTESIAN_POINT ( 'NONE',  ( -8.000000000000008882, 206.9523078486584780, 14.49886208192143577 ) ) ;
#19393=CARTESIAN_POINT ( 'NONE',  ( -8.118202686958039038, 201.1607312380087080, 60.20113791807857240 ) ) ;
#19394=CARTESIAN_POINT ( 'NONE',  ( 6.139770520408368348, 198.4640165459539674, 38.45113791807855819 ) ) ;
#19397=CARTESIAN_POINT ( 'NONE',  ( -4.984841277089726574, 200.2242689037092305, 0.05113791807856601229 ) ) ;
#19401=CARTESIAN_POINT ( 'NONE',  ( -11.98450388067348804, 210.9467285061362247, 18.65113791807856458 ) ) ;
#19403=CARTESIAN_POINT ( 'NONE',  ( -8.062137200540920645, 212.9164362838581894, 69.80113791807856671 ) ) ;
#19404=CARTESIAN_POINT ( 'NONE',  ( 6.139770520408367460, 198.4640165459539389, 44.45113791807856529 ) ) ;
#19408=CARTESIAN_POINT ( 'NONE',  ( 11.98450388067341876, 210.9467285061363953, 6.848862081921435419 ) ) ;
#19409=CARTESIAN_POINT ( 'NONE',  ( 3.135527875058981895, 197.5041725223112792, 7.598862081921435419 ) ) ;
#19412=CARTESIAN_POINT ( 'NONE',  ( -12.01549611932652972, 203.1486557965464499, 48.35113791807857098 ) ) ;
#19413=CARTESIAN_POINT ( 'NONE',  ( 4.903702542908601636, 200.1653181626581102, 65.45113791807858661 ) ) ;
#19414=CARTESIAN_POINT ( 'NONE',  ( 6.220909254589681581, 198.5229672870052582, 31.44886208192142263 ) ) ;
#19418=CARTESIAN_POINT ( 'NONE',  ( 0.05014649552810505201, 217.5146222423826714, 94.25113791807855534 ) ) ;
#19423=CARTESIAN_POINT ( 'NONE',  ( -8.015496119326531499, 204.4483345814780364, 18.35113791807856387 ) ) ;
#19427=CARTESIAN_POINT ( 'NONE',  ( 6.139770520408223575, 215.5359834540460611, 6.548862081921434708 ) ) ;
#19431=CARTESIAN_POINT ( 'NONE',  ( -2.426778023690262742, 214.6231898156240163, 49.10113791807857808 ) ) ;
#19434=CARTESIAN_POINT ( 'NONE',  ( 0.05014649552828275708, 196.4853777576173002, 88.74886208192140202 ) ) ;
#19436=CARTESIAN_POINT ( 'NONE',  ( -3.044812012440131443, 216.5253028482142952, 37.10113791807857098 ) ) ;
#19438=CARTESIAN_POINT ( 'NONE',  ( 7.375838497908012492, 217.2372850707501186, 75.54886208192142760 ) ) ;
#19443=CARTESIAN_POINT ( 'NONE',  ( 9.984503880673470277, 203.7031108863295401, 92.15113791807856103 ) ) ;
#19446=CARTESIAN_POINT ( 'NONE',  ( -10.00000000000000711, 207.0476921513413515, 33.50113791807856956 ) ) ;
#19454=CARTESIAN_POINT ( 'NONE',  ( 7.375838497908181246, 196.7627149292499666, 23.45113791807856884 ) ) ;
#19461=CARTESIAN_POINT ( 'NONE',  ( 12.00000000000000711, 207.0476921513415220, 39.99886208192143755 ) ) ;
#19463=CARTESIAN_POINT ( 'NONE',  ( -0.05014649552810635652, 196.4853777576173002, 50.75113791807856956 ) ) ;
#19464=CARTESIAN_POINT ( 'NONE',  ( -0.05014649552828365914, 215.4116977939061144, 9.248862081921435774 ) ) ;
#19468=CARTESIAN_POINT ( 'NONE',  ( 4.903702542908435547, 213.8346818373419751, 102.5488620819214560 ) ) ;
#19470=CARTESIAN_POINT ( 'NONE',  ( -4.984841277089726574, 200.2242689037092305, 45.05113791807857382 ) ) ;
#19474=CARTESIAN_POINT ( 'NONE',  ( -10.00000000000000178, 206.7692714347156198, 108.3323677711372000 ) ) ;
#19477=CARTESIAN_POINT ( 'NONE',  ( -3.044812012439970683, 197.4746971517856196, 64.89886208192145034 ) ) ;
#19480=CARTESIAN_POINT ( 'NONE',  ( -0.05014649552807731031, 198.5883022060938572, 95.75113791807856956 ) ) ;
#19485=CARTESIAN_POINT ( 'NONE',  ( -6.500168698208244500, 211.6636982574061676, 83.79886208192144181 ) ) ;
#19490=CARTESIAN_POINT ( 'NONE',  ( 3.044812012440130555, 197.4746971517856764, 23.60113791807857098 ) ) ;
#19494=CARTESIAN_POINT ( 'NONE',  ( 12.00000000000000711, 206.9523078486586485, 89.00113791807858377 ) ) ;
#19500=CARTESIAN_POINT ( 'NONE',  ( -9.736236675708031640, 214.0148392665760753, 68.79886208192144181 ) ) ;
#19501=CARTESIAN_POINT ( 'NONE',  ( -3.135527875058982783, 216.4958274776886924, 75.09886208192143897 ) ) ;
#19502=CARTESIAN_POINT ( 'NONE',  ( -3.753561863808878130, 218.3979405102790281, 12.09886208192143364 ) ) ;
#19503=CARTESIAN_POINT ( 'NONE',  ( -9.000000000000001776, 206.7692714347155629, 108.3323677711371857 ) ) ;
#19504=CIRCLE ( 'NONE', #2668, 0.9999999999999947820 ) ;
#19505=CARTESIAN_POINT ( 'NONE',  ( 6.139770520408368348, 198.4640165459539674, 20.45113791807855819 ) ) ;
#19506=CARTESIAN_POINT ( 'NONE',  ( 3.135527875058981895, 197.5041725223112792, 85.59886208192143897 ) ) ;
#19513=CARTESIAN_POINT ( 'NONE',  ( 8.000000000000008882, 207.0476921513415220, 66.99886208192144466 ) ) ;
#19522=CARTESIAN_POINT ( 'NONE',  ( -2.517493886308901807, 199.4062855549015012, 68.90113791807856103 ) ) ;
#19526=CARTESIAN_POINT ( 'NONE',  ( 8.015496119326595448, 204.4483345814782638, 55.14886208192145034 ) ) ;
#19528=CARTESIAN_POINT ( 'NONE',  ( -6.220909254589537696, 198.5229672870051161, 75.05113791807858092 ) ) ;
#19535=CARTESIAN_POINT ( 'NONE',  ( 3.662846001190051659, 195.5725841191953691, 53.60113791807856387 ) ) ;
#19537=CARTESIAN_POINT ( 'NONE',  ( -7.456977232089304408, 196.8216656703010301, 0.05113791807856556820 ) ) ;
#19538=CARTESIAN_POINT ( 'NONE',  ( -8.118202686958039038, 201.1607312380087080, 78.20113791807857240 ) ) ;
#19540=CARTESIAN_POINT ( 'NONE',  ( 3.662846001189864698, 218.4274158808046593, 36.39886208192143613 ) ) ;
#19541=CARTESIAN_POINT ( 'NONE',  ( -10.00000000000000711, 206.9523078486584495, 50.49886208192143044 ) ) ;
#19543=CARTESIAN_POINT ( 'NONE',  ( -12.01549611932652972, 203.1486557965464499, 90.35113791807857808 ) ) ;
#19544=CARTESIAN_POINT ( 'NONE',  ( 6.500168698208129925, 211.6636982574063381, 100.7011379180785866 ) ) ;
#19545=CARTESIAN_POINT ( 'NONE',  ( -3.044812012439970683, 197.4746971517856196, 55.89886208192143613 ) ) ;
#19547=CARTESIAN_POINT ( 'NONE',  ( -12.01549611932659722, 210.8513442034533227, 62.64886208192143613 ) ) ;
#19550=CARTESIAN_POINT ( 'NONE',  ( 4.903702542908435547, 213.8346818373419751, 39.54886208192143471 ) ) ;
#19557=CARTESIAN_POINT ( 'NONE',  ( -8.015496119326531499, 204.4483345814780364, 57.35113791807857098 ) ) ;
#19560=CARTESIAN_POINT ( 'NONE',  ( -6.220909254589682469, 215.4770327129946850, 41.94886208192144039 ) ) ;
#19566=CARTESIAN_POINT ( 'NONE',  ( -6.500168698208244500, 211.6636982574061676, 17.79886208192143471 ) ) ;
#19567=CARTESIAN_POINT ( 'NONE',  ( 0.05014649552810505201, 217.5146222423826714, 64.25113791807856956 ) ) ;
#19568=CARTESIAN_POINT ( 'NONE',  ( -6.220909254589537696, 198.5229672870051161, 48.05113791807858092 ) ) ;
#19570=CARTESIAN_POINT ( 'NONE',  ( 0.05014649552810505201, 217.5146222423826714, 22.25113791807856956 ) ) ;
#19571=CARTESIAN_POINT ( 'NONE',  ( -6.500168698208244500, 211.6636982574061676, 98.79886208192142760 ) ) ;
#19575=CARTESIAN_POINT ( 'NONE',  ( -3.753561863808691168, 195.6020594897209435, 23.90113791807857169 ) ) ;
#19576=AXIS2_PLACEMENT_3D ( 'NONE', #10510, #26328, #17698 ) ;
#19578=CARTESIAN_POINT ( 'NONE',  ( -0.05014649552810635652, 196.4853777576173002, 74.75113791807858377 ) ) ;
#19579=CARTESIAN_POINT ( 'NONE',  ( -8.062137200540920645, 212.9164362838581894, 42.80113791807857382 ) ) ;
#19582=CARTESIAN_POINT ( 'NONE',  ( -7.456977232089471386, 217.1783343296987709, 5.948862081921435063 ) ) ;
#19583=CARTESIAN_POINT ( 'NONE',  ( -0.05014649552828402690, 217.5146222423826714, 15.24886208192143400 ) ) ;
#19585=ORIENTED_EDGE ( 'NONE', *, *, #367, .F. ) ;
#19586=CARTESIAN_POINT ( 'NONE',  ( 12.00000000000000711, 206.9523078486586485, 53.00113791807857666 ) ) ;
#19587=CARTESIAN_POINT ( 'NONE',  ( 7.984503880673485376, 204.3529502787953902, 71.15113791807857524 ) ) ;
#19589=CARTESIAN_POINT ( 'NONE',  ( -9.984503880673420539, 203.7031108863293980, 32.34886208192143187 ) ) ;
#19593=CARTESIAN_POINT ( 'NONE',  ( 8.118202686958039038, 212.8392687619912635, 88.70113791807857240 ) ) ;
#19600=CARTESIAN_POINT ( 'NONE',  ( -0.05014649552807731031, 198.5883022060938572, 20.75113791807856600 ) ) ;
#19602=CARTESIAN_POINT ( 'NONE',  ( -3.135527875058982783, 216.4958274776886924, 3.098862081921434974 ) ) ;
#19605=CARTESIAN_POINT ( 'NONE',  ( 6.444103211791042618, 202.2591342207267644, 53.30113791807858092 ) ) ;
#19608=CARTESIAN_POINT ( 'NONE',  ( 8.118202686958138514, 201.1607312380088501, 91.29886208192144181 ) ) ;
#19610=CARTESIAN_POINT ( 'NONE',  ( -0.05014649552810635652, 196.4853777576173002, 29.75113791807856956 ) ) ;
#19611=FACE_OUTER_BOUND ( 'NONE', #11959, .T. ) ;
#19612=CARTESIAN_POINT ( 'NONE',  ( 6.139770520408368348, 198.4640165459539674, 14.45113791807856352 ) ) ;
#19618=CARTESIAN_POINT ( 'NONE',  ( -3.135527875058821579, 197.5041725223112223, 95.90113791807858945 ) ) ;
#19621=CARTESIAN_POINT ( 'NONE',  ( 6.139770520408368348, 198.4640165459539674, 38.45113791807855819 ) ) ;
#19627=CARTESIAN_POINT ( 'NONE',  ( 12.01549611932652972, 210.8513442034534933, 22.85113791807856742 ) ) ;
#19631=CARTESIAN_POINT ( 'NONE',  ( -7.375838497908014268, 196.7627149292498530, 44.04886208192143471 ) ) ;
#19632=CARTESIAN_POINT ( 'NONE',  ( -8.118202686958039038, 201.1607312380087080, 3.201137918078566180 ) ) ;
#19633=CARTESIAN_POINT ( 'NONE',  ( 9.984503880673470277, 203.7031108863295401, 62.15113791807856813 ) ) ;
#19634=CARTESIAN_POINT ( 'NONE',  ( 4.984841277089891776, 200.2242689037093726, 13.44886208192143684 ) ) ;
#19640=CARTESIAN_POINT ( 'NONE',  ( 8.015496119326595448, 204.4483345814782638, 97.14886208192146455 ) ) ;
#19643=CARTESIAN_POINT ( 'NONE',  ( -8.000000000000008882, 207.0476921513413515, 36.50113791807857666 ) ) ;
#19648=CARTESIAN_POINT ( 'NONE',  ( 8.062137200540920645, 201.0835637161417822, -0.6988620819214342861 ) ) ;
#19649=CARTESIAN_POINT ( 'NONE',  ( -0.05014649552828403384, 217.5146222423826714, 66.24886208192143044 ) ) ;
#19652=CARTESIAN_POINT ( 'NONE',  ( -6.220909254589537696, 198.5229672870051161, 3.051137918078564937 ) ) ;
#19655=CARTESIAN_POINT ( 'NONE',  ( 6.444103211790928043, 211.7408657792734061, 78.69886208192143329 ) ) ;
#19657=DIRECTION ( 'NONE',  ( 0.000000000000000000, -0.04769215134144040580, 0.9988620819214356628 ) ) ;
#19659=CARTESIAN_POINT ( 'NONE',  ( -9.984503880673475606, 210.2968891136704315, 24.65113791807856458 ) ) ;
#19664=CARTESIAN_POINT ( 'NONE',  ( 11.98450388067348271, 203.0532714938637753, 89.15113791807856103 ) ) ;
#19667=CARTESIAN_POINT ( 'NONE',  ( -3.753561863808878130, 218.3979405102790281, 69.09886208192143897 ) ) ;
#19668=CARTESIAN_POINT ( 'NONE',  ( -6.220909254589682469, 215.4770327129947134, 74.94886208192143329 ) ) ;
#19669=CARTESIAN_POINT ( 'NONE',  ( 9.736236675708031640, 199.9851607334238963, 16.29886208192143471 ) ) ;
#19671=CARTESIAN_POINT ( 'NONE',  ( 3.135527875058820690, 216.4958274776887492, 34.40113791807856813 ) ) ;
#19673=CARTESIAN_POINT ( 'NONE',  ( -6.139770520408224463, 198.4640165459539389, 89.04886208192139918 ) ) ;
#19676=CARTESIAN_POINT ( 'NONE',  ( -9.945352646237287431, 205.9548993908332193, 104.4520571433695579 ) ) ;
#19677=CARTESIAN_POINT ( 'NONE',  ( -6.444103211790928043, 202.2591342207265939, 74.19886208192143329 ) ) ;
#19685=CARTESIAN_POINT ( 'NONE',  ( 8.000000000000008882, 206.9523078486586485, 74.00113791807856956 ) ) ;
#19690=CARTESIAN_POINT ( 'NONE',  ( 4.903702542908435547, 213.8346818373419751, 51.54886208192144181 ) ) ;
#19696=CARTESIAN_POINT ( 'NONE',  ( 7.456977232089302632, 217.1783343296989131, 58.55113791807858092 ) ) ;
#19698=CARTESIAN_POINT ( 'NONE',  ( -0.05014649552807705357, 194.3824533091408000, 2.751137918078565114 ) ) ;
#19699=CARTESIAN_POINT ( 'NONE',  ( 10.00000000000000711, 206.9523078486586201, 74.00113791807858377 ) ) ;
#19700=CARTESIAN_POINT ( 'NONE',  ( 9.736236675708031640, 199.9851607334238963, 40.29886208192143471 ) ) ;
#19702=CARTESIAN_POINT ( 'NONE',  ( 3.135527875058981895, 197.5041725223112792, 49.59886208192143897 ) ) ;
#19704=CARTESIAN_POINT ( 'NONE',  ( 12.00000000000000711, 206.9523078486586485, 86.00113791807856956 ) ) ;
#19705=CARTESIAN_POINT ( 'NONE',  ( -6.500168698208129925, 202.3363017425936050, 96.20113791807858661 ) ) ;
#19706=CARTESIAN_POINT ( 'NONE',  ( 9.984503880673420539, 210.2968891136705167, 60.84886208192142476 ) ) ;
#19708=CARTESIAN_POINT ( 'NONE',  ( -9.736236675708031640, 214.0148392665760753, 68.79886208192144181 ) ) ;
#19712=CARTESIAN_POINT ( 'NONE',  ( 8.000000000000008882, 207.0476921513415220, 39.99886208192145176 ) ) ;
#19719=CARTESIAN_POINT ( 'NONE',  ( 4.984841277089725686, 213.7757310962907411, 61.55113791807858092 ) ) ;
#19721=CARTESIAN_POINT ( 'NONE',  ( 6.139770520408223575, 215.5359834540460611, 39.54886208192143471 ) ) ;
#19726=( LENGTH_UNIT ( ) NAMED_UNIT ( * ) SI_UNIT ( .MILLI., .METRE. ) );
#19729=CARTESIAN_POINT ( 'NONE',  ( 4.984841277089891776, 200.2242689037093726, 22.44886208192143329 ) ) ;
#19730=CARTESIAN_POINT ( 'NONE',  ( -9.984503880673473830, 210.2968891136704315, 63.65113791807857524 ) ) ;
#19731=CARTESIAN_POINT ( 'NONE',  ( 6.139770520408368348, 198.4640165459539674, 44.45113791807855819 ) ) ;
#19734=CARTESIAN_POINT ( 'NONE',  ( 10.01549611932653860, 210.2015048109876716, 19.85113791807856387 ) ) ;
#19735=CARTESIAN_POINT ( 'NONE',  ( 7.984503880673485376, 204.3529502787953902, 5.151137918078566358 ) ) ;
#19740=CARTESIAN_POINT ( 'NONE',  ( 9.680171189290831535, 199.9079932115568852, 26.30113791807856316 ) ) ;
#19743=CARTESIAN_POINT ( 'NONE',  ( 8.118202686958039038, 212.8392687619912635, 73.70113791807857240 ) ) ;
#19744=CARTESIAN_POINT ( 'NONE',  ( -0.05014649552810635652, 196.4853777576173002, 44.75113791807856956 ) ) ;
#19747=CARTESIAN_POINT ( 'NONE',  ( 7.375838497908012492, 217.2372850707501186, 12.54886208192143826 ) ) ;
#19748=CARTESIAN_POINT ( 'NONE',  ( 9.984503880673420539, 210.2968891136705736, 15.84886208192143719 ) ) ;
#19751=CARTESIAN_POINT ( 'NONE',  ( -7.456977232089304408, 196.8216656703010301, 60.05113791807858092 ) ) ;
#19752=CARTESIAN_POINT ( 'NONE',  ( 6.500168698208129925, 211.6636982574063381, 64.70113791807857240 ) ) ;
#19754=CARTESIAN_POINT ( 'NONE',  ( 3.135527875058981895, 197.5041725223112792, 34.59886208192143897 ) ) ;
#19758=CARTESIAN_POINT ( 'NONE',  ( -9.984503880673473830, 210.2968891136704315, 90.65113791807854682 ) ) ;
#19764=CARTESIAN_POINT ( 'NONE',  ( 0.05014649552807626948, 215.4116977939061144, 37.25113791807857666 ) ) ;
#19767=CARTESIAN_POINT ( 'NONE',  ( -8.118202686958138514, 212.8392687619910930, 11.79886208192143471 ) ) ;
#19771=CARTESIAN_POINT ( 'NONE',  ( -0.05014649552807731031, 198.5883022060938572, 53.75113791807857666 ) ) ;
#19774=CARTESIAN_POINT ( 'NONE',  ( 10.01549611932659545, 203.7984951890123853, 103.1488620819214077 ) ) ;
#19776=CARTESIAN_POINT ( 'NONE',  ( 3.044812012440130555, 197.4746971517856764, 35.60113791807857098 ) ) ;
#19778=EDGE_CURVE ( 'NONE', #22743, #13301, #4030, .T. ) ;
#19780=CARTESIAN_POINT ( 'NONE',  ( 0.05014649552810505201, 217.5146222423826714, 13.25113791807856778 ) ) ;
#19785=CARTESIAN_POINT ( 'NONE',  ( -10.01549611932653860, 203.7984951890123284, 102.3511379180785781 ) ) ;
#19790=CARTESIAN_POINT ( 'NONE',  ( -10.01549611932653860, 203.7984951890123284, 42.35113791807855677 ) ) ;
#19797=CARTESIAN_POINT ( 'NONE',  ( 0.05014649552807549926, 219.6175466908591716, 31.25113791807856956 ) ) ;
#19803=CARTESIAN_POINT ( 'NONE',  ( 7.375838497908012492, 217.2372850707501186, 42.54886208192143471 ) ) ;
#19805=CARTESIAN_POINT ( 'NONE',  ( -8.118202686958039038, 201.1607312380087080, 63.20113791807857240 ) ) ;
#19806=CARTESIAN_POINT ( 'NONE',  ( -2.517493886309087880, 214.5937144450984135, 27.09886208192143897 ) ) ;
#19809=CARTESIAN_POINT ( 'NONE',  ( 4.984841277089725686, 213.7757310962907411, 1.551137918078566047 ) ) ;
#19811=CARTESIAN_POINT ( 'NONE',  ( 0.05014649552828288198, 194.3824533091408000, 85.74886208192143044 ) ) ;
#19817=CARTESIAN_POINT ( 'NONE',  ( -6.220909254589682469, 215.4770327129946850, 59.94886208192141908 ) ) ;
#19820=CARTESIAN_POINT ( 'NONE',  ( 8.118202686958039038, 212.8392687619912635, 4.701137918078565292 ) ) ;
#19824=CARTESIAN_POINT ( 'NONE',  ( -7.984503880673422316, 204.3529502787951628, 83.34886208192143897 ) ) ;
#19827=CARTESIAN_POINT ( 'NONE',  ( 3.753561863808876797, 195.6020594897209719, 82.59886208192143897 ) ) ;
#19829=CARTESIAN_POINT ( 'NONE',  ( -10.01549611932653860, 203.7984951890123000, 18.35113791807856742 ) ) ;
#19833=CARTESIAN_POINT ( 'NONE',  ( -9.736236675707914401, 199.9851607334237542, 87.20113791807858661 ) ) ;
#19836=CARTESIAN_POINT ( 'NONE',  ( 9.736236675708031640, 199.9851607334238963, 67.29886208192144181 ) ) ;
#19837=CARTESIAN_POINT ( 'NONE',  ( 6.220909254589680693, 198.5229672870052582, 76.44886208192143329 ) ) ;
#19838=CARTESIAN_POINT ( 'NONE',  ( -7.375838497908014268, 196.7627149292498530, 11.04886208192143648 ) ) ;
#19840=CARTESIAN_POINT ( 'NONE',  ( -3.135527875058821579, 197.5041725223112223, 29.90113791807856813 ) ) ;
#19842=CARTESIAN_POINT ( 'NONE',  ( -6.220909254589682469, 215.4770327129946850, 95.94886208192143329 ) ) ;
#19846=CARTESIAN_POINT ( 'NONE',  ( 0.05014649552828262524, 198.5883022060938572, 70.74886208192144466 ) ) ;
#19853=CARTESIAN_POINT ( 'NONE',  ( -4.903702542908602524, 213.8346818373418898, 78.95113791807858661 ) ) ;
#19856=CARTESIAN_POINT ( 'NONE',  ( -4.984841277089891776, 213.7757310962905990, 56.94886208192144039 ) ) ;
#19862=CARTESIAN_POINT ( 'NONE',  ( -12.01549611932652972, 203.1486557965464499, 60.35113791807857098 ) ) ;
#19864=CARTESIAN_POINT ( 'NONE',  ( 6.139770520408368348, 198.4640165459539674, 101.4511379180785866 ) ) ;
#19867=CARTESIAN_POINT ( 'NONE',  ( 8.062137200540920645, 201.0835637161417822, 74.30113791807858092 ) ) ;
#19868=CARTESIAN_POINT ( 'NONE',  ( -12.01549611932659722, 210.8513442034533227, 38.64886208192143613 ) ) ;
#19869=CARTESIAN_POINT ( 'NONE',  ( -3.044812012439970683, 197.4746971517856196, 49.89886208192143613 ) ) ;
#19871=CARTESIAN_POINT ( 'NONE',  ( 11.98450388067348271, 203.0532714938637753, 83.15113791807856103 ) ) ;
#19873=CARTESIAN_POINT ( 'NONE',  ( 6.139770520408368348, 198.4640165459539674, 2.451137918078566180 ) ) ;
#19874=CARTESIAN_POINT ( 'NONE',  ( 10.01549611932659545, 203.7984951890123853, 58.14886208192142192 ) ) ;
#19877=CARTESIAN_POINT ( 'NONE',  ( -7.375838497908014268, 196.7627149292498530, 74.04886208192142760 ) ) ;
#19880=CARTESIAN_POINT ( 'NONE',  ( 0.05014649552828262524, 198.5883022060938572, 40.74886208192143755 ) ) ;
#19886=CARTESIAN_POINT ( 'NONE',  ( 8.062137200540822946, 212.9164362838583315, 39.69886208192143329 ) ) ;
#19892=CARTESIAN_POINT ( 'NONE',  ( 4.984841277089891776, 200.2242689037093726, 25.44886208192143684 ) ) ;
#19893=CARTESIAN_POINT ( 'NONE',  ( -3.135527875058821579, 197.5041725223112223, 65.90113791807857524 ) ) ;
#19894=CARTESIAN_POINT ( 'NONE',  ( -8.062137200540920645, 212.9164362838581894, 45.80113791807856671 ) ) ;
#19897=CARTESIAN_POINT ( 'NONE',  ( -3.044812012440131443, 216.5253028482142952, 19.10113791807856742 ) ) ;
#19898=CARTESIAN_POINT ( 'NONE',  ( 6.500168698208129925, 211.6636982574063381, 7.701137918078567068 ) ) ;
#19902=CARTESIAN_POINT ( 'NONE',  ( 3.753561863808689836, 218.3979405102790565, 28.40113791807856813 ) ) ;
#19904=CARTESIAN_POINT ( 'NONE',  ( 3.135527875058820690, 216.4958274776887492, 79.40113791807857524 ) ) ;
#19906=CARTESIAN_POINT ( 'NONE',  ( -10.01549611932653860, 203.7984951890123000, 48.35113791807857098 ) ) ;
#19908=DIRECTION ( 'NONE',  ( -0.9998603841633338929, 0.01669062914075312987, 0.0007969188393214247284 ) ) ;
#19909=CARTESIAN_POINT ( 'NONE',  ( 12.01549611932659367, 203.1486557965466773, 10.14886208192143435 ) ) ;
#19910=CARTESIAN_POINT ( 'NONE',  ( -10.00000000000000711, 206.9523078486584495, 17.49886208192143400 ) ) ;
#19913=CARTESIAN_POINT ( 'NONE',  ( 12.00000000000000711, 206.9523078486586485, 62.00113791807856956 ) ) ;
#19914=CARTESIAN_POINT ( 'NONE',  ( 4.903702542908601636, 200.1653181626581102, 74.45113791807855819 ) ) ;
#19915=CARTESIAN_POINT ( 'NONE',  ( -8.062137200540822946, 201.0835637161416400, 32.19886208192143329 ) ) ;
#19921=VERTEX_POINT ( 'NONE', #33218 ) ;
#19926=CARTESIAN_POINT ( 'NONE',  ( -8.015496119326531499, 204.4483345814780364, 30.35113791807856742 ) ) ;
#19930=CARTESIAN_POINT ( 'NONE',  ( -10.00000000000000711, 206.9523078486584495, 17.49886208192143400 ) ) ;
#19933=CARTESIAN_POINT ( 'NONE',  ( 2.517493886308900919, 214.5937144450984420, 46.40113791807856813 ) ) ;
#19937=CARTESIAN_POINT ( 'NONE',  ( -10.05084501415679732, 217.6133941545940047, 104.9910338291041683 ) ) ;
#19940=CARTESIAN_POINT ( 'NONE',  ( -9.984503880673473830, 210.2968891136704315, 36.65113791807855392 ) ) ;
#19942=CARTESIAN_POINT ( 'NONE',  ( 0.05014649552810505201, 217.5146222423826714, 19.25113791807856600 ) ) ;
#19948=CARTESIAN_POINT ( 'NONE',  ( 9.680171189290831535, 199.9079932115568852, -0.6988620819214345081 ) ) ;
#19951=CARTESIAN_POINT ( 'NONE',  ( -10.00000000000000711, 207.0476921513413515, 48.50113791807856956 ) ) ;
#19959=CARTESIAN_POINT ( 'NONE',  ( -12.00000000000000711, 207.0476921513413515, 30.50113791807856600 ) ) ;
#19961=CARTESIAN_POINT ( 'NONE',  ( -7.456977232089471386, 217.1783343296987709, 101.9488620819214475 ) ) ;
#19964=CARTESIAN_POINT ( 'NONE',  ( 10.00000000000000711, 206.9523078486586201, 65.00113791807856956 ) ) ;
#19965=CARTESIAN_POINT ( 'NONE',  ( -0.05014649552828365914, 215.4116977939061144, 21.24886208192143755 ) ) ;
#19970=CARTESIAN_POINT ( 'NONE',  ( -6.444103211791042618, 211.7408657792732356, 3.801137918078566269 ) ) ;
#19973=CARTESIAN_POINT ( 'NONE',  ( -9.736236675708031640, 214.0148392665760753, 86.79886208192142760 ) ) ;
#19980=CARTESIAN_POINT ( 'NONE',  ( 8.062137200540822946, 212.9164362838583315, 72.69886208192143329 ) ) ;
#19984=CARTESIAN_POINT ( 'NONE',  ( 3.135527875058820690, 216.4958274776887492, 7.401137918078566358 ) ) ;
#19987=CARTESIAN_POINT ( 'NONE',  ( -10.01549611932653860, 203.7984951890123284, 87.35113791807854966 ) ) ;
#19989=CARTESIAN_POINT ( 'NONE',  ( 8.000000000000008882, 207.0476921513415220, 78.99886208192144466 ) ) ;
#19993=CARTESIAN_POINT ( 'NONE',  ( 7.375838497908012492, 217.2372850707501186, 87.54886208192142760 ) ) ;
#19996=CARTESIAN_POINT ( 'NONE',  ( -6.220909254589537696, 198.5229672870051445, 24.05113791807856316 ) ) ;
#20001=CARTESIAN_POINT ( 'NONE',  ( 7.375838497908181246, 196.7627149292499666, 89.45113791807857240 ) ) ;
#20005=CARTESIAN_POINT ( 'NONE',  ( -7.375838497908014268, 196.7627149292498530, 71.04886208192142760 ) ) ;
#20006=CARTESIAN_POINT ( 'NONE',  ( 6.139770520408223575, 215.5359834540460611, 72.54886208192142760 ) ) ;
#20007=CARTESIAN_POINT ( 'NONE',  ( 3.662846001189864698, 218.4274158808046593, 18.39886208192143613 ) ) ;
#20009=CARTESIAN_POINT ( 'NONE',  ( -9.984503880673473830, 210.2968891136704315, 33.65113791807856813 ) ) ;
#20011=CARTESIAN_POINT ( 'NONE',  ( 10.00000000000000711, 207.0476921513415220, 96.99886208192143044 ) ) ;
#20014=FACE_OUTER_BOUND ( 'NONE', #5434, .T. ) ;
#20015=CARTESIAN_POINT ( 'NONE',  ( 6.444103211790928043, 211.7408657792734061, 78.69886208192143329 ) ) ;
#20025=CARTESIAN_POINT ( 'NONE',  ( 2.517493886308900919, 214.5937144450984420, 82.40113791807856103 ) ) ;
#20030=CARTESIAN_POINT ( 'NONE',  ( -0.05014649552828365914, 215.4116977939061144, 54.24886208192144466 ) ) ;
#20036=CARTESIAN_POINT ( 'NONE',  ( -11.98450388067348804, 210.9467285061362247, 54.65113791807857524 ) ) ;
#20039=CARTESIAN_POINT ( 'NONE',  ( 10.01549611932653860, 210.2015048109876716, 100.8511379180785497 ) ) ;
#20040=CARTESIAN_POINT ( 'NONE',  ( 10.01549611932653860, 210.2015048109876716, 79.85113791807856387 ) ) ;
#20042=CARTESIAN_POINT ( 'NONE',  ( -9.680171189290716072, 199.9079932115567146, 44.19886208192143329 ) ) ;
#20043=CARTESIAN_POINT ( 'NONE',  ( 10.00000000000000711, 207.0476921513415220, 48.99886208192143044 ) ) ;
#20045=CARTESIAN_POINT ( 'NONE',  ( 3.753561863808689836, 218.3979405102790565, 82.40113791807856103 ) ) ;
#20047=CARTESIAN_POINT ( 'NONE',  ( -10.01549611932653860, 203.7984951890123284, 3.351137918078566091 ) ) ;
#20048=CARTESIAN_POINT ( 'NONE',  ( 8.118202686958138514, 201.1607312380088501, 70.29886208192142760 ) ) ;
#20051=CARTESIAN_POINT ( 'NONE',  ( 7.456977232089471386, 196.8216656703012006, 73.44886208192143329 ) ) ;
#20054=CARTESIAN_POINT ( 'NONE',  ( -6.444103211790928043, 202.2591342207265939, 56.19886208192144039 ) ) ;
#20062=CARTESIAN_POINT ( 'NONE',  ( 3.044812012439969795, 216.5253028482143520, 45.39886208192143613 ) ) ;
#20066=CARTESIAN_POINT ( 'NONE',  ( 8.000000000000008882, 206.9523078486586485, 11.00113791807856600 ) ) ;
#20070=CARTESIAN_POINT ( 'NONE',  ( 4.984841277089891776, 200.2242689037093726, 28.44886208192142973 ) ) ;
#20071=CARTESIAN_POINT ( 'NONE',  ( -10.00000000000000711, 207.0476921513413515, 60.50113791807857666 ) ) ;
#20072=CARTESIAN_POINT ( 'NONE',  ( 9.984503880673470277, 203.7031108863295401, 47.15113791807857524 ) ) ;
#20075=CARTESIAN_POINT ( 'NONE',  ( 6.220909254589536808, 215.4770327129947702, 16.55113791807857027 ) ) ;
#20076=CARTESIAN_POINT ( 'NONE',  ( -2.426778023690262742, 214.6231898156240163, 7.101137918078566535 ) ) ;
#20080=CARTESIAN_POINT ( 'NONE',  ( 7.456977232089302632, 217.1783343296989131, 28.55113791807857027 ) ) ;
#20082=CARTESIAN_POINT ( 'NONE',  ( -6.139770520408369237, 215.5359834540460042, 72.95113791807854398 ) ) ;
#20083=CARTESIAN_POINT ( 'NONE',  ( 8.062137200540920645, 201.0835637161417822, 53.30113791807857382 ) ) ;
#20086=CARTESIAN_POINT ( 'NONE',  ( 9.736236675708031640, 199.9851607334238963, 10.29886208192143471 ) ) ;
#20087=CARTESIAN_POINT ( 'NONE',  ( -0.05014649552828402690, 217.5146222423826714, 21.24886208192143400 ) ) ;
#20090=CARTESIAN_POINT ( 'NONE',  ( -7.456977232089304408, 196.8216656703010301, 54.05113791807856671 ) ) ;
#20092=CARTESIAN_POINT ( 'NONE',  ( 4.903702542908601636, 200.1653181626581102, 77.45113791807855819 ) ) ;
#20093=CARTESIAN_POINT ( 'NONE',  ( 6.139770520408223575, 215.5359834540460611, 45.54886208192144181 ) ) ;
#20102=CARTESIAN_POINT ( 'NONE',  ( -2.426778023690262742, 214.6231898156240163, 31.10113791807856742 ) ) ;
#20105=CARTESIAN_POINT ( 'NONE',  ( 8.062137200540822946, 212.9164362838583315, 9.698862081921435063 ) ) ;
#20108=CARTESIAN_POINT ( 'NONE',  ( -0.05014649552807731031, 198.5883022060938572, 59.75113791807857666 ) ) ;
#20112=CARTESIAN_POINT ( 'NONE',  ( -6.139770520408224463, 198.4640165459539389, 101.0488620819214134 ) ) ;
#20114=CARTESIAN_POINT ( 'NONE',  ( 3.135527875058820690, 216.4958274776887492, 34.40113791807856813 ) ) ;
#20116=CARTESIAN_POINT ( 'NONE',  ( -3.044812012440131443, 216.5253028482142952, 22.10113791807856742 ) ) ;
#20120=CARTESIAN_POINT ( 'NONE',  ( 10.01549611932653860, 210.2015048109876716, 100.8511379180785497 ) ) ;
#20123=CARTESIAN_POINT ( 'NONE',  ( -10.00000000000000711, 207.0476921513413515, 51.50113791807857666 ) ) ;
#20129=CARTESIAN_POINT ( 'NONE',  ( 7.375838497908181246, 196.7627149292499666, 32.45113791807856529 ) ) ;
#20131=CARTESIAN_POINT ( 'NONE',  ( -3.044812012439970683, 197.4746971517856196, 7.898862081921434353 ) ) ;
#20134=CARTESIAN_POINT ( 'NONE',  ( 9.984503880673470277, 203.7031108863295401, 2.151137918078565914 ) ) ;
#20135=CARTESIAN_POINT ( 'NONE',  ( 8.062137200540920645, 201.0835637161417822, 59.30113791807857382 ) ) ;
#20137=VERTEX_POINT ( 'NONE', #7504 ) ;
#20138=CARTESIAN_POINT ( 'NONE',  ( 0.05014649552828262524, 198.5883022060938572, 25.74886208192143755 ) ) ;
#20141=CARTESIAN_POINT ( 'NONE',  ( -2.517493886308901807, 199.4062855549015012, -0.09886208192143407236 ) ) ;
#20144=CARTESIAN_POINT ( 'NONE',  ( -9.736236675708031640, 214.0148392665760753, 89.79886208192142760 ) ) ;
#20149=CARTESIAN_POINT ( 'NONE',  ( -10.00000000000000711, 206.9523078486584495, 71.49886208192144466 ) ) ;
#20152=CARTESIAN_POINT ( 'NONE',  ( -6.139770520408369237, 215.5359834540460042, 0.9511379180785658471 ) ) ;
#20156=CARTESIAN_POINT ( 'NONE',  ( -10.00000000000000711, 207.0476921513413515, 87.50113791807858377 ) ) ;
#20159=CARTESIAN_POINT ( 'NONE',  ( -8.118202686958039038, 201.1607312380087080, 78.20113791807857240 ) ) ;
#20162=CARTESIAN_POINT ( 'NONE',  ( 12.01549611932659367, 203.1486557965466773, 91.14886208192143613 ) ) ;
#20164=CARTESIAN_POINT ( 'NONE',  ( -3.135527875058821579, 197.5041725223112223, 32.90113791807857524 ) ) ;
#20168=CARTESIAN_POINT ( 'NONE',  ( -3.662846001190052991, 218.4274158808045740, 91.10113791807859229 ) ) ;
#20172=CARTESIAN_POINT ( 'NONE',  ( -3.044812012439970683, 197.4746971517856196, 82.89886208192145034 ) ) ;
#20174=CARTESIAN_POINT ( 'NONE',  ( 11.98450388067341876, 210.9467285061363953, 9.848862081921433642 ) ) ;
#20176=CARTESIAN_POINT ( 'NONE',  ( 6.139770520408368348, 198.4640165459539674, 32.45113791807856529 ) ) ;
#20179=CARTESIAN_POINT ( 'NONE',  ( -3.044812012439970683, 197.4746971517856196, 97.89886208192145034 ) ) ;
#20183=CARTESIAN_POINT ( 'NONE',  ( 0.05014649552828262524, 198.5883022060938572, 82.74886208192144466 ) ) ;
#20191=CARTESIAN_POINT ( 'NONE',  ( -8.000000000000008882, 207.0476921513413515, 78.50113791807856956 ) ) ;
#20195=CARTESIAN_POINT ( 'NONE',  ( -4.903702542908436435, 200.1653181626580249, 56.04886208192144181 ) ) ;
#20203=CARTESIAN_POINT ( 'NONE',  ( -9.680171189290831535, 214.0920067884431148, 60.80113791807858092 ) ) ;
#20205=CARTESIAN_POINT ( 'NONE',  ( 12.00000000000000711, 206.9523078486586485, 2.001137918078565114 ) ) ;
#20207=CARTESIAN_POINT ( 'NONE',  ( -8.062137200540920645, 212.9164362838581894, 75.80113791807858092 ) ) ;
#20208=CARTESIAN_POINT ( 'NONE',  ( 12.01549611932659367, 203.1486557965466773, 46.14886208192143613 ) ) ;
#20209=CARTESIAN_POINT ( 'NONE',  ( 6.139770520408223575, 215.5359834540460611, 51.54886208192142760 ) ) ;
#20211=CARTESIAN_POINT ( 'NONE',  ( 12.01549611932652972, 210.8513442034534933, 82.85113791807857808 ) ) ;
#20213=CARTESIAN_POINT ( 'NONE',  ( 10.01549611932653860, 210.2015048109876716, 7.851137918078566535 ) ) ;
#20215=CARTESIAN_POINT ( 'NONE',  ( 6.220909254589681581, 198.5229672870052582, 67.44886208192143329 ) ) ;
#20218=CARTESIAN_POINT ( 'NONE',  ( 7.375838497908012492, 217.2372850707501186, 75.54886208192142760 ) ) ;
#20222=CARTESIAN_POINT ( 'NONE',  ( 2.426778023690075337, 214.6231898156240447, 51.39886208192145745 ) ) ;
#20230=CARTESIAN_POINT ( 'NONE',  ( -10.00000000000000711, 206.9523078486584495, 38.49886208192143755 ) ) ;
#20236=CARTESIAN_POINT ( 'NONE',  ( -2.426778023690076225, 199.3768101843759553, 28.89886208192143613 ) ) ;
#20237=CARTESIAN_POINT ( 'NONE',  ( -6.139770520408369237, 215.5359834540460042, 72.95113791807854398 ) ) ;
#20239=CARTESIAN_POINT ( 'NONE',  ( 9.984503880673470277, 203.7031108863295401, 50.15113791807855392 ) ) ;
#20240=CARTESIAN_POINT ( 'NONE',  ( 3.044812012440130555, 197.4746971517856764, 14.60113791807856565 ) ) ;
#20241=CARTESIAN_POINT ( 'NONE',  ( 6.500168698208129925, 211.6636982574063381, 4.701137918078565292 ) ) ;
#20244=CARTESIAN_POINT ( 'NONE',  ( 9.736236675707914401, 214.0148392665762458, 31.70113791807856529 ) ) ;
#20247=CARTESIAN_POINT ( 'NONE',  ( 8.118202686958039038, 212.8392687619912635, 76.70113791807857240 ) ) ;
#20248=CARTESIAN_POINT ( 'NONE',  ( -3.135527875058821579, 197.5041725223112223, 53.90113791807857524 ) ) ;
#20251=CARTESIAN_POINT ( 'NONE',  ( 3.753561863808876797, 195.6020594897209719, 16.59886208192143187 ) ) ;
#20252=CARTESIAN_POINT ( 'NONE',  ( 9.984503880673420539, 210.2968891136705736, 21.84886208192143542 ) ) ;
#20256=CARTESIAN_POINT ( 'NONE',  ( -9.680171189290831535, 214.0920067884431148, 54.80113791807857382 ) ) ;
#20257=CARTESIAN_POINT ( 'NONE',  ( -8.015496119326531499, 204.4483345814780364, 75.35113791807856387 ) ) ;
#20259=CARTESIAN_POINT ( 'NONE',  ( 6.220909254589681581, 198.5229672870052582, 43.44886208192143329 ) ) ;
#20268=CARTESIAN_POINT ( 'NONE',  ( -6.444103211791042618, 211.7408657792732356, 33.80113791807857382 ) ) ;
#20270=CARTESIAN_POINT ( 'NONE',  ( -0.05014649552828403384, 217.5146222423826714, 9.248862081921432221 ) ) ;
#20273=CARTESIAN_POINT ( 'NONE',  ( 0.05014649552807626948, 215.4116977939061144, 64.25113791807856956 ) ) ;
#20275=AXIS2_PLACEMENT_3D ( 'NONE', #22249, #32970, #14242 ) ;
#20277=CARTESIAN_POINT ( 'NONE',  ( -10.10169002831358576, 228.2744804605295315, 105.4832055762869061 ) ) ;
#20280=CARTESIAN_POINT ( 'NONE',  ( -10.01549611932653860, 203.7984951890123284, 45.35113791807857808 ) ) ;
#20282=CARTESIAN_POINT ( 'NONE',  ( 10.01549611932653860, 210.2015048109876716, 19.85113791807856387 ) ) ;
#20283=CARTESIAN_POINT ( 'NONE',  ( 3.135527875058981895, 197.5041725223112792, 103.5988620819214390 ) ) ;
#20288=CARTESIAN_POINT ( 'NONE',  ( 3.753561863808689836, 218.3979405102790565, 4.401137918078566358 ) ) ;
#20291=CARTESIAN_POINT ( 'NONE',  ( 3.135527875058820690, 216.4958274776887492, 49.40113791807857524 ) ) ;
#20298=CARTESIAN_POINT ( 'NONE',  ( -11.98450388067348804, 210.9467285061362247, 30.65113791807856458 ) ) ;
#20301=CARTESIAN_POINT ( 'NONE',  ( 0.05014649552828275708, 196.4853777576173002, 7.748862081921435774 ) ) ;
#20305=CARTESIAN_POINT ( 'NONE',  ( 3.044812012440130555, 197.4746971517856764, 8.601137918078565647 ) ) ;
#20306=CARTESIAN_POINT ( 'NONE',  ( -10.00000000000000711, 207.0476921513413515, 60.50113791807857666 ) ) ;
#20309=CARTESIAN_POINT ( 'NONE',  ( 8.015496119326595448, 204.4483345814782638, 22.14886208192143613 ) ) ;
#20313=CARTESIAN_POINT ( 'NONE',  ( -2.426778023690262742, 214.6231898156240163, 7.101137918078566535 ) ) ;
#20314=CARTESIAN_POINT ( 'NONE',  ( 9.736236675708031640, 199.9851607334238963, 85.29886208192145602 ) ) ;
#20319=CARTESIAN_POINT ( 'NONE',  ( 8.118202686958039038, 212.8392687619912635, 1.701137918078565736 ) ) ;
#20322=CARTESIAN_POINT ( 'NONE',  ( 8.118202686958138514, 201.1607312380088501, 70.29886208192142760 ) ) ;
#20325=CARTESIAN_POINT ( 'NONE',  ( 3.044812012440130555, 197.4746971517856764, 2.601137918078566091 ) ) ;
#20330=CARTESIAN_POINT ( 'NONE',  ( -6.139770520408369237, 215.5359834540460042, 87.95113791807858661 ) ) ;
#20332=CARTESIAN_POINT ( 'NONE',  ( -6.220909254589537696, 198.5229672870051161, 72.05113791807853829 ) ) ;
#20336=CARTESIAN_POINT ( 'NONE',  ( -12.01549611932659722, 210.8513442034533227, 83.64886208192143613 ) ) ;
#20339=CARTESIAN_POINT ( 'NONE',  ( 10.00000000000000711, 206.9523078486586201, 26.00113791807856956 ) ) ;
#20343=CARTESIAN_POINT ( 'NONE',  ( -9.680171189290831535, 214.0920067884431148, 96.80113791807858092 ) ) ;
#20348=CARTESIAN_POINT ( 'NONE',  ( -10.00000000000000711, 206.9523078486584495, 83.49886208192143044 ) ) ;
#20349=CARTESIAN_POINT ( 'NONE',  ( -12.01549611932659722, 210.8513442034533227, 23.64886208192143968 ) ) ;
#20352=CARTESIAN_POINT ( 'NONE',  ( 8.062137200540920645, 201.0835637161417822, 29.30113791807857027 ) ) ;
#20354=CARTESIAN_POINT ( 'NONE',  ( 3.044812012439969795, 216.5253028482143520, 99.39886208192145034 ) ) ;
#20360=CARTESIAN_POINT ( 'NONE',  ( 6.444103211790928043, 211.7408657792734061, 81.69886208192144750 ) ) ;
#20366=CARTESIAN_POINT ( 'NONE',  ( 6.500168698208129925, 211.6636982574063381, 61.70113791807857240 ) ) ;
#20368=EDGE_CURVE ( 'NONE', #24063, #20665, #8918, .T. ) ;
#20370=CARTESIAN_POINT ( 'NONE',  ( 2.426778023690261410, 199.3768101843759837, 77.60113791807854966 ) ) ;
#20374=CARTESIAN_POINT ( 'NONE',  ( 4.903702542908435547, 213.8346818373419751, 60.54886208192144181 ) ) ;
#20376=CARTESIAN_POINT ( 'NONE',  ( -3.135527875058821579, 197.5041725223112223, -0.09886208192143428053 ) ) ;
#20382=CARTESIAN_POINT ( 'NONE',  ( 12.01549611932652972, 210.8513442034534933, 67.85113791807857808 ) ) ;
#20384=CARTESIAN_POINT ( 'NONE',  ( 3.662846001190051659, 195.5725841191953691, 11.60113791807856742 ) ) ;
#20385=CARTESIAN_POINT ( 'NONE',  ( 8.118202686958039038, 212.8392687619912635, 85.70113791807858661 ) ) ;
#20386=CARTESIAN_POINT ( 'NONE',  ( -9.736236675708031640, 214.0148392665760753, 41.79886208192143471 ) ) ;
#20387=CARTESIAN_POINT ( 'NONE',  ( 9.984503880673420539, 210.2968891136705736, 60.84886208192143187 ) ) ;
#20389=CARTESIAN_POINT ( 'NONE',  ( 7.456977232089302632, 217.1783343296989131, 97.55113791807858092 ) ) ;
#20391=CARTESIAN_POINT ( 'NONE',  ( -0.05014649552810635652, 196.4853777576173002, 2.751137918078565114 ) ) ;
#20392=CARTESIAN_POINT ( 'NONE',  ( -6.139770520408224463, 198.4640165459539389, 74.04886208192142760 ) ) ;
#20395=CARTESIAN_POINT ( 'NONE',  ( 11.98450388067341876, 210.9467285061363953, 66.84886208192143897 ) ) ;
#20396=CARTESIAN_POINT ( 'NONE',  ( 0.05014649552810505201, 217.5146222423826714, 91.25113791807858377 ) ) ;
#20399=CARTESIAN_POINT ( 'NONE',  ( -7.984503880673422316, 204.3529502787951628, 53.34886208192144608 ) ) ;
#20404=DIRECTION ( 'NONE',  ( 0.000000000000000000, 0.9988620819214349966, -0.04769215134146094492 ) ) ;
#20408=CARTESIAN_POINT ( 'NONE',  ( -10.00000000000000711, 206.9523078486584495, 56.49886208192143755 ) ) ;
#20413=CARTESIAN_POINT ( 'NONE',  ( 6.444103211790928043, 211.7408657792734061, 21.69886208192144039 ) ) ;
#20415=CARTESIAN_POINT ( 'NONE',  ( 8.062137200540920645, 201.0835637161417822, 68.30113791807856671 ) ) ;
#20417=CARTESIAN_POINT ( 'NONE',  ( -3.044812012440131443, 216.5253028482142952, 55.10113791807857098 ) ) ;
#20418=CARTESIAN_POINT ( 'NONE',  ( -10.00000000000000711, 207.0476921513413515, 24.50113791807856600 ) ) ;
#20419=CARTESIAN_POINT ( 'NONE',  ( 8.000000000000008882, 206.9523078486586485, 2.001137918078566003 ) ) ;
#20423=CARTESIAN_POINT ( 'NONE',  ( -3.662846001190052991, 218.4274158808045740, 25.10113791807856742 ) ) ;
#20425=CARTESIAN_POINT ( 'NONE',  ( -10.00000000000000711, 207.0476921513413515, 84.50113791807856956 ) ) ;
#20426=CARTESIAN_POINT ( 'NONE',  ( 3.044812012440130555, 197.4746971517856764, 50.60113791807857808 ) ) ;
#20428=CARTESIAN_POINT ( 'NONE',  ( -3.753561863808878130, 218.3979405102790281, 9.098862081921435419 ) ) ;
#20429=CARTESIAN_POINT ( 'NONE',  ( -3.135527875058982783, 216.4958274776886924, 30.09886208192143897 ) ) ;
#20432=CARTESIAN_POINT ( 'NONE',  ( 9.736236675707914401, 214.0148392665762458, 58.70113791807857240 ) ) ;
#20433=CARTESIAN_POINT ( 'NONE',  ( 7.984503880673485376, 204.3529502787953902, 83.15113791807856103 ) ) ;
#20434=CARTESIAN_POINT ( 'NONE',  ( -0.05014649552828403384, 217.5146222423826714, 36.24886208192143755 ) ) ;
#20437=CARTESIAN_POINT ( 'NONE',  ( 11.98450388067341876, 210.9467285061363953, 39.84886208192143187 ) ) ;
#20443=CARTESIAN_POINT ( 'NONE',  ( 2.517493886308900919, 214.5937144450984420, 34.40113791807856813 ) ) ;
#20446=CARTESIAN_POINT ( 'NONE',  ( 9.984503880673420539, 210.2968891136705167, 9.848862081921435419 ) ) ;
#20449=CARTESIAN_POINT ( 'NONE',  ( 4.903702542908601636, 200.1653181626581102, 59.45113791807857240 ) ) ;
#20453=CARTESIAN_POINT ( 'NONE',  ( 3.135527875058981895, 197.5041725223112792, 103.5988620819214390 ) ) ;
#20455=CARTESIAN_POINT ( 'NONE',  ( 10.01549611932653860, 210.2015048109876716, 37.85113791807854966 ) ) ;
#20457=CARTESIAN_POINT ( 'NONE',  ( -9.984503880673473830, 210.2968891136704315, 27.65113791807855748 ) ) ;
#20463=CARTESIAN_POINT ( 'NONE',  ( 12.01549611932652972, 210.8513442034534933, 1.851137918078565647 ) ) ;
#20466=CARTESIAN_POINT ( 'NONE',  ( -6.139770520408369237, 215.5359834540460042, 48.95113791807855108 ) ) ;
#20472=CARTESIAN_POINT ( 'NONE',  ( -9.736236675707914401, 199.9851607334237542, 27.20113791807857240 ) ) ;
#20474=CARTESIAN_POINT ( 'NONE',  ( 8.062137200540822946, 212.9164362838583315, 9.698862081921435063 ) ) ;
#20477=CARTESIAN_POINT ( 'NONE',  ( -9.984503880673473830, 210.2968891136704315, 9.651137918078568134 ) ) ;
#20478=CARTESIAN_POINT ( 'NONE',  ( -6.220909254589537696, 198.5229672870051161, 72.05113791807853829 ) ) ;
#20480=CARTESIAN_POINT ( 'NONE',  ( 6.500168698208244500, 202.3363017425938324, 25.29886208192143826 ) ) ;
#20483=CARTESIAN_POINT ( 'NONE',  ( 8.000000000000008882, 206.9523078486586485, 8.001137918078566003 ) ) ;
#20485=CARTESIAN_POINT ( 'NONE',  ( 11.98450388067341876, 210.9467285061363953, 84.84886208192142476 ) ) ;
#20491=CARTESIAN_POINT ( 'NONE',  ( 8.118202686958039038, 212.8392687619912635, 4.701137918078565292 ) ) ;
#20492=CARTESIAN_POINT ( 'NONE',  ( 10.01549611932659545, 203.7984951890123853, 73.14886208192143613 ) ) ;
#20495=CARTESIAN_POINT ( 'NONE',  ( -10.00000000000000711, 207.0476921513413515, 12.50113791807856778 ) ) ;
#20500=CARTESIAN_POINT ( 'NONE',  ( -10.00000000000000711, 207.0476921513413515, 102.5011379180785838 ) ) ;
#20502=CARTESIAN_POINT ( 'NONE',  ( -8.062137200540920645, 212.9164362838581894, 78.80113791807858092 ) ) ;
#20505=CARTESIAN_POINT ( 'NONE',  ( 11.98450388067341876, 210.9467285061363953, 84.84886208192142476 ) ) ;
#20510=CARTESIAN_POINT ( 'NONE',  ( 12.00000000000000711, 206.9523078486586485, 92.00113791807858377 ) ) ;
#20515=CARTESIAN_POINT ( 'NONE',  ( 0.05014649552828275014, 196.4853777576173002, 85.74886208192141623 ) ) ;
#20516=CARTESIAN_POINT ( 'NONE',  ( -7.456977232089471386, 217.1783343296987709, 26.94886208192142973 ) ) ;
#20518=CARTESIAN_POINT ( 'NONE',  ( 6.220909254589536808, 215.4770327129947702, 43.55113791807857382 ) ) ;
#20520=CARTESIAN_POINT ( 'NONE',  ( -9.984503880673420539, 203.7031108863293980, 101.3488620819213963 ) ) ;
#20523=CARTESIAN_POINT ( 'NONE',  ( -4.984841277089891776, 213.7757310962905990, 80.94886208192143329 ) ) ;
#20528=CARTESIAN_POINT ( 'NONE',  ( -2.517493886308901807, 199.4062855549015012, 62.90113791807858945 ) ) ;
#20531=CARTESIAN_POINT ( 'NONE',  ( -2.517493886308901807, 199.4062855549015012, 83.90113791807856103 ) ) ;
#20536=CARTESIAN_POINT ( 'NONE',  ( -7.984503880673422316, 204.3529502787951628, 59.34886208192144608 ) ) ;
#20540=CARTESIAN_POINT ( 'NONE',  ( 0.05014649552810506589, 217.5146222423826714, 1.251137918078566003 ) ) ;
#20545=CARTESIAN_POINT ( 'NONE',  ( 12.00000000000000711, 206.9523078486586485, 65.00113791807856956 ) ) ;
#20547=CARTESIAN_POINT ( 'NONE',  ( 11.98450388067348271, 203.0532714938637753, 11.15113791807856636 ) ) ;
#20548=CARTESIAN_POINT ( 'NONE',  ( -9.984503880673475606, 210.2968891136704315, 84.65113791807857524 ) ) ;
#20549=CARTESIAN_POINT ( 'NONE',  ( 9.736236675708031640, 199.9851607334238963, 49.29886208192143471 ) ) ;
#20550=CARTESIAN_POINT ( 'NONE',  ( 8.118202686958138514, 201.1607312380088501, 55.29886208192144181 ) ) ;
#20552=CARTESIAN_POINT ( 'NONE',  ( -7.456977232089304408, 196.8216656703010301, 99.05113791807858092 ) ) ;
#20555=CARTESIAN_POINT ( 'NONE',  ( 6.220909254589536808, 215.4770327129947702, 4.551137918078564937 ) ) ;
#20556=CARTESIAN_POINT ( 'NONE',  ( -6.139770520408224463, 198.4640165459539389, 65.04886208192144181 ) ) ;
#20560=CARTESIAN_POINT ( 'NONE',  ( 12.01549611932659367, 203.1486557965466773, 79.14886208192143613 ) ) ;
#20562=CARTESIAN_POINT ( 'NONE',  ( -10.01549611932653860, 203.7984951890123284, 93.35113791807857808 ) ) ;
#20565=CARTESIAN_POINT ( 'NONE',  ( -6.444103211790928043, 202.2591342207265939, 53.19886208192144039 ) ) ;
#20575=CARTESIAN_POINT ( 'NONE',  ( -9.984503880673420539, 203.7031108863293980, 50.34886208192141765 ) ) ;
#20580=CARTESIAN_POINT ( 'NONE',  ( -4.984841277089891776, 213.7757310962905990, 38.94886208192144039 ) ) ;
#20582=CARTESIAN_POINT ( 'NONE',  ( -6.139770520408369237, 215.5359834540460042, 69.95113791807857240 ) ) ;
#20584=CARTESIAN_POINT ( 'NONE',  ( -8.062137200540920645, 212.9164362838581894, 57.80113791807857382 ) ) ;
#20588=CARTESIAN_POINT ( 'NONE',  ( 8.118202686958039038, 212.8392687619912635, 28.70113791807856884 ) ) ;
#20589=CARTESIAN_POINT ( 'NONE',  ( 4.984841277089725686, 213.7757310962907411, 19.55113791807856671 ) ) ;
#20591=CARTESIAN_POINT ( 'NONE',  ( 10.00000000000000888, 207.9248754155063637, 0.9569796661747027589 ) ) ;
#20593=CARTESIAN_POINT ( 'NONE',  ( 7.375838497908181246, 196.7627149292499666, 41.45113791807857240 ) ) ;
#20595=CARTESIAN_POINT ( 'NONE',  ( 8.118202686958039038, 212.8392687619912635, 88.70113791807857240 ) ) ;
#20596=CARTESIAN_POINT ( 'NONE',  ( -8.118202686958039038, 201.1607312380087080, 63.20113791807857240 ) ) ;
#20598=CARTESIAN_POINT ( 'NONE',  ( -3.662846001189865142, 195.5725841191952838, 19.89886208192143613 ) ) ;
#20599=CARTESIAN_POINT ( 'NONE',  ( 3.044812012439969795, 216.5253028482143520, 30.39886208192143613 ) ) ;
#20602=CARTESIAN_POINT ( 'NONE',  ( 3.753561863808689836, 218.3979405102790565, 70.40113791807856103 ) ) ;
#20603=CARTESIAN_POINT ( 'NONE',  ( -6.444103211791042618, 211.7408657792732356, 78.80113791807858092 ) ) ;
#20605=CARTESIAN_POINT ( 'NONE',  ( 10.01549611932659545, 203.7984951890123853, 43.14886208192142192 ) ) ;
#20608=CARTESIAN_POINT ( 'NONE',  ( 0.05014649552828288198, 194.3824533091408000, 49.74886208192143044 ) ) ;
#20618=CARTESIAN_POINT ( 'NONE',  ( 4.903702542908601636, 200.1653181626581102, 44.45113791807857240 ) ) ;
#20619=CARTESIAN_POINT ( 'NONE',  ( 10.01549611932659545, 203.7984951890123853, 25.14886208192143613 ) ) ;
#20624=CARTESIAN_POINT ( 'NONE',  ( -6.444103211790928043, 202.2591342207265939, 8.198862081921436840 ) ) ;
#20625=CARTESIAN_POINT ( 'NONE',  ( 10.00000000000000711, 206.9523078486586201, 41.00113791807856956 ) ) ;
#20626=CARTESIAN_POINT ( 'NONE',  ( 10.00000000000000711, 206.9523078486586201, 29.00113791807856956 ) ) ;
#20627=CARTESIAN_POINT ( 'NONE',  ( 6.139770520408223575, 215.5359834540460611, 102.5488620819214134 ) ) ;
#20630=CARTESIAN_POINT ( 'NONE',  ( 2.517493886309087436, 199.4062855549015865, 79.59886208192143897 ) ) ;
#20633=CARTESIAN_POINT ( 'NONE',  ( 12.01549611932652972, 210.8513442034534933, 7.851137918078565647 ) ) ;
#20637=EDGE_CURVE ( 'NONE', #19921, #13301, #22277, .T. ) ;
#20638=CARTESIAN_POINT ( 'NONE',  ( -8.062137200540920645, 212.9164362838581894, 60.80113791807857382 ) ) ;
#20639=EDGE_CURVE ( 'NONE', #25814, #9574, #8092, .T. ) ;
#20643=CARTESIAN_POINT ( 'NONE',  ( -8.062137200540822946, 201.0835637161416400, 2.198862081921434175 ) ) ;
#20646=CARTESIAN_POINT ( 'NONE',  ( -12.01549611932652972, 203.1486557965464499, 36.35113791807856387 ) ) ;
#20651=CARTESIAN_POINT ( 'NONE',  ( 6.220909254589681581, 198.5229672870052582, 16.44886208192143329 ) ) ;
#20654=CARTESIAN_POINT ( 'NONE',  ( 10.01549611932653860, 210.2015048109876716, 10.85113791807856387 ) ) ;
#20655=CARTESIAN_POINT ( 'NONE',  ( 3.044812012440130555, 197.4746971517856764, 68.60113791807857808 ) ) ;
#20657=CARTESIAN_POINT ( 'NONE',  ( 0.05014649552828262524, 198.5883022060938572, 28.74886208192144110 ) ) ;
#20661=CARTESIAN_POINT ( 'NONE',  ( -6.444103211791042618, 211.7408657792732356, 15.80113791807856849 ) ) ;
#20663=CARTESIAN_POINT ( 'NONE',  ( 7.375838497908012492, 217.2372850707501186, 96.54886208192142760 ) ) ;
#20665=VERTEX_POINT ( 'NONE', #6605 ) ;
#20668=CARTESIAN_POINT ( 'NONE',  ( -10.00000000000000711, 207.0476921513413515, 6.501137918078566003 ) ) ;
#20669=CARTESIAN_POINT ( 'NONE',  ( 9.984503880673420539, 210.2968891136705167, 75.84886208192143897 ) ) ;
#20672=CARTESIAN_POINT ( 'NONE',  ( 3.135527875058820690, 216.4958274776887492, 13.40113791807856636 ) ) ;
#20674=CARTESIAN_POINT ( 'NONE',  ( -3.044812012440131443, 216.5253028482142952, 97.10113791807857808 ) ) ;
#20676=CARTESIAN_POINT ( 'NONE',  ( -9.984503880673473830, 210.2968891136704315, 81.65113791807857524 ) ) ;
#20679=CARTESIAN_POINT ( 'NONE',  ( 9.736236675708031640, 199.9851607334238963, 100.2988620819214276 ) ) ;
#20684=CARTESIAN_POINT ( 'NONE',  ( 12.01549611932652972, 210.8513442034534933, 91.85113791807857808 ) ) ;
#20685=CARTESIAN_POINT ( 'NONE',  ( -10.37719565735124938, 206.0286316962952640, 104.3663993655802784 ) ) ;
#20687=CARTESIAN_POINT ( 'NONE',  ( -3.044812012439970683, 197.4746971517856196, 88.89886208192143613 ) ) ;
#20688=CARTESIAN_POINT ( 'NONE',  ( -12.00000000000000711, 206.9523078486584780, 20.49886208192143755 ) ) ;
#20690=CARTESIAN_POINT ( 'NONE',  ( -8.118202686958039038, 201.1607312380087080, 45.20113791807857240 ) ) ;
#20692=CARTESIAN_POINT ( 'NONE',  ( -4.903702542908436435, 200.1653181626580249, 2.048862081921434708 ) ) ;
#20695=CARTESIAN_POINT ( 'NONE',  ( -4.903702542908436435, 200.1653181626580249, 83.04886208192144181 ) ) ;
#20698=ORIENTED_EDGE ( 'NONE', *, *, #23335, .F. ) ;
#20702=CARTESIAN_POINT ( 'NONE',  ( 6.500168698208129925, 211.6636982574063381, 85.70113791807858661 ) ) ;
#20705=CARTESIAN_POINT ( 'NONE',  ( -2.426778023690076225, 199.3768101843759553, 58.89886208192144323 ) ) ;
#20708=CARTESIAN_POINT ( 'NONE',  ( 10.00000000000000711, 206.9523078486586201, 2.001137918078565558 ) ) ;
#20713=CARTESIAN_POINT ( 'NONE',  ( -9.680171189290831535, 214.0920067884431148, 69.80113791807856671 ) ) ;
#20715=CARTESIAN_POINT ( 'NONE',  ( -0.05014649552807705357, 194.3824533091408000, 14.75113791807856600 ) ) ;
#20716=CARTESIAN_POINT ( 'NONE',  ( 3.044812012440130555, 197.4746971517856764, 86.60113791807857808 ) ) ;
#20717=CARTESIAN_POINT ( 'NONE',  ( -9.736236675708031640, 214.0148392665760753, 53.79886208192143471 ) ) ;
#20718=CARTESIAN_POINT ( 'NONE',  ( -8.062137200540822946, 201.0835637161416400, 59.19886208192144039 ) ) ;
#20720=CARTESIAN_POINT ( 'NONE',  ( -7.375838497908182134, 217.2372850707499765, 99.95113791807860082 ) ) ;
#20722=CARTESIAN_POINT ( 'NONE',  ( 6.220909254589536808, 215.4770327129947702, 16.55113791807857027 ) ) ;
#20723=CARTESIAN_POINT ( 'NONE',  ( -10.01549611932659722, 210.2015048109875011, 83.64886208192143613 ) ) ;
#20727=CARTESIAN_POINT ( 'NONE',  ( 11.98450388067341876, 210.9467285061363953, 78.84886208192143897 ) ) ;
#20731=CARTESIAN_POINT ( 'NONE',  ( 6.444103211790928043, 211.7408657792734061, 51.69886208192144039 ) ) ;
#20739=CARTESIAN_POINT ( 'NONE',  ( 10.01549611932659545, 203.7984951890123853, 55.14886208192143613 ) ) ;
#20743=CARTESIAN_POINT ( 'NONE',  ( -2.517493886309087880, 214.5937144450984135, 36.09886208192144608 ) ) ;
#20744=CARTESIAN_POINT ( 'NONE',  ( -10.00000000000000711, 207.0476921513413515, 69.50113791807856956 ) ) ;
#20746=CARTESIAN_POINT ( 'NONE',  ( -10.01549611932653860, 203.7984951890123284, 57.35113791807856387 ) ) ;
#20747=CARTESIAN_POINT ( 'NONE',  ( -3.044812012440131443, 216.5253028482142952, 31.10113791807856742 ) ) ;
#20748=CARTESIAN_POINT ( 'NONE',  ( -4.984841277089726574, 200.2242689037092305, 12.05113791807856849 ) ) ;
#20752=CARTESIAN_POINT ( 'NONE',  ( 12.01549611932652972, 210.8513442034534933, 40.85113791807856387 ) ) ;
#20754=CARTESIAN_POINT ( 'NONE',  ( 10.01549611932653860, 210.2015048109876716, 82.85113791807854966 ) ) ;
#20755=CARTESIAN_POINT ( 'NONE',  ( -10.01549611932653860, 203.7984951890123000, 54.35113791807856387 ) ) ;
#20757=CARTESIAN_POINT ( 'NONE',  ( -12.00000000000000711, 206.9523078486584780, 23.49886208192144110 ) ) ;
#20758=CARTESIAN_POINT ( 'NONE',  ( 6.220909254589680693, 198.5229672870052582, 28.44886208192143684 ) ) ;
#20761=CARTESIAN_POINT ( 'NONE',  ( -12.01549611932652972, 203.1486557965464499, 72.35113791807857808 ) ) ;
#20762=CARTESIAN_POINT ( 'NONE',  ( 8.000000000000008882, 206.9523078486586485, 86.00113791807856956 ) ) ;
#20763=CARTESIAN_POINT ( 'NONE',  ( -10.00000000000000711, 206.9523078486584495, 44.49886208192143755 ) ) ;
#20767=CARTESIAN_POINT ( 'NONE',  ( -3.753561863808878130, 218.3979405102790281, 48.09886208192143897 ) ) ;
#20774=CARTESIAN_POINT ( 'NONE',  ( -0.05014649552807731031, 198.5883022060938572, 41.75113791807856956 ) ) ;
#20776=CARTESIAN_POINT ( 'NONE',  ( 9.984503880673420539, 210.2968891136705167, 18.84886208192143542 ) ) ;
#20781=CARTESIAN_POINT ( 'NONE',  ( 4.984841277089891776, 200.2242689037093726, 4.448862081921435063 ) ) ;
#20783=CARTESIAN_POINT ( 'NONE',  ( 6.139770520408368348, 198.4640165459539674, 44.45113791807855819 ) ) ;
#20786=CARTESIAN_POINT ( 'NONE',  ( -6.139770520408369237, 215.5359834540460042, 27.95113791807856174 ) ) ;
#20787=CARTESIAN_POINT ( 'NONE',  ( -8.062137200540822946, 201.0835637161416400, 104.1988620819214475 ) ) ;
#20788=CARTESIAN_POINT ( 'NONE',  ( 7.984503880673422316, 209.6470497212048372, 96.84886208192143897 ) ) ;
#20793=CARTESIAN_POINT ( 'NONE',  ( -7.375838497908182134, 217.2372850707499765, 12.95113791807856707 ) ) ;
#20797=CARTESIAN_POINT ( 'NONE',  ( -3.044812012440131443, 216.5253028482142952, 52.10113791807857808 ) ) ;
#20803=CARTESIAN_POINT ( 'NONE',  ( 9.680171189290831535, 199.9079932115568852, 35.30113791807856671 ) ) ;
#20805=CARTESIAN_POINT ( 'NONE',  ( -9.984503880673420539, 203.7031108863293980, 8.348862081921435419 ) ) ;
#20809=CARTESIAN_POINT ( 'NONE',  ( -8.118202686958039038, 201.1607312380087080, 9.201137918078565292 ) ) ;
#20810=CARTESIAN_POINT ( 'NONE',  ( -9.984503880673473830, 210.2968891136704315, 69.65113791807854682 ) ) ;
#20812=CARTESIAN_POINT ( 'NONE',  ( -6.500168698208244500, 211.6636982574061676, 32.79886208192143471 ) ) ;
#20816=CARTESIAN_POINT ( 'NONE',  ( 6.500168698208129925, 211.6636982574063381, 16.70113791807856529 ) ) ;
#20819=CARTESIAN_POINT ( 'NONE',  ( -7.456977232089471386, 217.1783343296987709, 98.94886208192143329 ) ) ;
#20824=CARTESIAN_POINT ( 'NONE',  ( 6.220909254589536808, 215.4770327129947702, 7.551137918078564049 ) ) ;
#20825=CARTESIAN_POINT ( 'NONE',  ( -9.984503880673420539, 203.7031108863293980, 80.34886208192143897 ) ) ;
#20828=CARTESIAN_POINT ( 'NONE',  ( 0.05014649552810505201, 217.5146222423826714, 13.25113791807856778 ) ) ;
#20833=CARTESIAN_POINT ( 'NONE',  ( -9.898309971686792608, 228.3698647632124334, 103.4854814124440452 ) ) ;
#20835=CARTESIAN_POINT ( 'NONE',  ( 6.139770520408368348, 198.4640165459539674, 86.45113791807854398 ) ) ;
#20839=CARTESIAN_POINT ( 'NONE',  ( -12.01549611932659722, 210.8513442034533227, 95.64886208192143613 ) ) ;
#20845=CARTESIAN_POINT ( 'NONE',  ( 9.736236675707914401, 214.0148392665762458, 97.70113791807858661 ) ) ;
#20847=VECTOR ( 'NONE', #4166, 1000.000000000000227 ) ;
#20851=CARTESIAN_POINT ( 'NONE',  ( -6.220909254589682469, 215.4770327129947134, 83.94886208192144750 ) ) ;
#20852=CARTESIAN_POINT ( 'NONE',  ( -7.456977232089471386, 217.1783343296987709, 23.94886208192143684 ) ) ;
#20854=CARTESIAN_POINT ( 'NONE',  ( -9.984503880673473830, 210.2968891136704315, 45.65113791807855392 ) ) ;
#20857=CARTESIAN_POINT ( 'NONE',  ( 0.05014649552828262524, 198.5883022060938572, 4.748862081921434886 ) ) ;
#20861=CARTESIAN_POINT ( 'NONE',  ( -8.015496119326597224, 209.5516654185217362, 86.64886208192143613 ) ) ;
#20864=CARTESIAN_POINT ( 'NONE',  ( 8.000000000000008882, 206.9523078486586485, 29.00113791807856956 ) ) ;
#20872=CARTESIAN_POINT ( 'NONE',  ( -0.05014649552807731031, 198.5883022060938572, 86.75113791807856956 ) ) ;
#20877=CARTESIAN_POINT ( 'NONE',  ( -2.426778023690076225, 199.3768101843759553, 61.89886208192143613 ) ) ;
#20881=CARTESIAN_POINT ( 'NONE',  ( -8.118202686958039038, 201.1607312380087080, 3.201137918078566180 ) ) ;
#20885=CARTESIAN_POINT ( 'NONE',  ( -7.375838497908182134, 217.2372850707499765, 69.95113791807858661 ) ) ;
#20887=CARTESIAN_POINT ( 'NONE',  ( -3.662846001190052991, 218.4274158808045740, 13.10113791807856742 ) ) ;
#20888=CARTESIAN_POINT ( 'NONE',  ( -3.044812012440131443, 216.5253028482142952, 85.10113791807857808 ) ) ;
#20890=CARTESIAN_POINT ( 'NONE',  ( -3.753561863808878130, 218.3979405102790281, 54.09886208192143897 ) ) ;
#20891=CARTESIAN_POINT ( 'NONE',  ( 6.220909254589680693, 198.5229672870052582, 61.44886208192142618 ) ) ;
#20893=CARTESIAN_POINT ( 'NONE',  ( 12.01549611932652972, 210.8513442034534933, 100.8511379180785781 ) ) ;
#20895=CARTESIAN_POINT ( 'NONE',  ( -8.062137200540920645, 212.9164362838581894, 9.801137918078566713 ) ) ;
#20897=CARTESIAN_POINT ( 'NONE',  ( 8.118202686958138514, 201.1607312380088501, 79.29886208192144181 ) ) ;
#20899=CARTESIAN_POINT ( 'NONE',  ( 3.753561863808876797, 195.6020594897209719, 76.59886208192142476 ) ) ;
#20903=CARTESIAN_POINT ( 'NONE',  ( -8.000000000000008882, 206.9523078486584780, 65.49886208192144466 ) ) ;
#20911=CARTESIAN_POINT ( 'NONE',  ( -0.05014649552828403384, 217.5146222423826714, 54.24886208192142334 ) ) ;
#20916=CARTESIAN_POINT ( 'NONE',  ( 0.05014649552828262524, 198.5883022060938572, 34.74886208192143755 ) ) ;
#20918=CARTESIAN_POINT ( 'NONE',  ( -10.00000000000000711, 207.0476921513413515, 72.50113791807858377 ) ) ;
#20921=CARTESIAN_POINT ( 'NONE',  ( -6.139770520408369237, 215.5359834540460042, 60.95113791807857950 ) ) ;
#20922=CARTESIAN_POINT ( 'NONE',  ( 9.984503880673470277, 203.7031108863295401, 26.15113791807856813 ) ) ;
#20923=CARTESIAN_POINT ( 'NONE',  ( -7.984503880673488041, 209.6470497212046098, 18.65113791807856458 ) ) ;
#20927=CARTESIAN_POINT ( 'NONE',  ( -3.753561863808691168, 195.6020594897209435, 41.90113791807856813 ) ) ;
#20929=CARTESIAN_POINT ( 'NONE',  ( -3.044812012440131443, 216.5253028482142952, 82.10113791807857808 ) ) ;
#20930=CARTESIAN_POINT ( 'NONE',  ( 3.135527875058820690, 216.4958274776887492, 55.40113791807857524 ) ) ;
#20932=CARTESIAN_POINT ( 'NONE',  ( 11.98450388067341876, 210.9467285061363953, 21.84886208192143542 ) ) ;
#20933=CARTESIAN_POINT ( 'NONE',  ( -0.05014649552828402690, 217.5146222423826714, 33.24886208192141623 ) ) ;
#20935=CARTESIAN_POINT ( 'NONE',  ( -12.00000000000000711, 207.0476921513413515, 63.50113791807856956 ) ) ;
#20936=CARTESIAN_POINT ( 'NONE',  ( -4.984841277089726574, 200.2242689037092305, 84.05113791807858092 ) ) ;
#20937=CARTESIAN_POINT ( 'NONE',  ( 10.00000000000000711, 207.0476921513415220, 51.99886208192143755 ) ) ;
#20940=CARTESIAN_POINT ( 'NONE',  ( 0.05014649552828288198, 194.3824533091408000, 55.74886208192143755 ) ) ;
#20945=CARTESIAN_POINT ( 'NONE',  ( 2.517493886308900919, 214.5937144450984420, 37.40113791807856813 ) ) ;
#20947=CARTESIAN_POINT ( 'NONE',  ( 10.00000000000000711, 207.0476921513415220, 18.99886208192143755 ) ) ;
#20953=CARTESIAN_POINT ( 'NONE',  ( 6.444103211790928043, 211.7408657792734061, 6.698862081921435063 ) ) ;
#20954=CARTESIAN_POINT ( 'NONE',  ( 3.044812012440130555, 197.4746971517856764, 38.60113791807857098 ) ) ;
#20957=CARTESIAN_POINT ( 'NONE',  ( -8.062137200540920645, 212.9164362838581894, 24.80113791807857027 ) ) ;
#20958=CARTESIAN_POINT ( 'NONE',  ( -9.984503880673420539, 203.7031108863293980, 101.3488620819214248 ) ) ;
#20960=CARTESIAN_POINT ( 'NONE',  ( -2.426778023690076225, 199.3768101843759553, 91.89886208192143613 ) ) ;
#20963=CARTESIAN_POINT ( 'NONE',  ( 9.736236675707914401, 214.0148392665762458, 10.70113791807856529 ) ) ;
#20966=CARTESIAN_POINT ( 'NONE',  ( -10.01549611932653860, 203.7984951890123284, 57.35113791807856387 ) ) ;
#20967=CARTESIAN_POINT ( 'NONE',  ( -9.984503880673475606, 210.2968891136704315, 30.65113791807856813 ) ) ;
#20969=ADVANCED_FACE ( 'NONE', ( #7296 ), #10684, .T. ) ;
#20971=CARTESIAN_POINT ( 'NONE',  ( -10.01549611932659545, 210.2015048109875011, 2.648862081921434353 ) ) ;
#20974=CARTESIAN_POINT ( 'NONE',  ( -12.01549611932652972, 203.1486557965464499, 42.35113791807857098 ) ) ;
#20976=CARTESIAN_POINT ( 'NONE',  ( -3.044812012439970683, 197.4746971517856196, 22.89886208192143613 ) ) ;
#20979=CARTESIAN_POINT ( 'NONE',  ( 8.118202686958039038, 212.8392687619912635, 70.70113791807857240 ) ) ;
#20984=CARTESIAN_POINT ( 'NONE',  ( -6.500168698208129925, 202.3363017425936050, 15.20113791807857062 ) ) ;
#20986=CARTESIAN_POINT ( 'NONE',  ( -7.375838497908014268, 196.7627149292498530, 95.04886208192144181 ) ) ;
#20991=CARTESIAN_POINT ( 'NONE',  ( -8.062137200540920645, 212.9164362838581894, 12.80113791807856671 ) ) ;
#20992=CARTESIAN_POINT ( 'NONE',  ( 9.984503880673420539, 210.2968891136705167, 78.84886208192139634 ) ) ;
#20995=CARTESIAN_POINT ( 'NONE',  ( 10.01549611932653860, 210.2015048109876716, 10.85113791807856387 ) ) ;
#20999=CARTESIAN_POINT ( 'NONE',  ( 3.044812012440130555, 197.4746971517856764, 98.60113791807857808 ) ) ;
#21001=CARTESIAN_POINT ( 'NONE',  ( 8.118202686958039038, 212.8392687619912635, 82.70113791807857240 ) ) ;
#21004=CARTESIAN_POINT ( 'NONE',  ( -12.00000000000000711, 206.9523078486584780, 92.49886208192144466 ) ) ;
#21009=ADVANCED_BREP_SHAPE_REPRESENTATION ( '', ( #1296, #2404 ), #11135 ) ;
#21010=CARTESIAN_POINT ( 'NONE',  ( -11.98450388067348804, 210.9467285061362247, 96.65113791807858945 ) ) ;
#21014=CARTESIAN_POINT ( 'NONE',  ( -3.135527875058982783, 216.4958274776886924, 99.09886208192143897 ) ) ;
#21015=CARTESIAN_POINT ( 'NONE',  ( -9.680171189290716072, 199.9079932115567146, 26.19886208192144039 ) ) ;
#21016=CARTESIAN_POINT ( 'NONE',  ( 8.118202686958039038, 212.8392687619912635, 46.70113791807857240 ) ) ;
#21019=CARTESIAN_POINT ( 'NONE',  ( -6.500168698208244500, 211.6636982574061676, 8.798862081921434708 ) ) ;
#21023=CARTESIAN_POINT ( 'NONE',  ( 4.903702542908435547, 213.8346818373419751, 93.54886208192142760 ) ) ;
#21024=CARTESIAN_POINT ( 'NONE',  ( -6.444103211791042618, 211.7408657792732356, 30.80113791807857027 ) ) ;
#21031=CARTESIAN_POINT ( 'NONE',  ( 2.426778023690261410, 199.3768101843759837, 92.60113791807857808 ) ) ;
#21034=CARTESIAN_POINT ( 'NONE',  ( 8.000000000000008882, 207.0476921513415220, 66.99886208192144466 ) ) ;
#21039=CARTESIAN_POINT ( 'NONE',  ( -6.139770520408368348, 215.5359834540460042, 0.9511379180785657361 ) ) ;
#21043=CARTESIAN_POINT ( 'NONE',  ( -12.01549611932652972, 203.1486557965464499, 63.35113791807857098 ) ) ;
#21047=CARTESIAN_POINT ( 'NONE',  ( -8.062137200540920645, 212.9164362838581894, 90.80113791807858092 ) ) ;
#21050=CARTESIAN_POINT ( 'NONE',  ( -12.00000000000000711, 206.9523078486584780, 50.49886208192143044 ) ) ;
#21051=CARTESIAN_POINT ( 'NONE',  ( 0.05014649552828275014, 196.4853777576173002, 55.74886208192143755 ) ) ;
#21052=CARTESIAN_POINT ( 'NONE',  ( -9.736236675707914401, 199.9851607334237542, 96.20113791807858661 ) ) ;
#21054=CARTESIAN_POINT ( 'NONE',  ( -0.05014649552810635652, 196.4853777576173002, 14.75113791807856245 ) ) ;
#21058=CARTESIAN_POINT ( 'NONE',  ( -3.135527875058982783, 216.4958274776886924, 75.09886208192143897 ) ) ;
#21060=CARTESIAN_POINT ( 'NONE',  ( 6.139770520408368348, 198.4640165459539674, 95.45113791807855819 ) ) ;
#21062=CARTESIAN_POINT ( 'NONE',  ( -6.444103211790928043, 202.2591342207265939, 65.19886208192143329 ) ) ;
#21069=CARTESIAN_POINT ( 'NONE',  ( -0.05014649552807731031, 198.5883022060938572, 56.75113791807857666 ) ) ;
#21070=CARTESIAN_POINT ( 'NONE',  ( 6.220909254589681581, 198.5229672870052582, 55.44886208192141908 ) ) ;
#21074=CARTESIAN_POINT ( 'NONE',  ( -8.000000000000008882, 206.9523078486584780, 32.49886208192143044 ) ) ;
#21075=CARTESIAN_POINT ( 'NONE',  ( 6.139770520408368348, 198.4640165459539674, 83.45113791807858661 ) ) ;
#21077=CARTESIAN_POINT ( 'NONE',  ( 9.984503880673470277, 203.7031108863295401, 59.15113791807858235 ) ) ;
#21078=CARTESIAN_POINT ( 'NONE',  ( 10.00000000000000711, 206.9523078486586201, 29.00113791807856956 ) ) ;
#21079=CARTESIAN_POINT ( 'NONE',  ( -8.000000000000008882, 207.0476921513413515, 15.50113791807856600 ) ) ;
#21083=CARTESIAN_POINT ( 'NONE',  ( 3.753561863808689836, 218.3979405102790565, 34.40113791807856813 ) ) ;
#21086=CARTESIAN_POINT ( 'NONE',  ( 3.135527875058820690, 216.4958274776887492, 88.40113791807857524 ) ) ;
#21087=CARTESIAN_POINT ( 'NONE',  ( -9.984503880673475606, 210.2968891136704315, 60.65113791807856813 ) ) ;
#21089=STYLED_ITEM ( 'NONE', ( #16288 ), #1296 ) ;
#21090=CARTESIAN_POINT ( 'NONE',  ( -9.680171189290716072, 199.9079932115567146, 26.19886208192144039 ) ) ;
#21091=CARTESIAN_POINT ( 'NONE',  ( -8.062137200540822946, 201.0835637161416400, 26.19886208192143684 ) ) ;
#21093=CARTESIAN_POINT ( 'NONE',  ( 11.98450388067348271, 203.0532714938637753, 65.15113791807856103 ) ) ;
#21094=CARTESIAN_POINT ( 'NONE',  ( -0.05014649552807731031, 198.5883022060938572, 92.75113791807858377 ) ) ;
#21096=CARTESIAN_POINT ( 'NONE',  ( 3.135527875058981895, 197.5041725223112792, 49.59886208192143897 ) ) ;
#21100=CARTESIAN_POINT ( 'NONE',  ( -9.680171189290716072, 199.9079932115567146, 53.19886208192144039 ) ) ;
#21102=ORIENTED_EDGE ( 'NONE', *, *, #4602, .F. ) ;
#21105=CARTESIAN_POINT ( 'NONE',  ( -8.000000000000008882, 207.0476921513413515, 42.50113791807857666 ) ) ;
#21109=CARTESIAN_POINT ( 'NONE',  ( 9.984503880673420539, 210.2968891136705167, 24.84886208192143897 ) ) ;
#21115=CARTESIAN_POINT ( 'NONE',  ( -0.05014649552828365914, 215.4116977939061144, 3.248862081921435330 ) ) ;
#21116=CARTESIAN_POINT ( 'NONE',  ( 8.118202686958039038, 212.8392687619912635, 49.70113791807857240 ) ) ;
#21118=CARTESIAN_POINT ( 'NONE',  ( -10.01549611932653860, 203.7984951890123284, 27.35113791807856742 ) ) ;
#21122=CARTESIAN_POINT ( 'NONE',  ( 4.903702542908435547, 213.8346818373419751, 93.54886208192142760 ) ) ;
#21125=CARTESIAN_POINT ( 'NONE',  ( -7.375838497908182134, 217.2372850707499765, 6.951137918078566180 ) ) ;
#21128=CARTESIAN_POINT ( 'NONE',  ( 3.044812012440130555, 197.4746971517856764, 59.60113791807857808 ) ) ;
#21129=CARTESIAN_POINT ( 'NONE',  ( -10.01549611932653860, 203.7984951890123000, 33.35113791807857098 ) ) ;
#21133=EDGE_LOOP ( 'NONE', ( #33607, #12985, #18662, #29898, #4557, #5919, #3710, #7370 ) ) ;
#21134=CARTESIAN_POINT ( 'NONE',  ( 7.456977232089302632, 217.1783343296989131, 34.55113791807856671 ) ) ;
#21136=CARTESIAN_POINT ( 'NONE',  ( -8.118202686958138514, 212.8392687619910930, 23.79886208192143471 ) ) ;
#21138=ORIENTED_EDGE ( 'NONE', *, *, #8713, .T. ) ;
#21140=CARTESIAN_POINT ( 'NONE',  ( -3.135527875058821579, 197.5041725223112223, 68.90113791807857524 ) ) ;
#21147=CARTESIAN_POINT ( 'NONE',  ( 7.984503880673485376, 204.3529502787953902, 11.15113791807856636 ) ) ;
#21148=CARTESIAN_POINT ( 'NONE',  ( 12.00000000000000711, 207.0476921513415220, 96.99886208192143044 ) ) ;
#21153=CARTESIAN_POINT ( 'NONE',  ( 8.118202686958039038, 212.8392687619912635, 10.70113791807856529 ) ) ;
#21155=CARTESIAN_POINT ( 'NONE',  ( -10.00000000000000711, 206.9523078486584495, 80.49886208192143044 ) ) ;
#21158=CARTESIAN_POINT ( 'NONE',  ( 10.00000000000000711, 206.9523078486586201, 23.00113791807856600 ) ) ;
#21161=CARTESIAN_POINT ( 'NONE',  ( 10.01549611932653860, 210.2015048109876716, 97.85113791807857808 ) ) ;
#21163=CARTESIAN_POINT ( 'NONE',  ( 6.139770520408368348, 198.4640165459539674, 89.45113791807857240 ) ) ;
#21166=CARTESIAN_POINT ( 'NONE',  ( -3.753561863808878130, 218.3979405102790281, 96.09886208192143897 ) ) ;
#21177=CARTESIAN_POINT ( 'NONE',  ( -8.118202686958138514, 212.8392687619910930, 95.79886208192144181 ) ) ;
#21178=CARTESIAN_POINT ( 'NONE',  ( 7.456977232089471386, 196.8216656703012006, 28.44886208192142973 ) ) ;
#21181=CARTESIAN_POINT ( 'NONE',  ( -6.220909254589537696, 198.5229672870051161, 42.05113791807857382 ) ) ;
#21183=CARTESIAN_POINT ( 'NONE',  ( -2.426778023690076225, 199.3768101843759553, 4.898862081921435241 ) ) ;
#21187=CARTESIAN_POINT ( 'NONE',  ( -6.444103211790928043, 202.2591342207265939, 89.19886208192144750 ) ) ;
#21188=CARTESIAN_POINT ( 'NONE',  ( -7.984503880673488041, 209.6470497212046098, 30.65113791807856458 ) ) ;
#21196=CARTESIAN_POINT ( 'NONE',  ( -2.517493886308901807, 199.4062855549015012, 89.90113791807857524 ) ) ;
#21199=CARTESIAN_POINT ( 'NONE',  ( -6.500168698208244500, 211.6636982574061676, 77.79886208192142760 ) ) ;
#21204=CARTESIAN_POINT ( 'NONE',  ( -6.139770520408368348, 215.5359834540460042, 6.951137918078566180 ) ) ;
#21209=CARTESIAN_POINT ( 'NONE',  ( -9.680171189290831535, 214.0920067884431148, 81.80113791807858092 ) ) ;
#21212=CARTESIAN_POINT ( 'NONE',  ( 10.00000000000000711, 206.9523078486586201, 98.00113791807856956 ) ) ;
#21215=CARTESIAN_POINT ( 'NONE',  ( 3.753561863808876797, 195.6020594897209719, 52.59886208192143897 ) ) ;
#21216=CARTESIAN_POINT ( 'NONE',  ( -10.01549611932659545, 210.2015048109875011, 71.64886208192143613 ) ) ;
#21217=CARTESIAN_POINT ( 'NONE',  ( -3.753561863808691168, 195.6020594897209435, 101.9011379180785895 ) ) ;
#21219=CARTESIAN_POINT ( 'NONE',  ( 6.220909254589536808, 215.4770327129947702, 13.55113791807856849 ) ) ;
#21220=CARTESIAN_POINT ( 'NONE',  ( 9.984503880673420539, 210.2968891136705167, 81.84886208192143897 ) ) ;
#21222=CARTESIAN_POINT ( 'NONE',  ( -10.01549611932653860, 203.7984951890123284, 102.3511379180785781 ) ) ;
#21225=CARTESIAN_POINT ( 'NONE',  ( -0.05014649552828365914, 215.4116977939061144, 60.24886208192144466 ) ) ;
#21233=CARTESIAN_POINT ( 'NONE',  ( 8.015496119326531499, 209.5516654185219636, 55.85113791807856387 ) ) ;
#21236=CARTESIAN_POINT ( 'NONE',  ( -9.254041968259778983, 206.2987758111210894, 104.1628994045829870 ) ) ;
#21239=CARTESIAN_POINT ( 'NONE',  ( -2.426778023690076225, 199.3768101843759553, 31.89886208192144323 ) ) ;
#21240=CARTESIAN_POINT ( 'NONE',  ( -8.062137200540920645, 212.9164362838581894, 84.80113791807856671 ) ) ;
#21243=CARTESIAN_POINT ( 'NONE',  ( 3.044812012440130555, 197.4746971517856764, 68.60113791807857808 ) ) ;
#21245=CARTESIAN_POINT ( 'NONE',  ( 6.500168698208129925, 211.6636982574063381, 16.70113791807856529 ) ) ;
#21249=CARTESIAN_POINT ( 'NONE',  ( 12.00000000000000711, 206.9523078486586485, 44.00113791807856956 ) ) ;
#21252=CARTESIAN_POINT ( 'NONE',  ( -3.044812012440131443, 216.5253028482142952, 94.10113791807857808 ) ) ;
#21253=CARTESIAN_POINT ( 'NONE',  ( -9.984503880673475606, 210.2968891136704315, 54.65113791807858235 ) ) ;
#21254=CARTESIAN_POINT ( 'NONE',  ( 3.753561863808876797, 195.6020594897209719, 25.59886208192143897 ) ) ;
#21255=CARTESIAN_POINT ( 'NONE',  ( -9.984503880673420539, 203.7031108863293980, 35.34886208192143187 ) ) ;
#21257=CARTESIAN_POINT ( 'NONE',  ( -9.680171189290831535, 214.0920067884431148, 63.80113791807858092 ) ) ;
#21258=CARTESIAN_POINT ( 'NONE',  ( 2.426778023690261410, 199.3768101843759837, 92.60113791807857808 ) ) ;
#21259=CARTESIAN_POINT ( 'NONE',  ( -10.01549611932659722, 210.2015048109875011, 47.64886208192142192 ) ) ;
#21263=CARTESIAN_POINT ( 'NONE',  ( 9.680171189290716072, 214.0920067884432854, 51.69886208192144039 ) ) ;
#21270=CARTESIAN_POINT ( 'NONE',  ( -0.05014649552807731031, 198.5883022060938572, 38.75113791807856956 ) ) ;
#21272=CARTESIAN_POINT ( 'NONE',  ( 9.984503880673420539, 210.2968891136705167, 27.84886208192143187 ) ) ;
#21279=CARTESIAN_POINT ( 'NONE',  ( -6.444103211790928043, 202.2591342207265939, 2.198862081921435063 ) ) ;
#21280=CARTESIAN_POINT ( 'NONE',  ( -8.062137200540920645, 212.9164362838581894, 51.80113791807857382 ) ) ;
#21282=CARTESIAN_POINT ( 'NONE',  ( -8.118202686958039038, 201.1607312380087080, 39.20113791807857240 ) ) ;
#21285=CARTESIAN_POINT ( 'NONE',  ( -6.500168698208244500, 211.6636982574061676, 95.79886208192144181 ) ) ;
#21289=CARTESIAN_POINT ( 'NONE',  ( 3.753561863808689836, 218.3979405102790565, 10.40113791807856636 ) ) ;
#21292=CARTESIAN_POINT ( 'NONE',  ( 10.01549611932653860, 210.2015048109876716, 52.85113791807854966 ) ) ;
#21293=CARTESIAN_POINT ( 'NONE',  ( -9.984503880673475606, 210.2968891136704315, 27.65113791807856458 ) ) ;
#21296=CARTESIAN_POINT ( 'NONE',  ( 6.220909254589680693, 198.5229672870052582, 13.44886208192143329 ) ) ;
#21299=CARTESIAN_POINT ( 'NONE',  ( -9.736236675707914401, 199.9851607334237542, 39.20113791807857240 ) ) ;
#21301=CARTESIAN_POINT ( 'NONE',  ( -6.139770520408224463, 198.4640165459539389, 26.04886208192143471 ) ) ;
#21304=CARTESIAN_POINT ( 'NONE',  ( 9.984503880673470277, 203.7031108863295401, 77.15113791807857524 ) ) ;
#21310=CARTESIAN_POINT ( 'NONE',  ( 2.426778023690261410, 199.3768101843759837, 14.60113791807856742 ) ) ;
#21312=CARTESIAN_POINT ( 'NONE',  ( 12.01549611932659367, 203.1486557965466773, 100.1488620819214646 ) ) ;
#21318=CARTESIAN_POINT ( 'NONE',  ( -10.00000000000000711, 206.9523078486584495, 83.49886208192143044 ) ) ;
#21320=CARTESIAN_POINT ( 'NONE',  ( -0.05014649552810635652, 196.4853777576173002, 20.75113791807855890 ) ) ;
#21325=CARTESIAN_POINT ( 'NONE',  ( -10.00000000000000711, 207.0476921513413515, 87.50113791807858377 ) ) ;
#21326=CARTESIAN_POINT ( 'NONE',  ( -10.00000000000019362, 205.9534653805592654, 104.4507591396482127 ) ) ;
#21328=CARTESIAN_POINT ( 'NONE',  ( -7.456977232089471386, 217.1783343296987709, 98.94886208192143329 ) ) ;
#21332=CARTESIAN_POINT ( 'NONE',  ( -4.927659837809095222, 206.3103720916592465, -5.504302862921502282 ) ) ;
#21338=CARTESIAN_POINT ( 'NONE',  ( -3.044812012439970683, 197.4746971517856196, 97.89886208192145034 ) ) ;
#21340=CARTESIAN_POINT ( 'NONE',  ( -0.05014649552828442242, 219.6175466908591716, 36.24886208192142334 ) ) ;
#21342=CARTESIAN_POINT ( 'NONE',  ( -0.05014649552810635652, 196.4853777576173002, 47.75113791807855534 ) ) ;
#21345=CARTESIAN_POINT ( 'NONE',  ( 2.517493886309087436, 199.4062855549015865, 4.598862081921435419 ) ) ;
#21348=CARTESIAN_POINT ( 'NONE',  ( -2.517493886309087880, 214.5937144450984135, 87.09886208192143897 ) ) ;
#21350=CARTESIAN_POINT ( 'NONE',  ( -8.015496119326531499, 204.4483345814780364, 27.35113791807856742 ) ) ;
#21357=CARTESIAN_POINT ( 'NONE',  ( -8.000000000000008882, 207.0476921513413515, 99.50113791807856956 ) ) ;
#21361=CARTESIAN_POINT ( 'NONE',  ( -7.984503880673422316, 204.3529502787951628, 74.34886208192142476 ) ) ;
#21366=CARTESIAN_POINT ( 'NONE',  ( -8.118202686958039038, 201.1607312380087080, 12.20113791807856707 ) ) ;
#21371=CARTESIAN_POINT ( 'NONE',  ( -7.375838497908182134, 217.2372850707499765, 75.95113791807857240 ) ) ;
#21373=CARTESIAN_POINT ( 'NONE',  ( -3.135527875058821579, 197.5041725223112223, 98.90113791807857524 ) ) ;
#21377=CARTESIAN_POINT ( 'NONE',  ( -3.662846001189865142, 195.5725841191952838, 61.89886208192143613 ) ) ;
#21379=CARTESIAN_POINT ( 'NONE',  ( 10.01549611932659367, 203.7984951890124421, 67.14886208192143613 ) ) ;
#21380=CARTESIAN_POINT ( 'NONE',  ( -12.01549611932659722, 210.8513442034533227, 8.648862081921436129 ) ) ;
#21382=CARTESIAN_POINT ( 'NONE',  ( -3.135527875058821579, 197.5041725223112223, 11.90113791807856636 ) ) ;
#21383=CARTESIAN_POINT ( 'NONE',  ( 10.01549611932659545, 203.7984951890123853, 79.14886208192142192 ) ) ;
#21385=CARTESIAN_POINT ( 'NONE',  ( -8.062137200540920645, 212.9164362838581894, 96.80113791807858092 ) ) ;
#21389=( BOUNDED_SURFACE ( )  B_SPLINE_SURFACE ( 3, 2, ( 
 ( #25089, #1418, #19648, #1747, #4476, #12146, #25261, #4652, #4135, #11810, #1586, #25428, #30037, #30723, #22541, #1927, #33097, #6702, #20319, #15036, #12313, #7208, #12489, #15210, #22709, #17594, #17762, #7383, #14527, #24928, #4816, #7558, #31551, #31387, #23390, #17945, #15875, #10112, #20491, #10778, #4991, #8219, #13322, #30894, #54, #18607, #25935, #28333, #2779, #15378, #20668, #31062, #28994, #219, #5653, #25601, #10289, #20824, #25770, #12996, #2267, #18272, #26270, #23713, #12822, #2938, #28661, #12649, #5155, #2610, #23214, #10450, #5487, #374, #8058, #7721, #2442, #5320, #21153, #31227, #33610, #18107, #28502, #23045, #15543, #33440, #7891, #15709, #26111, #13158, #23550, #10616, #20991, #18441, #28830, #19780, #7173, #4779, #12278, #22503, #27604, #17558, #27775, #19612, #11948, #25227, #12613, #33233, #4272, #22329, #22669, #30688, #17391, #30341, #17217, #27950, #9551, #2064, #14665, #30004, #9384, #17731, #12112, #1891, #27446, #28117, #17051, #12452, #32717, #25392, #22843, #9899, #30175, #6832, #4620, #19942, #1550, #6665, #4440, #20282, #15002, #7351, #25059, #1713, #7005, #15174, #25566, #33406, #32891, #33057, #2231, #14829, #24889, #9726, #20116, #30508, #23009, #4100, #14489, #2402, #336, #28299, #4952, #28955, #23179, #16006, #31516, #15339, #7854, #26398, #10413, #12789, #20957, #33570, #5119, #15509, #3056, #18403, #13444, #23838, #28463, #5280, #10251, #31185, #10079, #2746, #10736, #8186, #31028, #21118, #13119, #20457, #23354, #20786, #7684, #18238, #23677, #18570, #15838, #25900, #20626, #23512, #5614, #28627, #18067, #2570, #12958, #30855, #17, #7519, #17905, #180, #15674, #25732, #26076, #10579, #31350, #8017, #28796, #5452, #26227, #2898, #13285, #29287, #31836, #16667, #29626, #3726, #11226, #27063, #29121, #29451, #13946, #13779, #16837, #512, #11071, #26897, #29793, #18892, #8829, #3886, #837, #18735, #16162, #24510, #5939, #26722, #6275, #8501, #32340, #16498, #6457, #11402, #24175, #3556, #31676, #14116, #21611, #8346, #26553, #9005, #27232, #19394, #14280, #13610, #19231, #668, #21282, #5769, #10905, #1167, #32006, #11563, #16330, #3223, #24005, #21452, #3384, #24335, #8670, #19063, #6101, #21951, #1006, #21779, #32169, #27902, #24843, #17002, #22621, #25018, #6617, #24682, #32844, #17513, #12234, #12406, #14449, #27396, #25348, #27736, #4059, #19731, #1506, #11904, #9507, #1672, #22290, #9178, #7311, #30128, #19894, #9857, #4399, #14784, #32505, #22451, #9679, #22803, #6960, #20072, #30293, #33009, #25176, #32672, #17349, #19568, #1845, #4736, #11730, #33193, #9338, #29961, #17174, #6787, #2017, #27559, #30469, #7130, #4223, #20239, #14622, #4575, #12063, #14961, #30642, #1343, #17687, #28074, #22117, #28420, #28591, #7979, #17857, #15126, #15295, #5413, #33364, #10698, #2529, #12912, #13082, #2358, #18363, #13243, #15798, #30810, #25689, #23640, #10373, #2191, #25863, #23141, #20417, #26189, #33529, #23307, #8148, #12750, #2705, #300, #7809, #18027, #10202, #23472, #25516, #25522, #7472, #20746, #18530, #28755, #20584, #28254, #18200, #2858, #31142, #5242, #30988, #138, #7644, #21077, #10039, #31479, #15631, #26034, #10540, #5076, #28913, #12574, #22966, #4909, #15473, #20921, #31314, #26360, #16293, #13576, #10867, #29584, #23966, #26684, #32302, #5732, #26853, #24469, #31960, #8463, #630, #3514, #13734, #5571, #31636, #11188, #8964, #19188, #11027, #8303, #8629, #16625, #3344, #24132, #3185, #13906, #29247, #21740, #21409, #15965, #29084, #3680, #31796, #21567, #13404, #14072, #3019, #32130, #18694, #11358, #8792, #6237, #16122, #26516, #24290, #5898, #21243, #23799, #799, #27019, #960, #1130, #18850, #19024, #11524, #29412, #6062, #16454, #21905, #19355, #470, #30556, #29924, #14241, #12833, #1936, #4662, #15388, #9946, #20332, #3849, #27996, #15220, #17955, #12498, #25610, #15046, #4829, #30732, #6577, #2114, #24639, #7392, #10300, #16794, #28345, #14877, #1305, #22719, #19528, #7569, #9131, #28170, #12660, #16961, #30903, #11695, #2276, #22077, #23058, #27355, #29749, #32463, #4486, #25438, #9775, #17773, #33451, #25271, #6412, #20159, #12325, #33109, #10121, #20502, #22887, #23224, #7218, #33279, #17606, #5000, #25785, #2452, #33619, #27193, #23889, #31399, #13494, #15552, #15885, #386, #232, #3269, #20676, #31238, #13332, #16215, #5329, #29003, #24050, #21001, #5165, #2619, #10950, #26120, #13168, #26441, #18282, #18781, #2951, #26606, #31560, #10626, #23723, #18117, #3106, #8067, #28515, #13007, #29168, #13657, #5820, #719, #63, #5664, #20835, #7731, #25945, #31073, #557, #18453, #16051, #21325, #23400, #28671, #26279, #10461, #15721, #7901, #2788, #23562, #28840, #5496, #31722, #10788, #21163, #8394, #8227, #18616, #30008, #24221, #17057, #32553, #5989, #8884, #27450, #11449, #3434, #22004, #884, #6155, #16549, #4104, #19443, #14496, #24895, #29501, #6324, #11281, #32219, #11122, #3780, #11776, #9228, #32059, #1388, #14167, #21498, #24393, #21828, #8721, #19280, #24734, #22166, #16884, #26944, #21664, #24560, #19618, #29672, #19111, #3603, #13997, #31885, #1060, #6670, #8552, #1217, #16717, #27118, #11615, #32387, #18945, #9051, #29342, #16377, #29846, #26769, #6506, #13831, #27281, #3938, #14338, #33062, #15179, #25572, #7357, #7010, #25064, #4625, #2236, #20120, #22509, #12118, #17396, #22335, #32896, #12620, #32722, #25396, #25233, #19785, #9556, #2068, #12455 ),
 ( #9731, #12283, #19948, #33240, #1896, #17736, #30347, #11953, #1718, #33412, #27782, #17563, #9389, #10086, #30180, #28125, #4278, #4786, #23015, #20463, #4446, #27610, #9906, #22675, #17223, #1555, #30514, #30863, #22848, #7527, #14834, #14670, #17912, #15007, #7179, #27956, #20288, #30694, #28304, #4960, #15347, #6837, #8353, #31194, #188, #10912, #5460, #15846, #33579, #23520, #10745, #13452, #8026, #21125, #10586, #343, #26235, #2579, #31357, #20633, #2906, #5775, #12794, #23845, #10421, #10258, #18245, #15515, #3063, #5127, #23683, #8193, #25738, #25906, #16012, #31034, #21289, #13127, #20963, #31523, #12965, #28962, #519, #26404, #7692, #23361, #31683, #18411, #23185, #2752, #24, #18075, #18741, #20793, #28803, #29127, #7860, #13291, #2409, #18578, #28634, #5289, #5620, #28470, #15682, #26083, #21786, #9186, #29802, #24182, #18900, #8837, #27238, #13953, #26905, #13787, #14122, #6109, #32348, #11232, #26560, #5946, #14287, #8677, #32177, #24013, #24690, #13616, #9012, #29295, #21959, #19401, #6463, #16337, #8506, #24516, #16506, #31842, #16170, #24344, #16844, #3733, #3892, #26731, #3392, #1349, #19239, #844, #21619, #32013, #19069, #1013, #3563, #29458, #677, #32513, #11408, #29634, #11736, #6281, #16674, #11079, #27071, #1173, #22123, #11570, #19575, #29968, #3229, #21460, #17182, #12241, #1514, #30475, #20423, #27405, #4741, #25026, #14455, #32852, #30136, #17693, #19740, #4580, #22808, #27565, #7316, #11911, #25354, #22297, #33199, #4232, #6626, #24851, #14630, #1851, #19902, #20080, #9862, #9344, #2024, #25183, #14966, #7137, #1679, #22627, #32678, #17520, #17011, #4067, #15133, #12072, #6794, #9515, #22460, #28080, #30301, #12412, #20244, #6969, #25528, #17357, #30648, #27743, #2197, #4406, #14791, #33015, #9686, #27909, #12579, #22972, #33371, #10046, #30816, #30994, #21083, #15303, #26366, #18206, #28597, #28762, #18033, #306, #28919, #31487, #12756, #7651, #5579, #26041, #17864, #7816, #5083, #2366, #8154, #15479, #5248, #23805, #28428, #18370, #15972, #23478, #15717, #25870, #5419, #15637, #7480, #23147, #2712, #477, #10705, #2536, #33535, #145, #18537, #13089, #10546, #12919, #15804, #20752, #13250, #23315, #28262, #20593, #3025, #10379, #20927, #4916, #13411, #25695, #23646, #10208, #2865, #10874, #31149, #31320, #7986, #26197, #21574, #3193, #21249, #29418, #14080, #8798, #8970, #11034, #13582, #21911, #24298, #23973, #16300, #635, #31803, #6068, #31966, #21416, #5738, #3854, #26690, #16462, #6418, #966, #11367, #29090, #19030, #6243, #19360, #3520, #16129, #29755, #18702, #24475, #8469, #27027, #1136, #11530, #18857, #29253, #19195, #8637, #5905, #31643, #26861, #32308, #29592, #16801, #3351, #13741, #27198, #21746, #24138, #805, #11195, #13913, #32136, #16631, #3687, #26521, #14246, #24645, #1311, #8310, #25141, #1805, #19535, #9474, #30436, #33159, #27703, #7096, #30260, #20036, #12202, #22254, #17313, #6582, #22589, #25483, #32469, #9822, #30089, #29929, #4189, #1472, #22766, #24811, #9641, #27862, #32641, #12370, #16966, #17477, #27361, #4535, #9304, #11700, #4027, #19696, #6922, #24986, #32975, #14927, #14418, #22083, #11867, #1979, #6755, #7269, #32807, #19862, #25315, #17142, #20203, #30603, #17651, #27528, #14585, #28039, #4365, #9137, #22417, #1637, #12029, #4700, #14748, #15090, #28881, #2322, #23439, #21043, #28560, #5044, #10162, #104, #10341, #2157, #28215, #7775, #5537, #15764, #20545, #4874, #5208, #13209, #33665, #12877, #33493, #10506, #25830, #18325, #30947, #12540, #25655, #272, #28387, #18166, #28720, #7612, #22930, #20382, #23105, #31113, #15434, #15594, #5376, #15263, #33325, #12709, #26159, #30774, #31446, #23270, #20713, #20885, #17996, #2825, #10667, #23608, #17817, #2494, #8114, #25996, #9996, #2666, #13049, #7436, #18496, #31283, #7943, #15927, #26484, #13874, #11496, #18994, #29213, #596, #24258, #763, #26325, #18658, #31927, #19324, #6203, #10992, #29048, #29384, #3648, #24096, #3312, #23934, #928, #16262, #8764, #21371, #2990, #16090, #24439, #18819, #8598, #432, #1103, #23767, #19152, #5702, #32101, #29549, #16592, #3153, #13540, #11326, #26648, #8270, #13370, #11162, #26984, #21710, #14043, #31767, #8433, #21874, #6030, #5865, #13696, #21537, #16422, #26818, #3482, #32266, #10834, #8934, #29713, #6375, #21209, #31603, #30229, #24609, #14548, #1768, #4497, #32770, #12168, #1604, #25107, #6884, #27326, #22382, #11664, #17274, #30565, #3820, #14888, #1434, #1271, #9270, #6548, #27827, #29894, #14714, #32945, #3991, #17443, #22048, #22560, #32431, #7061, #9606, #22216, #16931, #19833, #25281, #11995, #14388, #24778, #32605, #14212, #11830, #1946, #9098, #27663, #6721, #19494, #19664, #4330, #20001, #9443, #9784, #30054, #30400, #17112, #12334, #27496, #4151, #22731, #33119, #20168, #24947, #16766, #27164, #2460, #20684, #20510, #23573, #7228, #17782, #33630, #2796, #25619, #15559, #10634, #7578, #25450, #22896, #31247, #12670, #33458, #13016, #4840, #5340, #23233, #13177, #18126, #30913, #10308, #4671, #23408, #17964, #15055, #33289, #15731, #242, #26128, #21010, #20343, #25954, #7401, #28005, #2125, #17618, #20845, #28354, #2631, #7909, #12508, #15230, #12841, #9956, #2286, #30742, #28182, #23066, #10130, #5008, #71, #15397, #25795, #18290, #31082, #7741, #28524, #5173, #10471, #28679, #26288, #29640, #4073, #32185, #24189, #9019, #11243, #26912, #3570, #14461, #6469 ),
 ( #6633, #24858, #17019, #1521, #21628, #16852, #32021, #18462, #5504, #27413, #11742, #19245, #27245, #22129, #11917, #6117, #3741, #31407, #13959, #2961, #8685, #19076, #13795, #8077, #3899, #6287, #851, #32519, #15893, #29465, #28849, #16513, #24354, #19582, #1021, #16681, #11416, #8845, #21793, #19408, #27078, #14130, #24524, #1180, #14295, #11576, #21966, #32354, #29810, #24697, #1354, #9192, #29975, #22977, #20428, #9522, #12584, #14974, #4922, #1859, #33024, #19909, #20086, #2202, #33377, #28087, #27749, #12078, #25361, #10051, #7143, #30309, #32860, #4412, #9351, #6976, #30821, #19747, #12420, #12248, #6801, #17363, #22814, #33205, #4588, #15308, #25033, #17528, #22636, #15141, #14798, #25191, #4750, #17699, #25534, #9694, #7488, #17188, #27916, #2033, #30481, #25700, #22303, #9868, #20251, #17872, #30656, #7323, #2373, #28267, #27573, #4239, #32683, #30144, #14636, #1685, #22469, #10879, #28768, #18708, #23651, #2716, #5423, #10215, #18541, #23483, #20598, #28433, #5583, #15485, #28923, #15978, #26370, #12925, #5090, #10709, #13093, #25876, #12762, #20932, #3030, #310, #482, #2542, #23321, #13415, #15808, #11360, #7823, #10385, #20757, #31324, #149, #31155, #31000, #29094, #18211, #7990, #31647, #26201, #2869, #7656, #10553, #31492, #21254, #13255, #8159, #18376, #21090, #23810, #28602, #8314, #18039, #5742, #26527, #33540, #16134, #5253, #15646, #26046, #23152, #14251, #16305, #1141, #19365, #24143, #3858, #8472, #21916, #31807, #29759, #809, #3198, #21421, #11199, #32140, #16467, #16635, #6425, #5910, #13586, #3356, #27202, #18861, #32474, #24302, #973, #11534, #21578, #16806, #1316, #24650, #29259, #13747, #11704, #8802, #23979, #13917, #31973, #26694, #22089, #8643, #11372, #29933, #19034, #24479, #9143, #29598, #6072, #29423, #32312, #21751, #640, #26867, #19199, #6587, #19540, #3524, #6248, #27031, #16970, #3695, #14085, #8978, #11038, #17319, #9828, #22421, #4033, #17146, #25490, #19868, #9645, #1478, #2161, #24815, #6761, #27532, #9308, #33330, #33164, #25145, #19700, #17656, #11874, #22259, #12544, #4194, #10002, #15094, #32646, #1810, #20386, #27709, #30094, #4541, #14594, #32812, #9478, #30779, #1985, #7440, #27366, #12034, #22593, #24991, #14752, #14422, #20042, #28043, #22935, #1642, #4705, #30441, #30264, #6926, #4370, #12206, #32981, #7273, #7101, #20208, #17481, #27866, #14931, #25319, #12375, #22772, #30608, #33671, #4879, #28391, #18502, #15267, #7949, #7779, #2327, #5048, #18332, #28725, #109, #10842, #20549, #2674, #31117, #10671, #12882, #15440, #276, #13213, #21050, #28565, #31451, #12715, #13054, #31288, #18170, #439, #17820, #25836, #10511, #13375, #2498, #26162, #21215, #5213, #23109, #33497, #8120, #23275, #10346, #23611, #20717, #15932, #20890, #23773, #5383, #15599, #15769, #25659, #28887, #26002, #10169, #30956, #26330, #31609, #2996, #28222, #7616, #2829, #18000, #23444, #5542, #16771, #21879, #29390, #26992, #32273, #22053, #16270, #13880, #24615, #3319, #13547, #1275, #8940, #26656, #10998, #933, #19330, #6037, #19000, #5871, #6209, #31933, #24444, #13703, #18663, #31771, #6383, #770, #24263, #16095, #27170, #5707, #1108, #21377, #14048, #11501, #29720, #8438, #602, #16598, #8603, #23940, #8277, #16428, #3825, #29555, #14217, #18825, #29219, #11670, #11331, #24102, #11167, #21543, #26824, #3488, #21716, #32106, #26490, #29054, #8769, #19159, #3158, #3654, #17280, #6552, #11999, #12171, #27831, #19836, #22563, #32774, #1771, #27667, #11835, #30232, #16935, #4335, #9789, #19500, #4501, #19667, #27331, #17115, #1440, #17448, #24784, #25110, #32948, #22220, #14891, #3995, #9609, #14392, #20005, #9273, #32437, #32610, #30059, #6888, #14553, #14718, #30405, #6724, #9104, #27499, #25284, #4156, #33122, #9446, #7066, #1950, #24951, #12338, #22735, #29899, #1609, #22385, #27277, #24388, #16211, #6150, #3429, #714, #19438, #13825, #16544, #22160, #29337, #16712, #14331, #21824, #32055, #24217, #27114, #3598, #29163, #21494, #1056, #29842, #880, #26940, #32548, #5984, #3776, #24727, #32215, #8717, #11277, #14162, #13992, #5815, #31879, #11445, #9223, #9046, #21660, #8547, #8878, #6502, #19275, #29668, #26765, #24557, #19108, #11609, #29496, #26601, #18941, #3934, #6318, #1213, #3264, #1382, #13653, #21998, #16372, #32383, #16880, #11770, #24046, #11117, #12308, #23039, #14860, #4986, #20485, #15373, #25084, #20314, #12141, #32746, #19811, #30888, #25596, #33092, #30718, #2262, #25765, #19973, #17589, #28328, #7037, #17249, #1742, #22536, #27637, #17940, #17757, #9761, #4306, #12644, #30204, #6861, #7553, #32921, #11972, #33435, #14692, #20144, #22357, #22703, #9580, #22873, #30375, #17419, #27804, #9416, #7378, #4471, #25256, #1922, #7203, #30540, #27980, #4647, #15031, #10107, #25423, #2097, #12484, #33264, #9931, #28154, #4811, #15205, #214, #16036, #26427, #8214, #7886, #25930, #5481, #3090, #20986, #23385, #12991, #18267, #23210, #49, #13479, #33605, #26265, #26106, #20663, #10445, #5802, #21148, #2436, #10611, #28989, #23708, #23872, #2604, #28497, #544, #15870, #18102, #31222, #5150, #20819, #31382, #2773, #28656, #31057, #18768, #5315, #8052, #21312, #2933, #13316, #10284, #18436, #31546, #10936, #28825, #18602, #369, #10772, #5648, #15704, #31708, #7716, #8380, #16198, #15538, #29151, #13153, #23545, #12817, #16360, #3920, #5972, #24544, #9035, #13813, #27263, #31868, #11596, #21484 ),
 ( #29830, #24716, #16870, #8533, #3417, #1372, #21811, #13641, #3587, #869, #18928, #14318, #11265, #13980, #19602, #26754, #14148, #11760, #19264, #29483, #21647, #1198, #1042, #26588, #29324, #32203, #29994, #6491, #32042, #24206, #29657, #22148, #24376, #11434, #8705, #21985, #16532, #19427, #19095, #3253, #6138, #32536, #26929, #8865, #703, #9212, #24035, #6651, #6306, #32371, #11105, #16701, #27101, #3763, #9714, #20270, #17206, #17545, #20105, #20446, #2052, #17039, #25214, #9887, #4609, #4768, #6821, #9372, #17720, #30498, #32705, #12100, #19767, #27593, #1880, #17381, #4260, #1539, #33397, #22492, #12265, #2219, #7161, #27938, #24876, #14817, #12440, #15162, #33045, #22831, #22657, #25381, #14992, #14654, #33223, #11936, #30676, #30845, #4089, #25555, #1703, #22319, #9539, #25050, #28107, #30163, #7341, #12603, #32879, #22998, #19930, #10069, #30328, #27433, #6995, #14479, #27765, #4429, #2737, #20776, #20947, #326, #10241, #7509, #7675, #31508, #25721, #3047, #28619, #5271, #5444, #28452, #10727, #5603, #8176, #23171, #18057, #15996, #13111, #28287, #18229, #15502, #12780, #18561, #25892, #15665, #501, #5111, #28787, #26388, #169, #10403, #2561, #15829, #26067, #17893, #33562, #23502, #10895, #21109, #12949, #20619, #10569, #28946, #31341, #8009, #23344, #26219, #31173, #23666, #8, #4941, #31018, #13432, #7844, #18394, #15327, #23830, #2393, #21272, #2887, #13274, #24500, #3717, #29279, #29783, #13937, #3878, #8819, #21600, #24325, #29111, #14105, #5930, #31996, #8996, #828, #24671, #6448, #1335, #11062, #6266, #31826, #18727, #5760, #16829, #11552, #19052, #16657, #21940, #11722, #16322, #3545, #14271, #26713, #3215, #21444, #8492, #13601, #31668, #1159, #29442, #23997, #32330, #16153, #26544, #27223, #18884, #8336, #19385, #659, #6090, #3375, #8661, #13769, #19221, #24166, #11218, #16488, #26887, #27054, #996, #11393, #21770, #32159, #29618, #9500, #28066, #14776, #22793, #20230, #9329, #12397, #25168, #4727, #1663, #32835, #19721, #19886, #2008, #33185, #27891, #27551, #11896, #1836, #9848, #6950, #30118, #32664, #4214, #9167, #6780, #30632, #19560, #12226, #12055, #6608, #17165, #22614, #33001, #4390, #15117, #24835, #17341, #22444, #14953, #14614, #25010, #4565, #17504, #25339, #30284, #7300, #16992, #27729, #9669, #20062, #25512, #22108, #30461, #7121, #17678, #2181, #32495, #29952, #27387, #4051, #14442, #1499, #22281, #5069, #26183, #2851, #18353, #18020, #2350, #15622, #13236, #31135, #33518, #23131, #28411, #33354, #10193, #23632, #10028, #2697, #2519, #30801, #20575, #13074, #23464, #28583, #6016, #15287, #7800, #25856, #5406, #7637, #30978, #28747, #7969, #15790, #23299, #293, #7463, #18190, #26025, #12904, #29371, #12566, #15463, #5233, #8584, #28782, #20911, #16407, #10365, #17845, #28245, #10689, #20739, #130, #21070, #10531, #31912, #31306, #18978, #26801, #22958, #20408, #4901, #25682, #12740, #3807, #14528, #6356, #30210, #11978, #6867, #16578, #11811, #3631, #24245, #11311, #22363, #17094, #24592, #22199, #27479, #17256, #11479, #9081, #19817, #32249, #8749, #26969, #14025, #19138, #9423, #9255, #1252, #29533, #4136, #21696, #32087, #32752, #24424, #3464, #24929, #6189, #11649, #13860, #14196, #1088, #14371, #21857, #8917, #19309, #912, #32589, #29698, #16747, #27149, #32416, #22033, #19477, #29877, #6534, #1588, #16914, #27310, #3971, #24764, #1419, #19649, #30039, #6704, #25429, #22710, #9586, #4477, #2104, #27987, #27810, #12147, #10290, #33098, #12490, #12824, #7384, #17764, #1748, #22879, #12650, #15379, #9938, #23048, #33270, #2268, #28161, #14866, #20322, #22543, #4818, #7722, #14698, #25773, #12315, #32927, #20149, #17426, #4992, #7043, #25602, #10113, #25263, #28335, #19980, #33442, #30382, #20492, #1928, #27644, #9767, #30547, #30724, #7209, #15211, #30895, #17596, #4313, #4653, #17946, #15037, #23215, #7560, #2444, #33611, #20669, #31064, #25090, #8386, #55, #28662, #16206, #13323, #5156, #28831, #26112, #23391, #18774, #2780, #5488, #11113, #18273, #5655, #3260, #10779, #20992, #13160, #16042, #26271, #18108, #10451, #23714, #21491, #31714, #23551, #20825, #21155, #29157, #15877, #2940, #15711, #26433, #8059, #550, #221, #28504, #7892, #26596, #10617, #376, #25936, #13649, #15544, #10943, #31229, #23879, #21318, #5810, #5321, #18609, #31552, #31875, #3097, #2611, #8220, #24042, #13486, #710, #31389, #18443, #12997, #28995, #24213, #8712, #876, #14485, #14326, #6314, #11273, #32544, #26762, #3425, #27441, #21654, #24885, #30000, #13821, #16708, #1546, #8874, #32050, #19434, #19103, #3594, #13988, #11944, #16876, #22325, #8541, #26936, #3772, #29492, #29664, #18936, #1207, #9219, #6658, #6146, #19608, #11604, #29332, #21819, #19271, #16540, #27110, #22156, #17046, #24722, #24384, #1050, #21994, #4095, #14156, #11441, #32210, #24552, #5979, #32379, #16368, #9042, #29838, #6498, #27271, #3928, #1378, #11766, #14998, #25728, #1709, #17553, #12272, #25561, #27771, #30336, #15169, #28113, #2226, #9721, #12609, #27600, #27946, #12447, #22664, #15335, #32713, #9546, #25386, #28294, #17388, #7347, #2400, #33052, #17212, #14661, #23005, #4436, #25222, #4774, #7002, #30851, #2059, #4947, #9895, #20112, #22837, #30170, #33403, #14824, #30504, #10075, #1887, #12786, #7516, #9380, #12107, #17727, #32886, #19774, #6827, #17900, #20453, #7169, #4268, #25055, #22499, #4616, #33229, #19937, #20277 ),
 ( #30684, #2893, #14, #28794, #18062, #13280, #3220, #10248, #21279, #7850, #31024, #15671, #12956, #509, #2567, #21115, #5610, #10409, #23835, #28458, #8182, #5116, #16002, #20781, #23176, #7681, #31180, #18400, #2743, #23672, #26394, #25897, #33567, #23351, #13439, #15507, #18732, #10575, #20953, #31514, #18235, #3052, #31673, #10901, #28624, #5276, #8342, #5448, #20624, #176, #26073, #13117, #29117, #23508, #31347, #16158, #8014, #10732, #5765, #15835, #26224, #332, #18567, #28952, #26549, #5935, #19228, #6615, #27230, #21607, #16327, #6272, #24678, #11399, #24332, #11223, #11560, #3551, #29789, #8667, #24002, #3381, #11728, #6098, #29624, #21449, #22115, #11067, #6455, #26719, #19392, #16835, #3884, #13775, #14114, #16664, #17000, #32338, #13606, #21777, #14278, #1165, #1341, #24171, #834, #32502, #27060, #29284, #19058, #32002, #29448, #3724, #19566, #24507, #13944, #21948, #31832, #9175, #16495, #1004, #29959, #26894, #27393, #665, #8498, #32166, #9002, #8827, #18888, #11901, #12571, #17684, #25174, #22799, #28071, #17853, #12061, #9675, #20413, #32842, #9336, #17171, #4220, #19729, #10034, #9854, #1842, #30125, #4734, #22287, #32670, #22963, #27557, #30807, #25519, #6785, #12232, #7469, #4395, #14620, #14958, #25015, #9505, #19892, #4056, #12402, #14447, #24841, #22449, #33007, #1669, #22619, #1504, #30467, #15123, #2187, #30290, #33361, #7127, #6956, #17347, #14781, #27734, #20070, #17509, #27898, #20236, #4571, #25345, #2014, #33190, #30638, #7306, #5073, #10370, #15291, #15469, #28910, #25686, #18360, #18196, #12746, #25860, #28751, #5410, #10537, #21239, #30985, #13079, #7805, #21074, #23303, #2524, #10695, #23637, #31475, #5239, #8144, #23136, #23469, #7976, #28588, #10864, #28251, #12908, #20916, #23796, #26602, #2855, #31633, #15627, #33525, #10199, #18527, #20743, #31139, #296, #26029, #26357, #466, #31311, #5568, #3016, #2702, #15962, #15795, #8300, #135, #26186, #13240, #13400, #4906, #2355, #20580, #7641, #18024, #28416, #8961, #3512, #5895, #29245, #797, #5729, #16291, #19352, #16119, #8790, #8626, #3181, #26681, #19186, #29581, #958, #11694, #21407, #13904, #31958, #11522, #13730, #3342, #1128, #14069, #21903, #29410, #32300, #13573, #24288, #32128, #19022, #1304, #18691, #24129, #11355, #14239, #11186, #27017, #22075, #6060, #23964, #627, #29746, #21565, #16452, #24467, #26850, #16791, #21738, #24637, #6233, #16622, #3678, #26512, #6410, #27191, #3847, #32461, #29081, #11025, #31794, #8461, #18848, #17470, #9296, #29922, #16960, #17644, #22760, #30253, #27855, #33152, #22924, #17136, #14741, #25478, #4182, #14413, #22244, #19690, #24806, #15083, #14918, #6915, #1463, #9816, #27354, #4021, #28031, #32634, #2150, #30596, #11860, #17307, #12534, #9468, #30082, #20030, #6747, #14577, #24977, #9129, #4527, #19526, #6576, #27522, #4357, #1630, #27693, #20195, #12022, #25308, #22409, #1972, #32800, #19856, #25133, #1796, #12196, #22583, #32968, #12363, #9634, #30429, #7088, #7260, #4693, #28870, #20705, #31105, #31276, #20536, #2818, #31435, #23601, #15255, #10153, #8105, #28553, #20374, #10333, #7604, #4866, #266, #17987, #7767, #26316, #33485, #20877, #18487, #25987, #2486, #28379, #7936, #18158, #33317, #25648, #5199, #2983, #13201, #5036, #2315, #2658, #10660, #15584, #13041, #30941, #18316, #23262, #15755, #15426, #9987, #23096, #5528, #25822, #23432, #7426, #15918, #30767, #26151, #12700, #5368, #21034, #13363, #12868, #96, #10497, #17811, #28709, #28209, #33656, #16584, #11317, #11486, #13532, #16083, #24431, #26808, #5694, #18811, #26475, #588, #31918, #24087, #23923, #8260, #6362, #29204, #8590, #8924, #3472, #13865, #31594, #21529, #8755, #21864, #6022, #19143, #18987, #32093, #24251, #10983, #29377, #18650, #918, #3812, #10825, #32257, #8425, #29041, #16255, #21361, #1095, #3144, #21702, #6195, #31758, #5856, #26641, #26974, #29539, #3637, #755, #14033, #3303, #16413, #19315, #13687, #16757, #23758, #11155, #29704, #27156, #423, #21199, #18070, #14536, #32422, #29886, #4956, #19655, #6711, #19989, #11818, #12791, #30219, #20630, #25097, #4143, #6875, #11656, #30390, #22207, #24938, #25734, #17103, #7688, #23181, #28466, #27317, #22551, #14379, #1261, #22039, #33575, #28301, #1596, #32936, #15342, #14203, #32596, #19824, #31030, #9262, #19485, #3981, #24770, #6540, #24600, #7523, #11985, #16920, #2405, #9087, #1426, #10254, #30045, #27488, #22371, #32760, #9432, #17263, #27653, #4320, #1758, #14705, #12157, #9596, #17908, #13448, #11075, #8503, #23515, #339, #5285, #26230, #21456, #31519, #5771, #3225, #26079, #29124, #8189, #31838, #18407, #15842, #2749, #2902, #18738, #16167, #10908, #10582, #28630, #18574, #26556, #23679, #13123, #15678, #20960, #25903, #184, #13613, #2575, #28958, #28799, #23357, #31353, #5616, #16008, #21122, #18896, #7856, #10741, #5455, #31679, #26400, #3059, #5123, #18241, #23842, #13288, #8349, #8022, #515, #21285, #24009, #671, #15511, #12962, #20, #10417, #20788, #31190, #11908, #29291, #6104, #21954, #24847, #13949, #3888, #32675, #29630, #13783, #11228, #19571, #1009, #21782, #1345, #26901, #27401, #11565, #1511, #6459, #19235, #32344, #26727, #11732, #3559, #6277, #6622, #32173, #22293, #4063, #9341, #8673, #14282, #29454, #16333, #3387, #14452, #9182, #16670, #24686, #29964, #5942, #24340, #1170, #24179, #11404, #840, #19065, #16502, #21615, #32010, #22119 ),
 ( #32510, #8832, #27067, #3729, #24512, #14118, #9008, #19397, #29798, #17006, #16840, #27234, #10042, #12410, #2361, #33011, #30471, #17354, #17517, #33367, #20419, #25525, #25179, #9511, #22805, #30812, #4577, #6965, #30297, #1847, #6790, #27739, #7475, #17178, #9859, #9682, #4228, #4402, #20241, #7313, #27905, #19735, #12068, #25351, #12752, #17860, #14787, #22455, #33195, #28258, #14963, #7133, #12237, #17690, #20076, #2194, #22623, #30132, #19898, #4912, #2021, #30644, #27562, #15299, #14626, #12576, #32848, #22969, #25691, #23143, #28077, #4739, #15130, #33531, #25022, #1675, #18366, #3021, #31483, #31638, #20066, #2532, #10870, #13245, #25866, #5244, #12915, #20748, #28758, #10542, #10375, #28424, #26518, #15633, #5415, #29086, #23642, #302, #18029, #7982, #28915, #8306, #26193, #5575, #15800, #18533, #10701, #31145, #2861, #5078, #21079, #23969, #30990, #18697, #28594, #15475, #2707, #7811, #21245, #23311, #8150, #26362, #18202, #5734, #26037, #15967, #13085, #13407, #23474, #10204, #141, #20923, #23801, #31316, #473, #16125, #3189, #20589, #13578, #7647, #31799, #3683, #8633, #19026, #962, #26686, #8794, #16627, #29587, #18853, #16295, #27023, #6064, #11030, #29414, #3347, #8465, #6239, #13737, #31962, #24471, #24134, #24294, #14076, #26855, #11191, #801, #29249, #16458, #1132, #3516, #5901, #11362, #21570, #13909, #21742, #632, #32132, #21411, #19191, #15746, #26304, #31265, #18478, #3294, #23747, #31746, #29194, #18306, #21350, #412, #13678, #10649, #8094, #28698, #28861, #10973, #8416, #3134, #2809, #20864, #10815, #18802, #15907, #5358, #7926, #13190, #18145, #26141, #5846, #28543, #21188, #21024, #15574, #23589, #31585, #8250, #13354, #24076, #86, #2975, #31424, #23914, #256, #5517, #13521, #26465, #578, #18638, #16245, #25972, #29030, #5685, #16074, #745, #31096, #26632, #11145, #7755, #5189, #2647, #13030, #23422, #10485, #3459, #11803, #26965, #14020, #27305, #19134, #19643, #3803, #27473, #32409, #11475, #14192, #18973, #3966, #29528, #21853, #32581, #24419, #14521, #30032, #24922, #907, #29870, #21691, #8580, #29367, #6697, #1413, #8911, #6529, #22192, #1581, #6183, #27143, #4130, #16574, #26796, #11306, #32083, #13856, #21520, #14365, #19304, #24241, #9249, #6012, #16402, #17087, #8745, #31907, #3626, #1083, #24759, #32244, #29694, #6351, #22028, #24587, #16742, #16909, #1246, #11644, #9075, #19470, #24719, #27768, #4264, #1543, #4432, #9542, #17042, #14657, #19933, #9718, #3923, #11939, #12268, #1375, #1202, #9039, #29835, #11601, #1883, #1706, #27436, #21989, #30331, #14152, #24548, #14820, #19431, #22660, #17384, #32375, #4092, #33048, #29997, #6494, #6824, #16873, #11763, #22151, #29661, #25053, #6310, #16705, #14322, #24879, #27266, #14482, #27106, #22322, #6999, #25218, #32540, #3767, #32708, #9215, #19605, #6654, #9375, #19771, #30166, #17209, #12103, #27596, #22496, #32882, #10860, #4944, #7344, #30680, #2222, #7164, #17723, #21233, #17548, #10687, #10072, #4612, #28110, #21069, #31471, #2849, #13569, #22834, #15330, #33401, #13393, #15166, #4771, #3012, #15954, #23792, #30848, #461, #14995, #26180, #292, #20449, #3178, #20108, #25558, #13234, #16113, #12606, #28906, #23959, #7512, #25384, #2055, #31629, #23001, #17896, #26351, #28290, #18684, #23630, #26508, #8297, #12444, #8138, #621, #18523, #33226, #5562, #9890, #29074, #5724, #30501, #27942, #20273, #14410, #29406, #6228, #11182, #32122, #16955, #3673, #11690, #9125, #31953, #1299, #14066, #27350, #24280, #21734, #8622, #8786, #24634, #22072, #16787, #16448, #793, #24463, #32455, #29576, #19018, #21560, #26844, #31789, #6056, #19522, #8456, #1125, #953, #29239, #3508, #11518, #21899, #27012, #4016, #13723, #16617, #11351, #3843, #13900, #19181, #27188, #6405, #14235, #32296, #29918, #5890, #8957, #19347, #29740, #24803, #11021, #6571, #21400, #18844, #16287, #26676, #3338, #24123, #19685, #17133, #25473, #6910, #27690, #7256, #32795, #33312, #17466, #7422, #12359, #25128, #27851, #32630, #17640, #9465, #1791, #12531, #4353, #28204, #9982, #4863, #14573, #30250, #20370, #9812, #7084, #30764, #15077, #22580, #20191, #2146, #15251, #19853, #4523, #17807, #17303, #6743, #24973, #1627, #27519, #1459, #28026, #32965, #4177, #22920, #30079, #12017, #11855, #22403, #22241, #9291, #14738, #14913, #12192, #9628, #20025, #30426, #25304, #1968, #22755, #4691, #33148, #30590, #15914, #10150, #20531, #10821, #5032, #31591, #13360, #30937, #23429, #8256, #25981, #17983, #2815, #15422, #20702, #31101, #18645, #262, #29038, #5691, #10330, #20872, #25819, #13036, #25644, #18313, #26312, #23755, #12865, #2981, #28704, #2310, #5195, #2653, #23256, #92, #5523, #419, #31431, #7762, #2482, #5365, #21196, #10492, #33650, #18154, #28549, #12696, #15580, #23092, #33482, #15752, #31271, #7601, #7932, #26147, #13197, #23597, #28375, #10657, #21031, #8101, #18484, #28867, #13685, #32252, #11482, #19312, #26804, #8921, #10979, #11314, #29536, #29374, #32419, #16080, #26638, #8753, #11653, #752, #24427, #19480, #16410, #585, #31753, #6359, #21526, #8587, #21861, #24083, #14199, #32090, #29701, #16750, #27152, #3810, #16252, #16581, #19141, #29880, #1091, #26472, #24248, #24595, #3634, #1256, #21357, #22036, #9084, #6193, #8422, #11151, #18808, #3300, #31915, #18982, #6019, #3142, #3468, #13528, #23920, #26972, #13863, #29201, #915, #14028, #5853, #21699, #33273 ),
 ( #2107, #24932, #14869, #9941, #6871, #24767, #22202, #30550, #11981, #32755, #12318, #4139, #7212, #20152, #22366, #22546, #30214, #32930, #3975, #22713, #14531, #17259, #17599, #9426, #20325, #15040, #6537, #19652, #1591, #4656, #25266, #12150, #25432, #27990, #27647, #1931, #12493, #16917, #19820, #9589, #22882, #4316, #11814, #30042, #6707, #32592, #27313, #33102, #14701, #9258, #14376, #1422, #17099, #27483, #25093, #1751, #19984, #30385, #7046, #17429, #27813, #4480, #9770, #10116, #25776, #2447, #2943, #5324, #13326, #379, #15382, #25939, #30898, #18111, #23718, #23394, #31392, #28834, #17949, #20995, #58, #10782, #10292, #7725, #28339, #28507, #10621, #8062, #2783, #12827, #20495, #10454, #18446, #15547, #2614, #20828, #20672, #30727, #7386, #7563, #31233, #26274, #23218, #15714, #17767, #31067, #15214, #12653, #5491, #33614, #5159, #13163, #4995, #15880, #28164, #13000, #7895, #18276, #28665, #4821, #23554, #26115, #225, #25606, #2271, #23051, #33445, #14158, #552, #16209, #19273, #29494, #26764, #29666, #1052, #8543, #6148, #11443, #1211, #29159, #3427, #3774, #26598, #26435, #10945, #21320, #3100, #27112, #26938, #18938, #13488, #21822, #5657, #16044, #6316, #31716, #24554, #8876, #23881, #29335, #21158, #21493, #8388, #32052, #18776, #3262, #13651, #31555, #16542, #8222, #18611, #5812, #16370, #24044, #5981, #28997, #13823, #32212, #16710, #712, #11115, #24215, #31877, #878, #11275, #21656, #8715, #19105, #3596, #13990, #24386, #1380, #14663, #1889, #30172, #32546, #22158, #27444, #32381, #9221, #12274, #9044, #1711, #1548, #29840, #19610, #12110, #22501, #27602, #4618, #14329, #6830, #24887, #4438, #6661, #30002, #27773, #7004, #14827, #22327, #25224, #6500, #22666, #17048, #33055, #16878, #30338, #27273, #9723, #4097, #11606, #3931, #14487, #17214, #11946, #25057, #20114, #24724, #21996, #11768, #30506, #32715, #7171, #9382, #19776, #9548, #4270, #17556, #27948, #15000, #32888, #19940, #25388, #17390, #19436, #12787, #10077, #7349, #26074, #20455, #23177, #28795, #2228, #23352, #20954, #28460, #4950, #30853, #15, #10249, #2061, #28115, #7682, #5449, #15672, #7518, #4776, #5117, #13118, #33568, #20625, #33405, #10410, #25730, #18236, #17902, #12450, #25564, #178, #28296, #18064, #9897, #2744, #17729, #15336, #28625, #7851, #5278, #23509, #12611, #2568, #15508, #15836, #20783, #22839, #31025, #10577, #31183, #31348, #20280, #8016, #18401, #25898, #15171, #2401, #23008, #12957, #33231, #30686, #26395, #10734, #8828, #31674, #666, #11400, #5936, #16328, #333, #24003, #11224, #13945, #8499, #21609, #11069, #835, #26720, #3054, #31833, #21116, #3382, #6273, #13281, #24334, #10902, #31515, #18733, #16003, #3553, #5612, #24173, #18890, #21778, #21280, #32003, #29625, #26550, #8183, #18568, #16496, #8344, #29118, #8668, #23836, #26895, #6099, #5766, #29285, #16160, #13777, #23674, #19059, #510, #3221, #1005, #13607, #19230, #32167, #26225, #13441, #21450, #2895, #29449, #28953, #25175, #30291, #4057, #1671, #6958, #30468, #24680, #22289, #33008, #11729, #21950, #29792, #16836, #32339, #22620, #22450, #14448, #9003, #17348, #1166, #11561, #1844, #6456, #9677, #4397, #19393, #24842, #20071, #17001, #27231, #27558, #3885, #22116, #32503, #16666, #25016, #27062, #3725, #1342, #11902, #14279, #1505, #14115, #9337, #27735, #14783, #9177, #12233, #19730, #24508, #29960, #27395, #19567, #32671, #6616, #30127, #32843, #6786, #17172, #4222, #14621, #12062, #9506, #19893, #22964, #27900, #17685, #7806, #4573, #30986, #30808, #25346, #28072, #7642, #18025, #23138, #136, #9855, #25687, #20415, #26061, #2188, #4735, #23305, #2526, #10371, #17855, #20744, #2015, #2356, #20582, #7470, #23470, #7128, #15124, #10538, #7309, #28417, #26032, #33527, #10036, #25520, #5074, #15292, #17510, #33191, #12748, #20918, #31140, #12572, #20237, #10200, #18198, #4907, #28252, #33362, #15471, #25861, #28589, #12910, #14959, #30639, #5240, #15628, #2703, #12404, #13080, #22800, #26358, #13731, #3343, #24131, #798, #31477, #31795, #23965, #959, #16292, #31312, #5730, #11187, #18849, #8628, #15796, #21566, #31959, #628, #13241, #3017, #23638, #8145, #16120, #31634, #18528, #26187, #13905, #13401, #26513, #16453, #11026, #21408, #5411, #29082, #26682, #19023, #13574, #29411, #3183, #5897, #8462, #28911, #29246, #2856, #6061, #11357, #18361, #26851, #15963, #297, #23797, #21075, #3513, #10696, #24289, #7977, #5569, #28752, #468, #10865, #21240, #8301, #18692, #21739, #6234, #8962, #17432, #1756, #1934, #15044, #24468, #32129, #21904, #12496, #16624, #17771, #9593, #19987, #20156, #19353, #25436, #20330, #22885, #3679, #32301, #30730, #27816, #8791, #32934, #29748, #27018, #33277, #6411, #30388, #19187, #12323, #12155, #14071, #16793, #22717, #33107, #4484, #15218, #1129, #7051, #22549, #2112, #27192, #3848, #4660, #17603, #9944, #14875, #7390, #11523, #25269, #9773, #30554, #4827, #29582, #14240, #7216, #28168, #24638, #27994, #25609, #2274, #30901, #28343, #2949, #18115, #5163, #18451, #10298, #13330, #26278, #28513, #28669, #2617, #5327, #10119, #28838, #20674, #13005, #23721, #15550, #5661, #21161, #16049, #25783, #7729, #10786, #20999, #18280, #31558, #384, #61, #31397, #8225, #26439, #31071, #15719, #29001, #25943, #17953, #2450, #12830, #4998, #18614, #5494, #10458, #15386, #12658, #7567, #23222, #23056, #33617, #33448, #20500, #23398, #20833 ) ),
 .UNSPECIFIED., .T., .F., .T. ) 
 B_SPLINE_SURFACE_WITH_KNOTS ( ( 4, 3, 4 ),
 ( 3, 2, 2, 2, 2, 2, 2, 2, 2, 2, 2, 2, 2, 2, 2, 2, 2, 2, 2, 2, 2, 2, 2, 2, 2, 2, 2, 2, 2, 2, 2, 2, 2, 2, 2, 2, 2, 2, 2, 2, 2, 2, 2, 2, 2, 2, 2, 2, 2, 2, 2, 2, 2, 2, 2, 2, 2, 2, 2, 2, 2, 2, 2, 2, 2, 2, 2, 2, 2, 2, 2, 2, 2, 2, 2, 2, 2, 2, 2, 2, 2, 2, 2, 2, 2, 2, 2, 2, 2, 2, 2, 2, 2, 2, 2, 2, 2, 2, 2, 2, 2, 2, 2, 2, 2, 2, 2, 2, 2, 2, 2, 2, 2, 2, 2, 2, 2, 2, 2, 2, 2, 2, 2, 2, 2, 2, 2, 2, 2, 2, 2, 2, 2, 2, 2, 2, 2, 2, 2, 2, 2, 2, 2, 2, 2, 2, 2, 2, 2, 2, 2, 2, 2, 2, 2, 2, 2, 2, 2, 2, 2, 2, 2, 2, 2, 2, 2, 2, 2, 2, 2, 2, 2, 2, 2, 2, 2, 2, 2, 2, 2, 2, 2, 2, 2, 2, 2, 2, 2, 2, 2, 2, 2, 2, 2, 2, 2, 2, 2, 2, 2, 2, 2, 2, 2, 2, 2, 2, 2, 2, 2, 2, 2, 2, 2, 2, 2, 2, 2, 2, 2, 2, 2, 2, 2, 2, 2, 2, 2, 2, 2, 2, 2, 2, 2, 2, 2, 2, 2, 2, 2, 2, 2, 2, 2, 2, 2, 2, 2, 2, 2, 2, 2, 2, 2, 2, 2, 2, 2, 2, 2, 2, 2, 2, 2, 2, 2, 2, 2, 2, 2, 2, 2, 2, 2, 2, 2, 2, 2, 2, 2, 2, 2, 2, 2, 2, 2, 2, 2, 2, 2, 2, 2, 2, 2, 2, 2, 2, 2, 2, 2, 2, 2, 2, 2, 2, 2, 2, 2, 2, 2, 2, 2, 2, 2, 2, 2, 2, 2, 2, 2, 2, 2, 2, 2, 2, 2, 2, 2, 2, 2, 2, 2, 2, 2, 2, 2, 2, 2, 2, 2, 2, 2, 2, 2, 2, 3 ),
 ( 0.000000000000000000, 0.5000000000000000000, 1.000000000000000000 ),
 ( 0.000000000000000000, 0.002857142857142857140, 0.005714285714285714281, 0.008571428571428571855, 0.01142857142857142856, 0.01428571428571428527, 0.01714285714285714371, 0.02000000000000000042, 0.02285714285714285712, 0.02571428571428571383, 0.02857142857142857054, 0.03142857142857143071, 0.03428571428571428742, 0.03714285714285714413, 0.04000000000000000083, 0.04285714285714285754, 0.04571428571428571425, 0.04857142857142857095, 0.05142857142857142766, 0.05428571428571428437, 0.05714285714285714107, 0.05999999999999999778, 0.06285714285714286143, 0.06571428571428571119, 0.06857142857142857484, 0.07142857142857142461, 0.07428571428571428825, 0.07714285714285713802, 0.08000000000000000167, 0.08285714285714285143, 0.08571428571428571508, 0.08857142857142856485, 0.09142857142857142849, 0.09428571428571429214, 0.09714285714285714191, 0.1000000000000000056, 0.1028571428571428553, 0.1057142857142857190, 0.1085714285714285687, 0.1114285714285714324, 0.1142857142857142821, 0.1171428571428571458, 0.1199999999999999956, 0.1228571428571428592, 0.1257142857142857229, 0.1285714285714285587, 0.1314285714285714224, 0.1342857142857142860, 0.1371428571428571497, 0.1400000000000000133, 0.1428571428571428492, 0.1457142857142857129, 0.1485714285714285765, 0.1514285714285714401, 0.1542857142857142760, 0.1571428571428571397, 0.1600000000000000033, 0.1628571428571428670, 0.1657142857142857029, 0.1685714285714285665, 0.1714285714285714302, 0.1742857142857142938, 0.1771428571428571297, 0.1799999999999999933, 0.1828571428571428570, 0.1857142857142857206, 0.1885714285714285843, 0.1914285714285714202, 0.1942857142857142838, 0.1971428571428571475, 0.2000000000000000111, 0.2028571428571428470, 0.2057142857142857106, 0.2085714285714285743, 0.2114285714285714379, 0.2142857142857142738, 0.2171428571428571375, 0.2200000000000000011, 0.2228571428571428648, 0.2257142857142857006, 0.2285714285714285643, 0.2314285714285714279, 0.2342857142857142916, 0.2371428571428571552, 0.2399999999999999911, 0.2428571428571428548, 0.2457142857142857184, 0.2485714285714285821, 0.2514285714285714457, 0.2542857142857142816, 0.2571428571428571175, 0.2600000000000000089, 0.2628571428571428448, 0.2657142857142857362, 0.2685714285714285721, 0.2714285714285714080, 0.2742857142857142994, 0.2771428571428571352, 0.2800000000000000266, 0.2828571428571428625, 0.2857142857142856984, 0.2885714285714285898, 0.2914285714285714257, 0.2942857142857142616, 0.2971428571428571530, 0.2999999999999999889, 0.3028571428571428803, 0.3057142857142857162, 0.3085714285714285521, 0.3114285714285714435, 0.3142857142857142794, 0.3171428571428571153, 0.3200000000000000067, 0.3228571428571428426, 0.3257142857142857340, 0.3285714285714285698, 0.3314285714285714057, 0.3342857142857142971, 0.3371428571428571330, 0.3400000000000000244, 0.3428571428571428603, 0.3457142857142856962, 0.3485714285714285876, 0.3514285714285714235, 0.3542857142857142594, 0.3571428571428571508, 0.3599999999999999867, 0.3628571428571428781, 0.3657142857142857140, 0.3685714285714285499, 0.3714285714285714413, 0.3742857142857142771, 0.3771428571428571686, 0.3800000000000000044, 0.3828571428571428403, 0.3857142857142857317, 0.3885714285714285676, 0.3914285714285714035, 0.3942857142857142949, 0.3971428571428571308, 0.4000000000000000222, 0.4028571428571428581, 0.4057142857142856940, 0.4085714285714285854, 0.4114285714285714213, 0.4142857142857143127, 0.4171428571428571486, 0.4199999999999999845, 0.4228571428571428759, 0.4257142857142857117, 0.4285714285714285476, 0.4314285714285714390, 0.4342857142857142749, 0.4371428571428571663, 0.4400000000000000022, 0.4428571428571428381, 0.4457142857142857295, 0.4485714285714285654, 0.4514285714285714013, 0.4542857142857142927, 0.4571428571428571286, 0.4600000000000000200, 0.4628571428571428559, 0.4657142857142856918, 0.4685714285714285832, 0.4714285714285714191, 0.4742857142857143105, 0.4771428571428571463, 0.4799999999999999822, 0.4828571428571428736, 0.4857142857142857095, 0.4885714285714285454, 0.4914285714285714368, 0.4942857142857142727, 0.4971428571428571641, 0.5000000000000000000, 0.5028571428571428914, 0.5057142857142856718, 0.5085714285714285632, 0.5114285714285714546, 0.5142857142857142350, 0.5171428571428571264, 0.5200000000000000178, 0.5228571428571429092, 0.5257142857142856895, 0.5285714285714285809, 0.5314285714285714723, 0.5342857142857142527, 0.5371428571428571441, 0.5400000000000000355, 0.5428571428571428159, 0.5457142857142857073, 0.5485714285714285987, 0.5514285714285713791, 0.5542857142857142705, 0.5571428571428571619, 0.5600000000000000533, 0.5628571428571428337, 0.5657142857142857251, 0.5685714285714286165, 0.5714285714285713969, 0.5742857142857142883, 0.5771428571428571797, 0.5799999999999999600, 0.5828571428571428514, 0.5857142857142857428, 0.5885714285714285232, 0.5914285714285714146, 0.5942857142857143060, 0.5971428571428571974, 0.5999999999999999778, 0.6028571428571428692, 0.6057142857142857606, 0.6085714285714285410, 0.6114285714285714324, 0.6142857142857143238, 0.6171428571428571042, 0.6199999999999999956, 0.6228571428571428870, 0.6257142857142856673, 0.6285714285714285587, 0.6314285714285714501, 0.6342857142857142305, 0.6371428571428571219, 0.6400000000000000133, 0.6428571428571429047, 0.6457142857142856851, 0.6485714285714285765, 0.6514285714285714679, 0.6542857142857142483, 0.6571428571428571397, 0.6600000000000000311, 0.6628571428571428115, 0.6657142857142857029, 0.6685714285714285943, 0.6714285714285713746, 0.6742857142857142660, 0.6771428571428571574, 0.6800000000000000488, 0.6828571428571428292, 0.6857142857142857206, 0.6885714285714286120, 0.6914285714285713924, 0.6942857142857142838, 0.6971428571428571752, 0.6999999999999999556, 0.7028571428571428470, 0.7057142857142857384, 0.7085714285714285188, 0.7114285714285714102, 0.7142857142857143016, 0.7171428571428571930, 0.7199999999999999734, 0.7228571428571428648, 0.7257142857142857562, 0.7285714285714285365, 0.7314285714285714279, 0.7342857142857143193, 0.7371428571428570997, 0.7399999999999999911, 0.7428571428571428825, 0.7457142857142856629, 0.7485714285714285543, 0.7514285714285714457, 0.7542857142857143371, 0.7571428571428571175, 0.7600000000000000089, 0.7628571428571429003, 0.7657142857142856807, 0.7685714285714285721, 0.7714285714285714635, 0.7742857142857142438, 0.7771428571428571352, 0.7800000000000000266, 0.7828571428571428070, 0.7857142857142856984, 0.7885714285714285898, 0.7914285714285714812, 0.7942857142857142616, 0.7971428571428571530, 0.8000000000000000444, 0.8028571428571428248, 0.8057142857142857162, 0.8085714285714286076, 0.8114285714285713880, 0.8142857142857142794, 0.8171428571428571708, 0.8199999999999999512, 0.8228571428571428426, 0.8257142857142857340, 0.8285714285714286254, 0.8314285714285714057, 0.8342857142857142971, 0.8371428571428571885, 0.8399999999999999689, 0.8428571428571428603, 0.8457142857142857517, 0.8485714285714285321, 0.8514285714285714235, 0.8542857142857143149, 0.8571428571428570953, 0.8599999999999999867, 0.8628571428571428781, 0.8657142857142857695, 0.8685714285714285499, 0.8714285714285714413, 0.8742857142857143327, 0.8771428571428571130, 0.8800000000000000044, 0.8828571428571428958, 0.8857142857142856762, 0.8885714285714285676, 0.8914285714285714590, 0.8942857142857142394, 0.8971428571428571308, 0.9000000000000000222, 0.9028571428571428026, 0.9057142857142856940, 0.9085714285714285854, 0.9114285714285714768, 0.9142857142857142572, 0.9171428571428571486, 0.9200000000000000400, 0.9228571428571428203, 0.9257142857142857117, 0.9285714285714286031, 0.9314285714285713835, 0.9342857142857142749, 0.9371428571428571663, 0.9399999999999999467, 0.9428571428571428381, 0.9457142857142857295, 0.9485714285714286209, 0.9514285714285714013, 0.9542857142857142927, 0.9571428571428571841, 0.9599999999999999645, 0.9628571428571428559, 0.9657142857142857473, 0.9685714285714285277, 0.9714285714285714191, 0.9742857142857143105, 0.9771428571428570908, 0.9799999999999999822, 0.9828571428571428736, 0.9857142857142857650, 0.9955714285714286627 ),
 .UNSPECIFIED. ) 
 GEOMETRIC_REPRESENTATION_ITEM ( )  RATIONAL_B_SPLINE_SURFACE ( (
 ( 1.000000000000000000, 0.9510565162951535312, 1.000000000000000000, 0.9510565162951535312, 1.000000000000000000, 0.9510565162951535312, 1.000000000000000000, 0.9510565162951535312, 1.000000000000000000, 0.9510565162951535312, 1.000000000000000000, 0.9510565162951535312, 1.000000000000000000, 0.9510565162951535312, 1.000000000000000000, 0.9510565162951535312, 1.000000000000000000, 0.9510565162951535312, 1.000000000000000000, 0.9510565162951535312, 1.000000000000000000, 0.9510565162951535312, 1.000000000000000000, 0.9510565162951535312, 1.000000000000000000, 0.9510565162951535312, 1.000000000000000000, 0.9510565162951535312, 1.000000000000000000, 0.9510565162951535312, 1.000000000000000000, 0.9510565162951535312, 1.000000000000000000, 0.9510565162951535312, 1.000000000000000000, 0.9510565162951535312, 1.000000000000000000, 0.9510565162951535312, 1.000000000000000000, 0.9510565162951535312, 1.000000000000000000, 0.9510565162951535312, 1.000000000000000000, 0.9510565162951535312, 1.000000000000000000, 0.9510565162951535312, 1.000000000000000000, 0.9510565162951535312, 1.000000000000000000, 0.9510565162951535312, 1.000000000000000000, 0.9510565162951535312, 1.000000000000000000, 0.9510565162951535312, 1.000000000000000000, 0.9510565162951535312, 1.000000000000000000, 0.9510565162951535312, 1.000000000000000000, 0.9510565162951535312, 1.000000000000000000, 0.9510565162951535312, 1.000000000000000000, 0.9510565162951535312, 1.000000000000000000, 0.9510565162951535312, 1.000000000000000000, 0.9510565162951535312, 1.000000000000000000, 0.9510565162951535312, 1.000000000000000000, 0.9510565162951535312, 1.000000000000000000, 0.9510565162951535312, 1.000000000000000000, 0.9510565162951535312, 1.000000000000000000, 0.9510565162951535312, 1.000000000000000000, 0.9510565162951535312, 1.000000000000000000, 0.9510565162951535312, 1.000000000000000000, 0.9510565162951535312, 1.000000000000000000, 0.9510565162951535312, 1.000000000000000000, 0.9510565162951535312, 1.000000000000000000, 0.9510565162951535312, 1.000000000000000000, 0.9510565162951535312, 1.000000000000000000, 0.9510565162951535312, 1.000000000000000000, 0.9510565162951535312, 1.000000000000000000, 0.9510565162951535312, 1.000000000000000000, 0.9510565162951535312, 1.000000000000000000, 0.9510565162951535312, 1.000000000000000000, 0.9510565162951535312, 1.000000000000000000, 0.9510565162951535312, 1.000000000000000000, 0.9510565162951535312, 1.000000000000000000, 0.9510565162951535312, 1.000000000000000000, 0.9510565162951535312, 1.000000000000000000, 0.9510565162951535312, 1.000000000000000000, 0.9510565162951535312, 1.000000000000000000, 0.9510565162951535312, 1.000000000000000000, 0.9510565162951535312, 1.000000000000000000, 0.9510565162951535312, 1.000000000000000000, 0.9510565162951535312, 1.000000000000000000, 0.9510565162951535312, 1.000000000000000000, 0.9510565162951535312, 1.000000000000000000, 0.9510565162951535312, 1.000000000000000000, 0.9510565162951535312, 1.000000000000000000, 0.9510565162951535312, 1.000000000000000000, 0.9510565162951535312, 1.000000000000000000, 0.9510565162951535312, 1.000000000000000000, 0.9510565162951535312, 1.000000000000000000, 0.9510565162951535312, 1.000000000000000000, 0.9510565162951535312, 1.000000000000000000, 0.9510565162951535312, 1.000000000000000000, 0.9510565162951535312, 1.000000000000000000, 0.9510565162951535312, 1.000000000000000000, 0.9510565162951535312, 1.000000000000000000, 0.9510565162951535312, 1.000000000000000000, 0.9510565162951535312, 1.000000000000000000, 0.9510565162951535312, 1.000000000000000000, 0.9510565162951535312, 1.000000000000000000, 0.9510565162951535312, 1.000000000000000000, 0.9510565162951535312, 1.000000000000000000, 0.9510565162951535312, 1.000000000000000000, 0.9510565162951535312, 1.000000000000000000, 0.9510565162951535312, 1.000000000000000000, 0.9510565162951535312, 1.000000000000000000, 0.9510565162951535312, 1.000000000000000000, 0.9510565162951535312, 1.000000000000000000, 0.9510565162951535312, 1.000000000000000000, 0.9510565162951535312, 1.000000000000000000, 0.9510565162951535312, 1.000000000000000000, 0.9510565162951535312, 1.000000000000000000, 0.9510565162951535312, 1.000000000000000000, 0.9510565162951535312, 1.000000000000000000, 0.9510565162951535312, 1.000000000000000000, 0.9510565162951535312, 1.000000000000000000, 0.9510565162951535312, 1.000000000000000000, 0.9510565162951535312, 1.000000000000000000, 0.9510565162951535312, 1.000000000000000000, 0.9510565162951535312, 1.000000000000000000, 0.9510565162951535312, 1.000000000000000000, 0.9510565162951535312, 1.000000000000000000, 0.9510565162951535312, 1.000000000000000000, 0.9510565162951535312, 1.000000000000000000, 0.9510565162951535312, 1.000000000000000000, 0.9510565162951535312, 1.000000000000000000, 0.9510565162951535312, 1.000000000000000000, 0.9510565162951535312, 1.000000000000000000, 0.9510565162951535312, 1.000000000000000000, 0.9510565162951535312, 1.000000000000000000, 0.9510565162951535312, 1.000000000000000000, 0.9510565162951535312, 1.000000000000000000, 0.9510565162951535312, 1.000000000000000000, 0.9510565162951535312, 1.000000000000000000, 0.9510565162951535312, 1.000000000000000000, 0.9510565162951535312, 1.000000000000000000, 0.9510565162951535312, 1.000000000000000000, 0.9510565162951535312, 1.000000000000000000, 0.9510565162951535312, 1.000000000000000000, 0.9510565162951535312, 1.000000000000000000, 0.9510565162951535312, 1.000000000000000000, 0.9510565162951535312, 1.000000000000000000, 0.9510565162951535312, 1.000000000000000000, 0.9510565162951535312, 1.000000000000000000, 0.9510565162951535312, 1.000000000000000000, 0.9510565162951535312, 1.000000000000000000, 0.9510565162951535312, 1.000000000000000000, 0.9510565162951535312, 1.000000000000000000, 0.9510565162951535312, 1.000000000000000000, 0.9510565162951535312, 1.000000000000000000, 0.9510565162951535312, 1.000000000000000000, 0.9510565162951535312, 1.000000000000000000, 0.9510565162951535312, 1.000000000000000000, 0.9510565162951535312, 1.000000000000000000, 0.9510565162951535312, 1.000000000000000000, 0.9510565162951535312, 1.000000000000000000, 0.9510565162951535312, 1.000000000000000000, 0.9510565162951535312, 1.000000000000000000, 0.9510565162951535312, 1.000000000000000000, 0.9510565162951535312, 1.000000000000000000, 0.9510565162951535312, 1.000000000000000000, 0.9510565162951535312, 1.000000000000000000, 0.9510565162951535312, 1.000000000000000000, 0.9510565162951535312, 1.000000000000000000, 0.9510565162951535312, 1.000000000000000000, 0.9510565162951535312, 1.000000000000000000, 0.9510565162951535312, 1.000000000000000000, 0.9510565162951535312, 1.000000000000000000, 0.9510565162951535312, 1.000000000000000000, 0.9510565162951535312, 1.000000000000000000, 0.9510565162951535312, 1.000000000000000000, 0.9510565162951535312, 1.000000000000000000, 0.9510565162951535312, 1.000000000000000000, 0.9510565162951535312, 1.000000000000000000, 0.9510565162951535312, 1.000000000000000000, 0.9510565162951535312, 1.000000000000000000, 0.9510565162951535312, 1.000000000000000000, 0.9510565162951535312, 1.000000000000000000, 0.9510565162951535312, 1.000000000000000000, 0.9510565162951535312, 1.000000000000000000, 0.9510565162951535312, 1.000000000000000000, 0.9510565162951535312, 1.000000000000000000, 0.9510565162951535312, 1.000000000000000000, 0.9510565162951535312, 1.000000000000000000, 0.9510565162951535312, 1.000000000000000000, 0.9510565162951535312, 1.000000000000000000, 0.9510565162951535312, 1.000000000000000000, 0.9510565162951535312, 1.000000000000000000, 0.9510565162951535312, 1.000000000000000000, 0.9510565162951535312, 1.000000000000000000, 0.9510565162951535312, 1.000000000000000000, 0.9510565162951535312, 1.000000000000000000, 0.9510565162951535312, 1.000000000000000000, 0.9510565162951535312, 1.000000000000000000, 0.9510565162951535312, 1.000000000000000000, 0.9510565162951535312, 1.000000000000000000, 0.9510565162951535312, 1.000000000000000000, 0.9510565162951535312, 1.000000000000000000, 0.9510565162951535312, 1.000000000000000000, 0.9510565162951535312, 1.000000000000000000, 0.9510565162951535312, 1.000000000000000000, 0.9510565162951535312, 1.000000000000000000, 0.9510565162951535312, 1.000000000000000000, 0.9510565162951535312, 1.000000000000000000, 0.9510565162951535312, 1.000000000000000000, 0.9510565162951535312, 1.000000000000000000, 0.9510565162951535312, 1.000000000000000000, 0.9510565162951535312, 1.000000000000000000, 0.9510565162951535312, 1.000000000000000000, 0.9510565162951535312, 1.000000000000000000, 0.9510565162951535312, 1.000000000000000000, 0.9510565162951535312, 1.000000000000000000, 0.9510565162951535312, 1.000000000000000000, 0.9510565162951535312, 1.000000000000000000, 0.9510565162951535312, 1.000000000000000000, 0.9510565162951535312, 1.000000000000000000, 0.9510565162951535312, 1.000000000000000000, 0.9510565162951535312, 1.000000000000000000, 0.9510565162951535312, 1.000000000000000000, 0.9510565162951535312, 1.000000000000000000, 0.9510565162951535312, 1.000000000000000000, 0.9510565162951535312, 1.000000000000000000, 0.9510565162951535312, 1.000000000000000000, 0.9510565162951535312, 1.000000000000000000, 0.9510565162951535312, 1.000000000000000000, 0.9510565162951535312, 1.000000000000000000, 0.9510565162951535312, 1.000000000000000000, 0.9510565162951535312, 1.000000000000000000, 0.9510565162951535312, 1.000000000000000000, 0.9510565162951535312, 1.000000000000000000, 0.9510565162951535312, 1.000000000000000000, 0.9510565162951535312, 1.000000000000000000, 0.9510565162951535312, 1.000000000000000000, 0.9510565162951535312, 1.000000000000000000, 0.9510565162951535312, 1.000000000000000000, 0.9510565162951535312, 1.000000000000000000, 0.9510565162951535312, 1.000000000000000000, 0.9510565162951535312, 1.000000000000000000, 0.9510565162951535312, 1.000000000000000000, 0.9510565162951535312, 1.000000000000000000, 0.9510565162951535312, 1.000000000000000000, 0.9510565162951535312, 1.000000000000000000, 0.9510565162951535312, 1.000000000000000000, 0.9510565162951535312, 1.000000000000000000, 0.9510565162951535312, 1.000000000000000000, 0.9510565162951535312, 1.000000000000000000, 0.9510565162951535312, 1.000000000000000000, 0.9510565162951535312, 1.000000000000000000, 0.9510565162951535312, 1.000000000000000000, 0.9510565162951535312, 1.000000000000000000, 0.9510565162951535312, 1.000000000000000000, 0.9510565162951535312, 1.000000000000000000, 0.9510565162951535312, 1.000000000000000000, 0.9510565162951535312, 1.000000000000000000, 0.9510565162951535312, 1.000000000000000000, 0.9510565162951535312, 1.000000000000000000, 0.9510565162951535312, 1.000000000000000000, 0.9510565162951535312, 1.000000000000000000, 0.9510565162951535312, 1.000000000000000000, 0.9510565162951535312, 1.000000000000000000, 0.9510565162951535312, 1.000000000000000000, 0.9510565162951535312, 1.000000000000000000, 0.9510565162951535312, 1.000000000000000000, 0.9510565162951535312, 1.000000000000000000, 0.9510565162951535312, 1.000000000000000000, 0.9510565162951535312, 1.000000000000000000, 0.9510565162951535312, 1.000000000000000000, 0.9510565162951535312, 1.000000000000000000, 0.9510565162951535312, 1.000000000000000000, 0.9510565162951535312, 1.000000000000000000, 0.9510565162951535312, 1.000000000000000000, 0.9510565162951535312, 1.000000000000000000, 0.9510565162951535312, 1.000000000000000000, 0.9510565162951535312, 1.000000000000000000, 0.9510565162951535312, 1.000000000000000000, 0.9510565162951535312, 1.000000000000000000, 0.9510565162951535312, 1.000000000000000000, 0.9510565162951535312, 1.000000000000000000, 0.9510565162951535312, 1.000000000000000000, 0.9510565162951535312, 1.000000000000000000, 0.9510565162951535312, 1.000000000000000000, 0.9510565162951535312, 1.000000000000000000, 0.9510565162951535312, 1.000000000000000000, 0.9510565162951535312, 1.000000000000000000, 0.9510565162951535312, 1.000000000000000000, 0.9510565162951535312, 1.000000000000000000, 0.9510565162951535312, 1.000000000000000000, 0.9510565162951535312, 1.000000000000000000, 0.9510565162951535312, 1.000000000000000000, 0.9510565162951535312, 1.000000000000000000, 0.9510565162951535312, 1.000000000000000000, 0.9510565162951535312, 1.000000000000000000, 0.9510565162951535312, 1.000000000000000000, 0.9510565162951535312, 1.000000000000000000, 0.9510565162951535312, 1.000000000000000000, 0.9510565162951535312, 1.000000000000000000, 0.9510565162951535312, 1.000000000000000000, 0.9510565162951535312, 1.000000000000000000, 0.9510565162951535312, 1.000000000000000000, 0.9510565162951535312, 1.000000000000000000, 0.9510565162951535312, 1.000000000000000000, 0.9510565162951535312, 1.000000000000000000, 0.9510565162951535312, 1.000000000000000000, 0.9510565162951535312, 1.000000000000000000, 0.9510565162951535312, 1.000000000000000000, 0.9510565162951535312, 1.000000000000000000, 0.9510565162951535312, 1.000000000000000000, 0.9510565162951535312, 1.000000000000000000, 0.9510565162951535312, 1.000000000000000000, 0.9510565162951535312, 1.000000000000000000, 0.9510565162951535312, 1.000000000000000000, 0.9510565162951535312, 1.000000000000000000, 0.9510565162951535312, 1.000000000000000000, 0.9510565162951535312, 1.000000000000000000, 0.9510565162951535312, 1.000000000000000000, 0.9510565162951535312, 1.000000000000000000, 0.9510565162951535312, 1.000000000000000000, 0.9510565162951535312, 1.000000000000000000, 0.9510565162951535312, 1.000000000000000000, 0.9510565162951535312, 1.000000000000000000, 0.9510565162951535312, 1.000000000000000000, 0.9510565162951535312, 1.000000000000000000, 0.9510565162951535312, 1.000000000000000000, 0.9510565162951535312, 1.000000000000000000, 0.9510565162951535312, 1.000000000000000000, 0.9510565162951535312, 1.000000000000000000, 0.9510565162951535312, 1.000000000000000000, 0.9510565162951535312, 1.000000000000000000, 0.9510565162951535312, 1.000000000000000000, 0.9510565162951535312, 1.000000000000000000, 0.9510565162951535312, 1.000000000000000000, 0.9510565162951535312, 1.000000000000000000, 0.9510565162951535312, 1.000000000000000000, 0.9510565162951535312, 1.000000000000000000, 0.9510565162951535312, 1.000000000000000000, 0.9510565162951535312, 1.000000000000000000, 0.9510565162951535312, 1.000000000000000000, 0.9510565162951535312, 1.000000000000000000, 0.9510565162951535312, 1.000000000000000000, 0.9510565162951535312, 1.000000000000000000, 0.9510565162951535312, 1.000000000000000000, 0.9510565162951535312, 1.000000000000000000, 0.9510565162951535312, 1.000000000000000000, 0.9510565162951535312, 1.000000000000000000, 0.9510565162951535312, 1.000000000000000000, 0.9510565162951535312, 1.000000000000000000, 0.9510565162951535312, 1.000000000000000000, 0.9510565162951535312, 1.000000000000000000, 0.9510565162951535312, 1.000000000000000000, 0.9510565162951535312, 1.000000000000000000, 0.9510565162951535312, 1.000000000000000000, 0.9510565162951535312, 1.000000000000000000, 0.9510565162951535312, 1.000000000000000000, 0.9510565162951535312, 1.000000000000000000, 0.9510565162951535312, 1.000000000000000000, 0.9510565162951535312, 1.000000000000000000, 0.9510565162951535312, 1.000000000000000000, 0.9510565162951535312, 1.000000000000000000, 0.9510565162951535312, 1.000000000000000000, 0.9510565162951535312, 1.000000000000000000, 0.9510565162951535312, 1.000000000000000000, 0.9510565162951535312, 1.000000000000000000, 0.9510565162951535312, 1.000000000000000000, 0.9510565162951535312, 1.000000000000000000, 0.9510565162951535312, 1.000000000000000000, 1.000000000000000000, 1.000000000000000000),
 ( 0.3333333333333333703, 0.3170188387650512141, 0.3333333333333333703, 0.3170188387650512141, 0.3333333333333333703, 0.3170188387650512141, 0.3333333333333333703, 0.3170188387650512141, 0.3333333333333333703, 0.3170188387650512141, 0.3333333333333333703, 0.3170188387650512141, 0.3333333333333333703, 0.3170188387650512141, 0.3333333333333333703, 0.3170188387650512141, 0.3333333333333333703, 0.3170188387650512141, 0.3333333333333333703, 0.3170188387650512141, 0.3333333333333333703, 0.3170188387650512141, 0.3333333333333333703, 0.3170188387650512141, 0.3333333333333333703, 0.3170188387650512141, 0.3333333333333333703, 0.3170188387650512141, 0.3333333333333333703, 0.3170188387650512141, 0.3333333333333333703, 0.3170188387650512141, 0.3333333333333333703, 0.3170188387650512141, 0.3333333333333333703, 0.3170188387650512141, 0.3333333333333333703, 0.3170188387650512141, 0.3333333333333333703, 0.3170188387650512141, 0.3333333333333333703, 0.3170188387650512141, 0.3333333333333333703, 0.3170188387650512141, 0.3333333333333333703, 0.3170188387650512141, 0.3333333333333333703, 0.3170188387650512141, 0.3333333333333333703, 0.3170188387650512141, 0.3333333333333333703, 0.3170188387650512141, 0.3333333333333333703, 0.3170188387650512141, 0.3333333333333333703, 0.3170188387650512141, 0.3333333333333333703, 0.3170188387650512141, 0.3333333333333333703, 0.3170188387650512141, 0.3333333333333333703, 0.3170188387650512141, 0.3333333333333333703, 0.3170188387650512141, 0.3333333333333333703, 0.3170188387650512141, 0.3333333333333333703, 0.3170188387650512141, 0.3333333333333333703, 0.3170188387650512141, 0.3333333333333333703, 0.3170188387650512141, 0.3333333333333333703, 0.3170188387650512141, 0.3333333333333333703, 0.3170188387650512141, 0.3333333333333333703, 0.3170188387650512141, 0.3333333333333333703, 0.3170188387650512141, 0.3333333333333333703, 0.3170188387650512141, 0.3333333333333333703, 0.3170188387650512141, 0.3333333333333333703, 0.3170188387650512141, 0.3333333333333333703, 0.3170188387650512141, 0.3333333333333333703, 0.3170188387650512141, 0.3333333333333333703, 0.3170188387650512141, 0.3333333333333333703, 0.3170188387650512141, 0.3333333333333333703, 0.3170188387650512141, 0.3333333333333333703, 0.3170188387650512141, 0.3333333333333333703, 0.3170188387650512141, 0.3333333333333333703, 0.3170188387650512141, 0.3333333333333333703, 0.3170188387650512141, 0.3333333333333333703, 0.3170188387650512141, 0.3333333333333333703, 0.3170188387650512141, 0.3333333333333333703, 0.3170188387650512141, 0.3333333333333333703, 0.3170188387650512141, 0.3333333333333333703, 0.3170188387650512141, 0.3333333333333333703, 0.3170188387650512141, 0.3333333333333333703, 0.3170188387650512141, 0.3333333333333333703, 0.3170188387650512141, 0.3333333333333333703, 0.3170188387650512141, 0.3333333333333333703, 0.3170188387650512141, 0.3333333333333333703, 0.3170188387650512141, 0.3333333333333333703, 0.3170188387650512141, 0.3333333333333333703, 0.3170188387650512141, 0.3333333333333333703, 0.3170188387650512141, 0.3333333333333333703, 0.3170188387650512141, 0.3333333333333333703, 0.3170188387650512141, 0.3333333333333333703, 0.3170188387650512141, 0.3333333333333333703, 0.3170188387650512141, 0.3333333333333333703, 0.3170188387650512141, 0.3333333333333333703, 0.3170188387650512141, 0.3333333333333333703, 0.3170188387650512141, 0.3333333333333333703, 0.3170188387650512141, 0.3333333333333333703, 0.3170188387650512141, 0.3333333333333333703, 0.3170188387650512141, 0.3333333333333333703, 0.3170188387650512141, 0.3333333333333333703, 0.3170188387650512141, 0.3333333333333333703, 0.3170188387650512141, 0.3333333333333333703, 0.3170188387650512141, 0.3333333333333333703, 0.3170188387650512141, 0.3333333333333333703, 0.3170188387650512141, 0.3333333333333333703, 0.3170188387650512141, 0.3333333333333333703, 0.3170188387650512141, 0.3333333333333333703, 0.3170188387650512141, 0.3333333333333333703, 0.3170188387650512141, 0.3333333333333333703, 0.3170188387650512141, 0.3333333333333333703, 0.3170188387650512141, 0.3333333333333333703, 0.3170188387650512141, 0.3333333333333333703, 0.3170188387650512141, 0.3333333333333333703, 0.3170188387650512141, 0.3333333333333333703, 0.3170188387650512141, 0.3333333333333333703, 0.3170188387650512141, 0.3333333333333333703, 0.3170188387650512141, 0.3333333333333333703, 0.3170188387650512141, 0.3333333333333333703, 0.3170188387650512141, 0.3333333333333333703, 0.3170188387650512141, 0.3333333333333333703, 0.3170188387650512141, 0.3333333333333333703, 0.3170188387650512141, 0.3333333333333333703, 0.3170188387650512141, 0.3333333333333333703, 0.3170188387650512141, 0.3333333333333333703, 0.3170188387650512141, 0.3333333333333333703, 0.3170188387650512141, 0.3333333333333333703, 0.3170188387650512141, 0.3333333333333333703, 0.3170188387650512141, 0.3333333333333333703, 0.3170188387650512141, 0.3333333333333333703, 0.3170188387650512141, 0.3333333333333333703, 0.3170188387650512141, 0.3333333333333333703, 0.3170188387650512141, 0.3333333333333333703, 0.3170188387650512141, 0.3333333333333333703, 0.3170188387650512141, 0.3333333333333333703, 0.3170188387650512141, 0.3333333333333333703, 0.3170188387650512141, 0.3333333333333333703, 0.3170188387650512141, 0.3333333333333333703, 0.3170188387650512141, 0.3333333333333333703, 0.3170188387650512141, 0.3333333333333333703, 0.3170188387650512141, 0.3333333333333333703, 0.3170188387650512141, 0.3333333333333333703, 0.3170188387650512141, 0.3333333333333333703, 0.3170188387650512141, 0.3333333333333333703, 0.3170188387650512141, 0.3333333333333333703, 0.3170188387650512141, 0.3333333333333333703, 0.3170188387650512141, 0.3333333333333333703, 0.3170188387650512141, 0.3333333333333333703, 0.3170188387650512141, 0.3333333333333333703, 0.3170188387650512141, 0.3333333333333333703, 0.3170188387650512141, 0.3333333333333333703, 0.3170188387650512141, 0.3333333333333333703, 0.3170188387650512141, 0.3333333333333333703, 0.3170188387650512141, 0.3333333333333333703, 0.3170188387650512141, 0.3333333333333333703, 0.3170188387650512141, 0.3333333333333333703, 0.3170188387650512141, 0.3333333333333333703, 0.3170188387650512141, 0.3333333333333333703, 0.3170188387650512141, 0.3333333333333333703, 0.3170188387650512141, 0.3333333333333333703, 0.3170188387650512141, 0.3333333333333333703, 0.3170188387650512141, 0.3333333333333333703, 0.3170188387650512141, 0.3333333333333333703, 0.3170188387650512141, 0.3333333333333333703, 0.3170188387650512141, 0.3333333333333333703, 0.3170188387650512141, 0.3333333333333333703, 0.3170188387650512141, 0.3333333333333333703, 0.3170188387650512141, 0.3333333333333333703, 0.3170188387650512141, 0.3333333333333333703, 0.3170188387650512141, 0.3333333333333333703, 0.3170188387650512141, 0.3333333333333333703, 0.3170188387650512141, 0.3333333333333333703, 0.3170188387650512141, 0.3333333333333333703, 0.3170188387650512141, 0.3333333333333333703, 0.3170188387650512141, 0.3333333333333333703, 0.3170188387650512141, 0.3333333333333333703, 0.3170188387650512141, 0.3333333333333333703, 0.3170188387650512141, 0.3333333333333333703, 0.3170188387650512141, 0.3333333333333333703, 0.3170188387650512141, 0.3333333333333333703, 0.3170188387650512141, 0.3333333333333333703, 0.3170188387650512141, 0.3333333333333333703, 0.3170188387650512141, 0.3333333333333333703, 0.3170188387650512141, 0.3333333333333333703, 0.3170188387650512141, 0.3333333333333333703, 0.3170188387650512141, 0.3333333333333333703, 0.3170188387650512141, 0.3333333333333333703, 0.3170188387650512141, 0.3333333333333333703, 0.3170188387650512141, 0.3333333333333333703, 0.3170188387650512141, 0.3333333333333333703, 0.3170188387650512141, 0.3333333333333333703, 0.3170188387650512141, 0.3333333333333333703, 0.3170188387650512141, 0.3333333333333333703, 0.3170188387650512141, 0.3333333333333333703, 0.3170188387650512141, 0.3333333333333333703, 0.3170188387650512141, 0.3333333333333333703, 0.3170188387650512141, 0.3333333333333333703, 0.3170188387650512141, 0.3333333333333333703, 0.3170188387650512141, 0.3333333333333333703, 0.3170188387650512141, 0.3333333333333333703, 0.3170188387650512141, 0.3333333333333333703, 0.3170188387650512141, 0.3333333333333333703, 0.3170188387650512141, 0.3333333333333333703, 0.3170188387650512141, 0.3333333333333333703, 0.3170188387650512141, 0.3333333333333333703, 0.3170188387650512141, 0.3333333333333333703, 0.3170188387650512141, 0.3333333333333333703, 0.3170188387650512141, 0.3333333333333333703, 0.3170188387650512141, 0.3333333333333333703, 0.3170188387650512141, 0.3333333333333333703, 0.3170188387650512141, 0.3333333333333333703, 0.3170188387650512141, 0.3333333333333333703, 0.3170188387650512141, 0.3333333333333333703, 0.3170188387650512141, 0.3333333333333333703, 0.3170188387650512141, 0.3333333333333333703, 0.3170188387650512141, 0.3333333333333333703, 0.3170188387650512141, 0.3333333333333333703, 0.3170188387650512141, 0.3333333333333333703, 0.3170188387650512141, 0.3333333333333333703, 0.3170188387650512141, 0.3333333333333333703, 0.3170188387650512141, 0.3333333333333333703, 0.3170188387650512141, 0.3333333333333333703, 0.3170188387650512141, 0.3333333333333333703, 0.3170188387650512141, 0.3333333333333333703, 0.3170188387650512141, 0.3333333333333333703, 0.3170188387650512141, 0.3333333333333333703, 0.3170188387650512141, 0.3333333333333333703, 0.3170188387650512141, 0.3333333333333333703, 0.3170188387650512141, 0.3333333333333333703, 0.3170188387650512141, 0.3333333333333333703, 0.3170188387650512141, 0.3333333333333333703, 0.3170188387650512141, 0.3333333333333333703, 0.3170188387650512141, 0.3333333333333333703, 0.3170188387650512141, 0.3333333333333333703, 0.3170188387650512141, 0.3333333333333333703, 0.3170188387650512141, 0.3333333333333333703, 0.3170188387650512141, 0.3333333333333333703, 0.3170188387650512141, 0.3333333333333333703, 0.3170188387650512141, 0.3333333333333333703, 0.3170188387650512141, 0.3333333333333333703, 0.3170188387650512141, 0.3333333333333333703, 0.3170188387650512141, 0.3333333333333333703, 0.3170188387650512141, 0.3333333333333333703, 0.3170188387650512141, 0.3333333333333333703, 0.3170188387650512141, 0.3333333333333333703, 0.3170188387650512141, 0.3333333333333333703, 0.3170188387650512141, 0.3333333333333333703, 0.3170188387650512141, 0.3333333333333333703, 0.3170188387650512141, 0.3333333333333333703, 0.3170188387650512141, 0.3333333333333333703, 0.3170188387650512141, 0.3333333333333333703, 0.3170188387650512141, 0.3333333333333333703, 0.3170188387650512141, 0.3333333333333333703, 0.3170188387650512141, 0.3333333333333333703, 0.3170188387650512141, 0.3333333333333333703, 0.3170188387650512141, 0.3333333333333333703, 0.3170188387650512141, 0.3333333333333333703, 0.3170188387650512141, 0.3333333333333333703, 0.3170188387650512141, 0.3333333333333333703, 0.3170188387650512141, 0.3333333333333333703, 0.3170188387650512141, 0.3333333333333333703, 0.3170188387650512141, 0.3333333333333333703, 0.3170188387650512141, 0.3333333333333333703, 0.3170188387650512141, 0.3333333333333333703, 0.3170188387650512141, 0.3333333333333333703, 0.3170188387650512141, 0.3333333333333333703, 0.3170188387650512141, 0.3333333333333333703, 0.3170188387650512141, 0.3333333333333333703, 0.3170188387650512141, 0.3333333333333333703, 0.3170188387650512141, 0.3333333333333333703, 0.3170188387650512141, 0.3333333333333333703, 0.3170188387650512141, 0.3333333333333333703, 0.3170188387650512141, 0.3333333333333333703, 0.3170188387650512141, 0.3333333333333333703, 0.3170188387650512141, 0.3333333333333333703, 0.3170188387650512141, 0.3333333333333333703, 0.3170188387650512141, 0.3333333333333333703, 0.3170188387650512141, 0.3333333333333333703, 0.3170188387650512141, 0.3333333333333333703, 0.3170188387650512141, 0.3333333333333333703, 0.3170188387650512141, 0.3333333333333333703, 0.3170188387650512141, 0.3333333333333333703, 0.3170188387650512141, 0.3333333333333333703, 0.3170188387650512141, 0.3333333333333333703, 0.3170188387650512141, 0.3333333333333333703, 0.3170188387650512141, 0.3333333333333333703, 0.3170188387650512141, 0.3333333333333333703, 0.3170188387650512141, 0.3333333333333333703, 0.3170188387650512141, 0.3333333333333333703, 0.3170188387650512141, 0.3333333333333333703, 0.3170188387650512141, 0.3333333333333333703, 0.3170188387650512141, 0.3333333333333333703, 0.3170188387650512141, 0.3333333333333333703, 0.3170188387650512141, 0.3333333333333333703, 0.3170188387650512141, 0.3333333333333333703, 0.3170188387650512141, 0.3333333333333333703, 0.3170188387650512141, 0.3333333333333333703, 0.3170188387650512141, 0.3333333333333333703, 0.3170188387650512141, 0.3333333333333333703, 0.3170188387650512141, 0.3333333333333333703, 0.3170188387650512141, 0.3333333333333333703, 0.3170188387650512141, 0.3333333333333333703, 0.3170188387650512141, 0.3333333333333333703, 0.3170188387650512141, 0.3333333333333333703, 0.3170188387650512141, 0.3333333333333333703, 0.3170188387650512141, 0.3333333333333333703, 0.3170188387650512141, 0.3333333333333333703, 0.3170188387650512141, 0.3333333333333333703, 0.3170188387650512141, 0.3333333333333333703, 0.3170188387650512141, 0.3333333333333333703, 0.3170188387650512141, 0.3333333333333333703, 0.3170188387650512141, 0.3333333333333333703, 0.3170188387650512141, 0.3333333333333333703, 0.3170188387650512141, 0.3333333333333333703, 0.3170188387650512141, 0.3333333333333333703, 0.3170188387650512141, 0.3333333333333333703, 0.3170188387650512141, 0.3333333333333333703, 0.3170188387650512141, 0.3333333333333333703, 0.3170188387650512141, 0.3333333333333333703, 0.3170188387650512141, 0.3333333333333333703, 0.3170188387650512141, 0.3333333333333333703, 0.3170188387650512141, 0.3333333333333333703, 0.3170188387650512141, 0.3333333333333333703, 0.3170188387650512141, 0.3333333333333333703, 0.3170188387650512141, 0.3333333333333333703, 0.3170188387650512141, 0.3333333333333333703, 0.3170188387650512141, 0.3333333333333333703, 0.3170188387650512141, 0.3333333333333333703, 0.3170188387650512141, 0.3333333333333333703, 0.3170188387650512141, 0.3333333333333333703, 0.3170188387650512141, 0.3333333333333333703, 0.3170188387650512141, 0.3333333333333333703, 0.3170188387650512141, 0.3333333333333333703, 0.3170188387650512141, 0.3333333333333333703, 0.3170188387650512141, 0.3333333333333333703, 0.3170188387650512141, 0.3333333333333333703, 0.3170188387650512141, 0.3333333333333333703, 0.3170188387650512141, 0.3333333333333333703, 0.3170188387650512141, 0.3333333333333333703, 0.3170188387650512141, 0.3333333333333333703, 0.3170188387650512141, 0.3333333333333333703, 0.3170188387650512141, 0.3333333333333333703, 0.3170188387650512141, 0.3333333333333333703, 0.3170188387650512141, 0.3333333333333333703, 0.3170188387650512141, 0.3333333333333333703, 0.3170188387650512141, 0.3333333333333333703, 0.3170188387650512141, 0.3333333333333333703, 0.3170188387650512141, 0.3333333333333333703, 0.3170188387650512141, 0.3333333333333333703, 0.3170188387650512141, 0.3333333333333333703, 0.3170188387650512141, 0.3333333333333333703, 0.3170188387650512141, 0.3333333333333333703, 0.3170188387650512141, 0.3333333333333333703, 0.3170188387650512141, 0.3333333333333333703, 0.3170188387650512141, 0.3333333333333333703, 0.3170188387650512141, 0.3333333333333333703, 0.3170188387650512141, 0.3333333333333333703, 0.3170188387650512141, 0.3333333333333333703, 0.3170188387650512141, 0.3333333333333333703, 0.3170188387650512141, 0.3333333333333333703, 0.3170188387650512141, 0.3333333333333333703, 0.3170188387650512141, 0.3333333333333333703, 0.3170188387650512141, 0.3333333333333333703, 0.3170188387650512141, 0.3333333333333333703, 0.3170188387650512141, 0.3333333333333333703, 0.3170188387650512141, 0.3333333333333333703, 0.3170188387650512141, 0.3333333333333333703, 0.3170188387650512141, 0.3333333333333333703, 0.3170188387650512141, 0.3333333333333333703, 0.3333333333333333703, 0.3333333333333333703),
 ( 0.3333333333333333703, 0.3170188387650512141, 0.3333333333333333703, 0.3170188387650512141, 0.3333333333333333703, 0.3170188387650512141, 0.3333333333333333703, 0.3170188387650512141, 0.3333333333333333703, 0.3170188387650512141, 0.3333333333333333703, 0.3170188387650512141, 0.3333333333333333703, 0.3170188387650512141, 0.3333333333333333703, 0.3170188387650512141, 0.3333333333333333703, 0.3170188387650512141, 0.3333333333333333703, 0.3170188387650512141, 0.3333333333333333703, 0.3170188387650512141, 0.3333333333333333703, 0.3170188387650512141, 0.3333333333333333703, 0.3170188387650512141, 0.3333333333333333703, 0.3170188387650512141, 0.3333333333333333703, 0.3170188387650512141, 0.3333333333333333703, 0.3170188387650512141, 0.3333333333333333703, 0.3170188387650512141, 0.3333333333333333703, 0.3170188387650512141, 0.3333333333333333703, 0.3170188387650512141, 0.3333333333333333703, 0.3170188387650512141, 0.3333333333333333703, 0.3170188387650512141, 0.3333333333333333703, 0.3170188387650512141, 0.3333333333333333703, 0.3170188387650512141, 0.3333333333333333703, 0.3170188387650512141, 0.3333333333333333703, 0.3170188387650512141, 0.3333333333333333703, 0.3170188387650512141, 0.3333333333333333703, 0.3170188387650512141, 0.3333333333333333703, 0.3170188387650512141, 0.3333333333333333703, 0.3170188387650512141, 0.3333333333333333703, 0.3170188387650512141, 0.3333333333333333703, 0.3170188387650512141, 0.3333333333333333703, 0.3170188387650512141, 0.3333333333333333703, 0.3170188387650512141, 0.3333333333333333703, 0.3170188387650512141, 0.3333333333333333703, 0.3170188387650512141, 0.3333333333333333703, 0.3170188387650512141, 0.3333333333333333703, 0.3170188387650512141, 0.3333333333333333703, 0.3170188387650512141, 0.3333333333333333703, 0.3170188387650512141, 0.3333333333333333703, 0.3170188387650512141, 0.3333333333333333703, 0.3170188387650512141, 0.3333333333333333703, 0.3170188387650512141, 0.3333333333333333703, 0.3170188387650512141, 0.3333333333333333703, 0.3170188387650512141, 0.3333333333333333703, 0.3170188387650512141, 0.3333333333333333703, 0.3170188387650512141, 0.3333333333333333703, 0.3170188387650512141, 0.3333333333333333703, 0.3170188387650512141, 0.3333333333333333703, 0.3170188387650512141, 0.3333333333333333703, 0.3170188387650512141, 0.3333333333333333703, 0.3170188387650512141, 0.3333333333333333703, 0.3170188387650512141, 0.3333333333333333703, 0.3170188387650512141, 0.3333333333333333703, 0.3170188387650512141, 0.3333333333333333703, 0.3170188387650512141, 0.3333333333333333703, 0.3170188387650512141, 0.3333333333333333703, 0.3170188387650512141, 0.3333333333333333703, 0.3170188387650512141, 0.3333333333333333703, 0.3170188387650512141, 0.3333333333333333703, 0.3170188387650512141, 0.3333333333333333703, 0.3170188387650512141, 0.3333333333333333703, 0.3170188387650512141, 0.3333333333333333703, 0.3170188387650512141, 0.3333333333333333703, 0.3170188387650512141, 0.3333333333333333703, 0.3170188387650512141, 0.3333333333333333703, 0.3170188387650512141, 0.3333333333333333703, 0.3170188387650512141, 0.3333333333333333703, 0.3170188387650512141, 0.3333333333333333703, 0.3170188387650512141, 0.3333333333333333703, 0.3170188387650512141, 0.3333333333333333703, 0.3170188387650512141, 0.3333333333333333703, 0.3170188387650512141, 0.3333333333333333703, 0.3170188387650512141, 0.3333333333333333703, 0.3170188387650512141, 0.3333333333333333703, 0.3170188387650512141, 0.3333333333333333703, 0.3170188387650512141, 0.3333333333333333703, 0.3170188387650512141, 0.3333333333333333703, 0.3170188387650512141, 0.3333333333333333703, 0.3170188387650512141, 0.3333333333333333703, 0.3170188387650512141, 0.3333333333333333703, 0.3170188387650512141, 0.3333333333333333703, 0.3170188387650512141, 0.3333333333333333703, 0.3170188387650512141, 0.3333333333333333703, 0.3170188387650512141, 0.3333333333333333703, 0.3170188387650512141, 0.3333333333333333703, 0.3170188387650512141, 0.3333333333333333703, 0.3170188387650512141, 0.3333333333333333703, 0.3170188387650512141, 0.3333333333333333703, 0.3170188387650512141, 0.3333333333333333703, 0.3170188387650512141, 0.3333333333333333703, 0.3170188387650512141, 0.3333333333333333703, 0.3170188387650512141, 0.3333333333333333703, 0.3170188387650512141, 0.3333333333333333703, 0.3170188387650512141, 0.3333333333333333703, 0.3170188387650512141, 0.3333333333333333703, 0.3170188387650512141, 0.3333333333333333703, 0.3170188387650512141, 0.3333333333333333703, 0.3170188387650512141, 0.3333333333333333703, 0.3170188387650512141, 0.3333333333333333703, 0.3170188387650512141, 0.3333333333333333703, 0.3170188387650512141, 0.3333333333333333703, 0.3170188387650512141, 0.3333333333333333703, 0.3170188387650512141, 0.3333333333333333703, 0.3170188387650512141, 0.3333333333333333703, 0.3170188387650512141, 0.3333333333333333703, 0.3170188387650512141, 0.3333333333333333703, 0.3170188387650512141, 0.3333333333333333703, 0.3170188387650512141, 0.3333333333333333703, 0.3170188387650512141, 0.3333333333333333703, 0.3170188387650512141, 0.3333333333333333703, 0.3170188387650512141, 0.3333333333333333703, 0.3170188387650512141, 0.3333333333333333703, 0.3170188387650512141, 0.3333333333333333703, 0.3170188387650512141, 0.3333333333333333703, 0.3170188387650512141, 0.3333333333333333703, 0.3170188387650512141, 0.3333333333333333703, 0.3170188387650512141, 0.3333333333333333703, 0.3170188387650512141, 0.3333333333333333703, 0.3170188387650512141, 0.3333333333333333703, 0.3170188387650512141, 0.3333333333333333703, 0.3170188387650512141, 0.3333333333333333703, 0.3170188387650512141, 0.3333333333333333703, 0.3170188387650512141, 0.3333333333333333703, 0.3170188387650512141, 0.3333333333333333703, 0.3170188387650512141, 0.3333333333333333703, 0.3170188387650512141, 0.3333333333333333703, 0.3170188387650512141, 0.3333333333333333703, 0.3170188387650512141, 0.3333333333333333703, 0.3170188387650512141, 0.3333333333333333703, 0.3170188387650512141, 0.3333333333333333703, 0.3170188387650512141, 0.3333333333333333703, 0.3170188387650512141, 0.3333333333333333703, 0.3170188387650512141, 0.3333333333333333703, 0.3170188387650512141, 0.3333333333333333703, 0.3170188387650512141, 0.3333333333333333703, 0.3170188387650512141, 0.3333333333333333703, 0.3170188387650512141, 0.3333333333333333703, 0.3170188387650512141, 0.3333333333333333703, 0.3170188387650512141, 0.3333333333333333703, 0.3170188387650512141, 0.3333333333333333703, 0.3170188387650512141, 0.3333333333333333703, 0.3170188387650512141, 0.3333333333333333703, 0.3170188387650512141, 0.3333333333333333703, 0.3170188387650512141, 0.3333333333333333703, 0.3170188387650512141, 0.3333333333333333703, 0.3170188387650512141, 0.3333333333333333703, 0.3170188387650512141, 0.3333333333333333703, 0.3170188387650512141, 0.3333333333333333703, 0.3170188387650512141, 0.3333333333333333703, 0.3170188387650512141, 0.3333333333333333703, 0.3170188387650512141, 0.3333333333333333703, 0.3170188387650512141, 0.3333333333333333703, 0.3170188387650512141, 0.3333333333333333703, 0.3170188387650512141, 0.3333333333333333703, 0.3170188387650512141, 0.3333333333333333703, 0.3170188387650512141, 0.3333333333333333703, 0.3170188387650512141, 0.3333333333333333703, 0.3170188387650512141, 0.3333333333333333703, 0.3170188387650512141, 0.3333333333333333703, 0.3170188387650512141, 0.3333333333333333703, 0.3170188387650512141, 0.3333333333333333703, 0.3170188387650512141, 0.3333333333333333703, 0.3170188387650512141, 0.3333333333333333703, 0.3170188387650512141, 0.3333333333333333703, 0.3170188387650512141, 0.3333333333333333703, 0.3170188387650512141, 0.3333333333333333703, 0.3170188387650512141, 0.3333333333333333703, 0.3170188387650512141, 0.3333333333333333703, 0.3170188387650512141, 0.3333333333333333703, 0.3170188387650512141, 0.3333333333333333703, 0.3170188387650512141, 0.3333333333333333703, 0.3170188387650512141, 0.3333333333333333703, 0.3170188387650512141, 0.3333333333333333703, 0.3170188387650512141, 0.3333333333333333703, 0.3170188387650512141, 0.3333333333333333703, 0.3170188387650512141, 0.3333333333333333703, 0.3170188387650512141, 0.3333333333333333703, 0.3170188387650512141, 0.3333333333333333703, 0.3170188387650512141, 0.3333333333333333703, 0.3170188387650512141, 0.3333333333333333703, 0.3170188387650512141, 0.3333333333333333703, 0.3170188387650512141, 0.3333333333333333703, 0.3170188387650512141, 0.3333333333333333703, 0.3170188387650512141, 0.3333333333333333703, 0.3170188387650512141, 0.3333333333333333703, 0.3170188387650512141, 0.3333333333333333703, 0.3170188387650512141, 0.3333333333333333703, 0.3170188387650512141, 0.3333333333333333703, 0.3170188387650512141, 0.3333333333333333703, 0.3170188387650512141, 0.3333333333333333703, 0.3170188387650512141, 0.3333333333333333703, 0.3170188387650512141, 0.3333333333333333703, 0.3170188387650512141, 0.3333333333333333703, 0.3170188387650512141, 0.3333333333333333703, 0.3170188387650512141, 0.3333333333333333703, 0.3170188387650512141, 0.3333333333333333703, 0.3170188387650512141, 0.3333333333333333703, 0.3170188387650512141, 0.3333333333333333703, 0.3170188387650512141, 0.3333333333333333703, 0.3170188387650512141, 0.3333333333333333703, 0.3170188387650512141, 0.3333333333333333703, 0.3170188387650512141, 0.3333333333333333703, 0.3170188387650512141, 0.3333333333333333703, 0.3170188387650512141, 0.3333333333333333703, 0.3170188387650512141, 0.3333333333333333703, 0.3170188387650512141, 0.3333333333333333703, 0.3170188387650512141, 0.3333333333333333703, 0.3170188387650512141, 0.3333333333333333703, 0.3170188387650512141, 0.3333333333333333703, 0.3170188387650512141, 0.3333333333333333703, 0.3170188387650512141, 0.3333333333333333703, 0.3170188387650512141, 0.3333333333333333703, 0.3170188387650512141, 0.3333333333333333703, 0.3170188387650512141, 0.3333333333333333703, 0.3170188387650512141, 0.3333333333333333703, 0.3170188387650512141, 0.3333333333333333703, 0.3170188387650512141, 0.3333333333333333703, 0.3170188387650512141, 0.3333333333333333703, 0.3170188387650512141, 0.3333333333333333703, 0.3170188387650512141, 0.3333333333333333703, 0.3170188387650512141, 0.3333333333333333703, 0.3170188387650512141, 0.3333333333333333703, 0.3170188387650512141, 0.3333333333333333703, 0.3170188387650512141, 0.3333333333333333703, 0.3170188387650512141, 0.3333333333333333703, 0.3170188387650512141, 0.3333333333333333703, 0.3170188387650512141, 0.3333333333333333703, 0.3170188387650512141, 0.3333333333333333703, 0.3170188387650512141, 0.3333333333333333703, 0.3170188387650512141, 0.3333333333333333703, 0.3170188387650512141, 0.3333333333333333703, 0.3170188387650512141, 0.3333333333333333703, 0.3170188387650512141, 0.3333333333333333703, 0.3170188387650512141, 0.3333333333333333703, 0.3170188387650512141, 0.3333333333333333703, 0.3170188387650512141, 0.3333333333333333703, 0.3170188387650512141, 0.3333333333333333703, 0.3170188387650512141, 0.3333333333333333703, 0.3170188387650512141, 0.3333333333333333703, 0.3170188387650512141, 0.3333333333333333703, 0.3170188387650512141, 0.3333333333333333703, 0.3170188387650512141, 0.3333333333333333703, 0.3170188387650512141, 0.3333333333333333703, 0.3170188387650512141, 0.3333333333333333703, 0.3170188387650512141, 0.3333333333333333703, 0.3170188387650512141, 0.3333333333333333703, 0.3170188387650512141, 0.3333333333333333703, 0.3170188387650512141, 0.3333333333333333703, 0.3170188387650512141, 0.3333333333333333703, 0.3170188387650512141, 0.3333333333333333703, 0.3170188387650512141, 0.3333333333333333703, 0.3170188387650512141, 0.3333333333333333703, 0.3170188387650512141, 0.3333333333333333703, 0.3170188387650512141, 0.3333333333333333703, 0.3170188387650512141, 0.3333333333333333703, 0.3170188387650512141, 0.3333333333333333703, 0.3170188387650512141, 0.3333333333333333703, 0.3170188387650512141, 0.3333333333333333703, 0.3170188387650512141, 0.3333333333333333703, 0.3170188387650512141, 0.3333333333333333703, 0.3170188387650512141, 0.3333333333333333703, 0.3170188387650512141, 0.3333333333333333703, 0.3170188387650512141, 0.3333333333333333703, 0.3170188387650512141, 0.3333333333333333703, 0.3170188387650512141, 0.3333333333333333703, 0.3170188387650512141, 0.3333333333333333703, 0.3170188387650512141, 0.3333333333333333703, 0.3170188387650512141, 0.3333333333333333703, 0.3170188387650512141, 0.3333333333333333703, 0.3170188387650512141, 0.3333333333333333703, 0.3170188387650512141, 0.3333333333333333703, 0.3170188387650512141, 0.3333333333333333703, 0.3170188387650512141, 0.3333333333333333703, 0.3170188387650512141, 0.3333333333333333703, 0.3170188387650512141, 0.3333333333333333703, 0.3170188387650512141, 0.3333333333333333703, 0.3170188387650512141, 0.3333333333333333703, 0.3170188387650512141, 0.3333333333333333703, 0.3170188387650512141, 0.3333333333333333703, 0.3170188387650512141, 0.3333333333333333703, 0.3170188387650512141, 0.3333333333333333703, 0.3170188387650512141, 0.3333333333333333703, 0.3170188387650512141, 0.3333333333333333703, 0.3170188387650512141, 0.3333333333333333703, 0.3170188387650512141, 0.3333333333333333703, 0.3170188387650512141, 0.3333333333333333703, 0.3170188387650512141, 0.3333333333333333703, 0.3170188387650512141, 0.3333333333333333703, 0.3170188387650512141, 0.3333333333333333703, 0.3170188387650512141, 0.3333333333333333703, 0.3170188387650512141, 0.3333333333333333703, 0.3170188387650512141, 0.3333333333333333703, 0.3170188387650512141, 0.3333333333333333703, 0.3170188387650512141, 0.3333333333333333703, 0.3170188387650512141, 0.3333333333333333703, 0.3170188387650512141, 0.3333333333333333703, 0.3170188387650512141, 0.3333333333333333703, 0.3170188387650512141, 0.3333333333333333703, 0.3170188387650512141, 0.3333333333333333703, 0.3170188387650512141, 0.3333333333333333703, 0.3170188387650512141, 0.3333333333333333703, 0.3170188387650512141, 0.3333333333333333703, 0.3170188387650512141, 0.3333333333333333703, 0.3170188387650512141, 0.3333333333333333703, 0.3170188387650512141, 0.3333333333333333703, 0.3170188387650512141, 0.3333333333333333703, 0.3170188387650512141, 0.3333333333333333703, 0.3170188387650512141, 0.3333333333333333703, 0.3170188387650512141, 0.3333333333333333703, 0.3170188387650512141, 0.3333333333333333703, 0.3170188387650512141, 0.3333333333333333703, 0.3170188387650512141, 0.3333333333333333703, 0.3170188387650512141, 0.3333333333333333703, 0.3170188387650512141, 0.3333333333333333703, 0.3170188387650512141, 0.3333333333333333703, 0.3170188387650512141, 0.3333333333333333703, 0.3170188387650512141, 0.3333333333333333703, 0.3170188387650512141, 0.3333333333333333703, 0.3170188387650512141, 0.3333333333333333703, 0.3170188387650512141, 0.3333333333333333703, 0.3170188387650512141, 0.3333333333333333703, 0.3170188387650512141, 0.3333333333333333703, 0.3170188387650512141, 0.3333333333333333703, 0.3170188387650512141, 0.3333333333333333703, 0.3170188387650512141, 0.3333333333333333703, 0.3170188387650512141, 0.3333333333333333703, 0.3170188387650512141, 0.3333333333333333703, 0.3170188387650512141, 0.3333333333333333703, 0.3170188387650512141, 0.3333333333333333703, 0.3170188387650512141, 0.3333333333333333703, 0.3170188387650512141, 0.3333333333333333703, 0.3170188387650512141, 0.3333333333333333703, 0.3170188387650512141, 0.3333333333333333703, 0.3170188387650512141, 0.3333333333333333703, 0.3170188387650512141, 0.3333333333333333703, 0.3170188387650512141, 0.3333333333333333703, 0.3170188387650512141, 0.3333333333333333703, 0.3170188387650512141, 0.3333333333333333703, 0.3170188387650512141, 0.3333333333333333703, 0.3170188387650512141, 0.3333333333333333703, 0.3170188387650512141, 0.3333333333333333703, 0.3170188387650512141, 0.3333333333333333703, 0.3170188387650512141, 0.3333333333333333703, 0.3170188387650512141, 0.3333333333333333703, 0.3170188387650512141, 0.3333333333333333703, 0.3333333333333333703, 0.3333333333333333703),
 ( 1.000000000000000000, 0.9510565162951535312, 1.000000000000000000, 0.9510565162951535312, 1.000000000000000000, 0.9510565162951535312, 1.000000000000000000, 0.9510565162951535312, 1.000000000000000000, 0.9510565162951535312, 1.000000000000000000, 0.9510565162951535312, 1.000000000000000000, 0.9510565162951535312, 1.000000000000000000, 0.9510565162951535312, 1.000000000000000000, 0.9510565162951535312, 1.000000000000000000, 0.9510565162951535312, 1.000000000000000000, 0.9510565162951535312, 1.000000000000000000, 0.9510565162951535312, 1.000000000000000000, 0.9510565162951535312, 1.000000000000000000, 0.9510565162951535312, 1.000000000000000000, 0.9510565162951535312, 1.000000000000000000, 0.9510565162951535312, 1.000000000000000000, 0.9510565162951535312, 1.000000000000000000, 0.9510565162951535312, 1.000000000000000000, 0.9510565162951535312, 1.000000000000000000, 0.9510565162951535312, 1.000000000000000000, 0.9510565162951535312, 1.000000000000000000, 0.9510565162951535312, 1.000000000000000000, 0.9510565162951535312, 1.000000000000000000, 0.9510565162951535312, 1.000000000000000000, 0.9510565162951535312, 1.000000000000000000, 0.9510565162951535312, 1.000000000000000000, 0.9510565162951535312, 1.000000000000000000, 0.9510565162951535312, 1.000000000000000000, 0.9510565162951535312, 1.000000000000000000, 0.9510565162951535312, 1.000000000000000000, 0.9510565162951535312, 1.000000000000000000, 0.9510565162951535312, 1.000000000000000000, 0.9510565162951535312, 1.000000000000000000, 0.9510565162951535312, 1.000000000000000000, 0.9510565162951535312, 1.000000000000000000, 0.9510565162951535312, 1.000000000000000000, 0.9510565162951535312, 1.000000000000000000, 0.9510565162951535312, 1.000000000000000000, 0.9510565162951535312, 1.000000000000000000, 0.9510565162951535312, 1.000000000000000000, 0.9510565162951535312, 1.000000000000000000, 0.9510565162951535312, 1.000000000000000000, 0.9510565162951535312, 1.000000000000000000, 0.9510565162951535312, 1.000000000000000000, 0.9510565162951535312, 1.000000000000000000, 0.9510565162951535312, 1.000000000000000000, 0.9510565162951535312, 1.000000000000000000, 0.9510565162951535312, 1.000000000000000000, 0.9510565162951535312, 1.000000000000000000, 0.9510565162951535312, 1.000000000000000000, 0.9510565162951535312, 1.000000000000000000, 0.9510565162951535312, 1.000000000000000000, 0.9510565162951535312, 1.000000000000000000, 0.9510565162951535312, 1.000000000000000000, 0.9510565162951535312, 1.000000000000000000, 0.9510565162951535312, 1.000000000000000000, 0.9510565162951535312, 1.000000000000000000, 0.9510565162951535312, 1.000000000000000000, 0.9510565162951535312, 1.000000000000000000, 0.9510565162951535312, 1.000000000000000000, 0.9510565162951535312, 1.000000000000000000, 0.9510565162951535312, 1.000000000000000000, 0.9510565162951535312, 1.000000000000000000, 0.9510565162951535312, 1.000000000000000000, 0.9510565162951535312, 1.000000000000000000, 0.9510565162951535312, 1.000000000000000000, 0.9510565162951535312, 1.000000000000000000, 0.9510565162951535312, 1.000000000000000000, 0.9510565162951535312, 1.000000000000000000, 0.9510565162951535312, 1.000000000000000000, 0.9510565162951535312, 1.000000000000000000, 0.9510565162951535312, 1.000000000000000000, 0.9510565162951535312, 1.000000000000000000, 0.9510565162951535312, 1.000000000000000000, 0.9510565162951535312, 1.000000000000000000, 0.9510565162951535312, 1.000000000000000000, 0.9510565162951535312, 1.000000000000000000, 0.9510565162951535312, 1.000000000000000000, 0.9510565162951535312, 1.000000000000000000, 0.9510565162951535312, 1.000000000000000000, 0.9510565162951535312, 1.000000000000000000, 0.9510565162951535312, 1.000000000000000000, 0.9510565162951535312, 1.000000000000000000, 0.9510565162951535312, 1.000000000000000000, 0.9510565162951535312, 1.000000000000000000, 0.9510565162951535312, 1.000000000000000000, 0.9510565162951535312, 1.000000000000000000, 0.9510565162951535312, 1.000000000000000000, 0.9510565162951535312, 1.000000000000000000, 0.9510565162951535312, 1.000000000000000000, 0.9510565162951535312, 1.000000000000000000, 0.9510565162951535312, 1.000000000000000000, 0.9510565162951535312, 1.000000000000000000, 0.9510565162951535312, 1.000000000000000000, 0.9510565162951535312, 1.000000000000000000, 0.9510565162951535312, 1.000000000000000000, 0.9510565162951535312, 1.000000000000000000, 0.9510565162951535312, 1.000000000000000000, 0.9510565162951535312, 1.000000000000000000, 0.9510565162951535312, 1.000000000000000000, 0.9510565162951535312, 1.000000000000000000, 0.9510565162951535312, 1.000000000000000000, 0.9510565162951535312, 1.000000000000000000, 0.9510565162951535312, 1.000000000000000000, 0.9510565162951535312, 1.000000000000000000, 0.9510565162951535312, 1.000000000000000000, 0.9510565162951535312, 1.000000000000000000, 0.9510565162951535312, 1.000000000000000000, 0.9510565162951535312, 1.000000000000000000, 0.9510565162951535312, 1.000000000000000000, 0.9510565162951535312, 1.000000000000000000, 0.9510565162951535312, 1.000000000000000000, 0.9510565162951535312, 1.000000000000000000, 0.9510565162951535312, 1.000000000000000000, 0.9510565162951535312, 1.000000000000000000, 0.9510565162951535312, 1.000000000000000000, 0.9510565162951535312, 1.000000000000000000, 0.9510565162951535312, 1.000000000000000000, 0.9510565162951535312, 1.000000000000000000, 0.9510565162951535312, 1.000000000000000000, 0.9510565162951535312, 1.000000000000000000, 0.9510565162951535312, 1.000000000000000000, 0.9510565162951535312, 1.000000000000000000, 0.9510565162951535312, 1.000000000000000000, 0.9510565162951535312, 1.000000000000000000, 0.9510565162951535312, 1.000000000000000000, 0.9510565162951535312, 1.000000000000000000, 0.9510565162951535312, 1.000000000000000000, 0.9510565162951535312, 1.000000000000000000, 0.9510565162951535312, 1.000000000000000000, 0.9510565162951535312, 1.000000000000000000, 0.9510565162951535312, 1.000000000000000000, 0.9510565162951535312, 1.000000000000000000, 0.9510565162951535312, 1.000000000000000000, 0.9510565162951535312, 1.000000000000000000, 0.9510565162951535312, 1.000000000000000000, 0.9510565162951535312, 1.000000000000000000, 0.9510565162951535312, 1.000000000000000000, 0.9510565162951535312, 1.000000000000000000, 0.9510565162951535312, 1.000000000000000000, 0.9510565162951535312, 1.000000000000000000, 0.9510565162951535312, 1.000000000000000000, 0.9510565162951535312, 1.000000000000000000, 0.9510565162951535312, 1.000000000000000000, 0.9510565162951535312, 1.000000000000000000, 0.9510565162951535312, 1.000000000000000000, 0.9510565162951535312, 1.000000000000000000, 0.9510565162951535312, 1.000000000000000000, 0.9510565162951535312, 1.000000000000000000, 0.9510565162951535312, 1.000000000000000000, 0.9510565162951535312, 1.000000000000000000, 0.9510565162951535312, 1.000000000000000000, 0.9510565162951535312, 1.000000000000000000, 0.9510565162951535312, 1.000000000000000000, 0.9510565162951535312, 1.000000000000000000, 0.9510565162951535312, 1.000000000000000000, 0.9510565162951535312, 1.000000000000000000, 0.9510565162951535312, 1.000000000000000000, 0.9510565162951535312, 1.000000000000000000, 0.9510565162951535312, 1.000000000000000000, 0.9510565162951535312, 1.000000000000000000, 0.9510565162951535312, 1.000000000000000000, 0.9510565162951535312, 1.000000000000000000, 0.9510565162951535312, 1.000000000000000000, 0.9510565162951535312, 1.000000000000000000, 0.9510565162951535312, 1.000000000000000000, 0.9510565162951535312, 1.000000000000000000, 0.9510565162951535312, 1.000000000000000000, 0.9510565162951535312, 1.000000000000000000, 0.9510565162951535312, 1.000000000000000000, 0.9510565162951535312, 1.000000000000000000, 0.9510565162951535312, 1.000000000000000000, 0.9510565162951535312, 1.000000000000000000, 0.9510565162951535312, 1.000000000000000000, 0.9510565162951535312, 1.000000000000000000, 0.9510565162951535312, 1.000000000000000000, 0.9510565162951535312, 1.000000000000000000, 0.9510565162951535312, 1.000000000000000000, 0.9510565162951535312, 1.000000000000000000, 0.9510565162951535312, 1.000000000000000000, 0.9510565162951535312, 1.000000000000000000, 0.9510565162951535312, 1.000000000000000000, 0.9510565162951535312, 1.000000000000000000, 0.9510565162951535312, 1.000000000000000000, 0.9510565162951535312, 1.000000000000000000, 0.9510565162951535312, 1.000000000000000000, 0.9510565162951535312, 1.000000000000000000, 0.9510565162951535312, 1.000000000000000000, 0.9510565162951535312, 1.000000000000000000, 0.9510565162951535312, 1.000000000000000000, 0.9510565162951535312, 1.000000000000000000, 0.9510565162951535312, 1.000000000000000000, 0.9510565162951535312, 1.000000000000000000, 0.9510565162951535312, 1.000000000000000000, 0.9510565162951535312, 1.000000000000000000, 0.9510565162951535312, 1.000000000000000000, 0.9510565162951535312, 1.000000000000000000, 0.9510565162951535312, 1.000000000000000000, 0.9510565162951535312, 1.000000000000000000, 0.9510565162951535312, 1.000000000000000000, 0.9510565162951535312, 1.000000000000000000, 0.9510565162951535312, 1.000000000000000000, 0.9510565162951535312, 1.000000000000000000, 0.9510565162951535312, 1.000000000000000000, 0.9510565162951535312, 1.000000000000000000, 0.9510565162951535312, 1.000000000000000000, 0.9510565162951535312, 1.000000000000000000, 0.9510565162951535312, 1.000000000000000000, 0.9510565162951535312, 1.000000000000000000, 0.9510565162951535312, 1.000000000000000000, 0.9510565162951535312, 1.000000000000000000, 0.9510565162951535312, 1.000000000000000000, 0.9510565162951535312, 1.000000000000000000, 0.9510565162951535312, 1.000000000000000000, 0.9510565162951535312, 1.000000000000000000, 0.9510565162951535312, 1.000000000000000000, 0.9510565162951535312, 1.000000000000000000, 0.9510565162951535312, 1.000000000000000000, 0.9510565162951535312, 1.000000000000000000, 0.9510565162951535312, 1.000000000000000000, 0.9510565162951535312, 1.000000000000000000, 0.9510565162951535312, 1.000000000000000000, 0.9510565162951535312, 1.000000000000000000, 0.9510565162951535312, 1.000000000000000000, 0.9510565162951535312, 1.000000000000000000, 0.9510565162951535312, 1.000000000000000000, 0.9510565162951535312, 1.000000000000000000, 0.9510565162951535312, 1.000000000000000000, 0.9510565162951535312, 1.000000000000000000, 0.9510565162951535312, 1.000000000000000000, 0.9510565162951535312, 1.000000000000000000, 0.9510565162951535312, 1.000000000000000000, 0.9510565162951535312, 1.000000000000000000, 0.9510565162951535312, 1.000000000000000000, 0.9510565162951535312, 1.000000000000000000, 0.9510565162951535312, 1.000000000000000000, 0.9510565162951535312, 1.000000000000000000, 0.9510565162951535312, 1.000000000000000000, 0.9510565162951535312, 1.000000000000000000, 0.9510565162951535312, 1.000000000000000000, 0.9510565162951535312, 1.000000000000000000, 0.9510565162951535312, 1.000000000000000000, 0.9510565162951535312, 1.000000000000000000, 0.9510565162951535312, 1.000000000000000000, 0.9510565162951535312, 1.000000000000000000, 0.9510565162951535312, 1.000000000000000000, 0.9510565162951535312, 1.000000000000000000, 0.9510565162951535312, 1.000000000000000000, 0.9510565162951535312, 1.000000000000000000, 0.9510565162951535312, 1.000000000000000000, 0.9510565162951535312, 1.000000000000000000, 0.9510565162951535312, 1.000000000000000000, 0.9510565162951535312, 1.000000000000000000, 0.9510565162951535312, 1.000000000000000000, 0.9510565162951535312, 1.000000000000000000, 0.9510565162951535312, 1.000000000000000000, 0.9510565162951535312, 1.000000000000000000, 0.9510565162951535312, 1.000000000000000000, 0.9510565162951535312, 1.000000000000000000, 0.9510565162951535312, 1.000000000000000000, 0.9510565162951535312, 1.000000000000000000, 0.9510565162951535312, 1.000000000000000000, 0.9510565162951535312, 1.000000000000000000, 0.9510565162951535312, 1.000000000000000000, 0.9510565162951535312, 1.000000000000000000, 0.9510565162951535312, 1.000000000000000000, 0.9510565162951535312, 1.000000000000000000, 0.9510565162951535312, 1.000000000000000000, 0.9510565162951535312, 1.000000000000000000, 0.9510565162951535312, 1.000000000000000000, 0.9510565162951535312, 1.000000000000000000, 0.9510565162951535312, 1.000000000000000000, 0.9510565162951535312, 1.000000000000000000, 0.9510565162951535312, 1.000000000000000000, 0.9510565162951535312, 1.000000000000000000, 0.9510565162951535312, 1.000000000000000000, 0.9510565162951535312, 1.000000000000000000, 0.9510565162951535312, 1.000000000000000000, 0.9510565162951535312, 1.000000000000000000, 0.9510565162951535312, 1.000000000000000000, 0.9510565162951535312, 1.000000000000000000, 0.9510565162951535312, 1.000000000000000000, 0.9510565162951535312, 1.000000000000000000, 0.9510565162951535312, 1.000000000000000000, 0.9510565162951535312, 1.000000000000000000, 0.9510565162951535312, 1.000000000000000000, 0.9510565162951535312, 1.000000000000000000, 0.9510565162951535312, 1.000000000000000000, 0.9510565162951535312, 1.000000000000000000, 0.9510565162951535312, 1.000000000000000000, 0.9510565162951535312, 1.000000000000000000, 0.9510565162951535312, 1.000000000000000000, 0.9510565162951535312, 1.000000000000000000, 0.9510565162951535312, 1.000000000000000000, 0.9510565162951535312, 1.000000000000000000, 0.9510565162951535312, 1.000000000000000000, 0.9510565162951535312, 1.000000000000000000, 0.9510565162951535312, 1.000000000000000000, 0.9510565162951535312, 1.000000000000000000, 0.9510565162951535312, 1.000000000000000000, 0.9510565162951535312, 1.000000000000000000, 0.9510565162951535312, 1.000000000000000000, 0.9510565162951535312, 1.000000000000000000, 0.9510565162951535312, 1.000000000000000000, 0.9510565162951535312, 1.000000000000000000, 0.9510565162951535312, 1.000000000000000000, 0.9510565162951535312, 1.000000000000000000, 0.9510565162951535312, 1.000000000000000000, 0.9510565162951535312, 1.000000000000000000, 0.9510565162951535312, 1.000000000000000000, 0.9510565162951535312, 1.000000000000000000, 0.9510565162951535312, 1.000000000000000000, 0.9510565162951535312, 1.000000000000000000, 0.9510565162951535312, 1.000000000000000000, 0.9510565162951535312, 1.000000000000000000, 0.9510565162951535312, 1.000000000000000000, 0.9510565162951535312, 1.000000000000000000, 0.9510565162951535312, 1.000000000000000000, 0.9510565162951535312, 1.000000000000000000, 0.9510565162951535312, 1.000000000000000000, 0.9510565162951535312, 1.000000000000000000, 0.9510565162951535312, 1.000000000000000000, 0.9510565162951535312, 1.000000000000000000, 0.9510565162951535312, 1.000000000000000000, 0.9510565162951535312, 1.000000000000000000, 0.9510565162951535312, 1.000000000000000000, 0.9510565162951535312, 1.000000000000000000, 0.9510565162951535312, 1.000000000000000000, 0.9510565162951535312, 1.000000000000000000, 0.9510565162951535312, 1.000000000000000000, 0.9510565162951535312, 1.000000000000000000, 0.9510565162951535312, 1.000000000000000000, 0.9510565162951535312, 1.000000000000000000, 0.9510565162951535312, 1.000000000000000000, 0.9510565162951535312, 1.000000000000000000, 0.9510565162951535312, 1.000000000000000000, 0.9510565162951535312, 1.000000000000000000, 0.9510565162951535312, 1.000000000000000000, 0.9510565162951535312, 1.000000000000000000, 0.9510565162951535312, 1.000000000000000000, 0.9510565162951535312, 1.000000000000000000, 0.9510565162951535312, 1.000000000000000000, 0.9510565162951535312, 1.000000000000000000, 0.9510565162951535312, 1.000000000000000000, 0.9510565162951535312, 1.000000000000000000, 1.000000000000000000, 1.000000000000000000),
 ( 0.3333333333333333703, 0.3170188387650512141, 0.3333333333333333703, 0.3170188387650512141, 0.3333333333333333703, 0.3170188387650512141, 0.3333333333333333703, 0.3170188387650512141, 0.3333333333333333703, 0.3170188387650512141, 0.3333333333333333703, 0.3170188387650512141, 0.3333333333333333703, 0.3170188387650512141, 0.3333333333333333703, 0.3170188387650512141, 0.3333333333333333703, 0.3170188387650512141, 0.3333333333333333703, 0.3170188387650512141, 0.3333333333333333703, 0.3170188387650512141, 0.3333333333333333703, 0.3170188387650512141, 0.3333333333333333703, 0.3170188387650512141, 0.3333333333333333703, 0.3170188387650512141, 0.3333333333333333703, 0.3170188387650512141, 0.3333333333333333703, 0.3170188387650512141, 0.3333333333333333703, 0.3170188387650512141, 0.3333333333333333703, 0.3170188387650512141, 0.3333333333333333703, 0.3170188387650512141, 0.3333333333333333703, 0.3170188387650512141, 0.3333333333333333703, 0.3170188387650512141, 0.3333333333333333703, 0.3170188387650512141, 0.3333333333333333703, 0.3170188387650512141, 0.3333333333333333703, 0.3170188387650512141, 0.3333333333333333703, 0.3170188387650512141, 0.3333333333333333703, 0.3170188387650512141, 0.3333333333333333703, 0.3170188387650512141, 0.3333333333333333703, 0.3170188387650512141, 0.3333333333333333703, 0.3170188387650512141, 0.3333333333333333703, 0.3170188387650512141, 0.3333333333333333703, 0.3170188387650512141, 0.3333333333333333703, 0.3170188387650512141, 0.3333333333333333703, 0.3170188387650512141, 0.3333333333333333703, 0.3170188387650512141, 0.3333333333333333703, 0.3170188387650512141, 0.3333333333333333703, 0.3170188387650512141, 0.3333333333333333703, 0.3170188387650512141, 0.3333333333333333703, 0.3170188387650512141, 0.3333333333333333703, 0.3170188387650512141, 0.3333333333333333703, 0.3170188387650512141, 0.3333333333333333703, 0.3170188387650512141, 0.3333333333333333703, 0.3170188387650512141, 0.3333333333333333703, 0.3170188387650512141, 0.3333333333333333703, 0.3170188387650512141, 0.3333333333333333703, 0.3170188387650512141, 0.3333333333333333703, 0.3170188387650512141, 0.3333333333333333703, 0.3170188387650512141, 0.3333333333333333703, 0.3170188387650512141, 0.3333333333333333703, 0.3170188387650512141, 0.3333333333333333703, 0.3170188387650512141, 0.3333333333333333703, 0.3170188387650512141, 0.3333333333333333703, 0.3170188387650512141, 0.3333333333333333703, 0.3170188387650512141, 0.3333333333333333703, 0.3170188387650512141, 0.3333333333333333703, 0.3170188387650512141, 0.3333333333333333703, 0.3170188387650512141, 0.3333333333333333703, 0.3170188387650512141, 0.3333333333333333703, 0.3170188387650512141, 0.3333333333333333703, 0.3170188387650512141, 0.3333333333333333703, 0.3170188387650512141, 0.3333333333333333703, 0.3170188387650512141, 0.3333333333333333703, 0.3170188387650512141, 0.3333333333333333703, 0.3170188387650512141, 0.3333333333333333703, 0.3170188387650512141, 0.3333333333333333703, 0.3170188387650512141, 0.3333333333333333703, 0.3170188387650512141, 0.3333333333333333703, 0.3170188387650512141, 0.3333333333333333703, 0.3170188387650512141, 0.3333333333333333703, 0.3170188387650512141, 0.3333333333333333703, 0.3170188387650512141, 0.3333333333333333703, 0.3170188387650512141, 0.3333333333333333703, 0.3170188387650512141, 0.3333333333333333703, 0.3170188387650512141, 0.3333333333333333703, 0.3170188387650512141, 0.3333333333333333703, 0.3170188387650512141, 0.3333333333333333703, 0.3170188387650512141, 0.3333333333333333703, 0.3170188387650512141, 0.3333333333333333703, 0.3170188387650512141, 0.3333333333333333703, 0.3170188387650512141, 0.3333333333333333703, 0.3170188387650512141, 0.3333333333333333703, 0.3170188387650512141, 0.3333333333333333703, 0.3170188387650512141, 0.3333333333333333703, 0.3170188387650512141, 0.3333333333333333703, 0.3170188387650512141, 0.3333333333333333703, 0.3170188387650512141, 0.3333333333333333703, 0.3170188387650512141, 0.3333333333333333703, 0.3170188387650512141, 0.3333333333333333703, 0.3170188387650512141, 0.3333333333333333703, 0.3170188387650512141, 0.3333333333333333703, 0.3170188387650512141, 0.3333333333333333703, 0.3170188387650512141, 0.3333333333333333703, 0.3170188387650512141, 0.3333333333333333703, 0.3170188387650512141, 0.3333333333333333703, 0.3170188387650512141, 0.3333333333333333703, 0.3170188387650512141, 0.3333333333333333703, 0.3170188387650512141, 0.3333333333333333703, 0.3170188387650512141, 0.3333333333333333703, 0.3170188387650512141, 0.3333333333333333703, 0.3170188387650512141, 0.3333333333333333703, 0.3170188387650512141, 0.3333333333333333703, 0.3170188387650512141, 0.3333333333333333703, 0.3170188387650512141, 0.3333333333333333703, 0.3170188387650512141, 0.3333333333333333703, 0.3170188387650512141, 0.3333333333333333703, 0.3170188387650512141, 0.3333333333333333703, 0.3170188387650512141, 0.3333333333333333703, 0.3170188387650512141, 0.3333333333333333703, 0.3170188387650512141, 0.3333333333333333703, 0.3170188387650512141, 0.3333333333333333703, 0.3170188387650512141, 0.3333333333333333703, 0.3170188387650512141, 0.3333333333333333703, 0.3170188387650512141, 0.3333333333333333703, 0.3170188387650512141, 0.3333333333333333703, 0.3170188387650512141, 0.3333333333333333703, 0.3170188387650512141, 0.3333333333333333703, 0.3170188387650512141, 0.3333333333333333703, 0.3170188387650512141, 0.3333333333333333703, 0.3170188387650512141, 0.3333333333333333703, 0.3170188387650512141, 0.3333333333333333703, 0.3170188387650512141, 0.3333333333333333703, 0.3170188387650512141, 0.3333333333333333703, 0.3170188387650512141, 0.3333333333333333703, 0.3170188387650512141, 0.3333333333333333703, 0.3170188387650512141, 0.3333333333333333703, 0.3170188387650512141, 0.3333333333333333703, 0.3170188387650512141, 0.3333333333333333703, 0.3170188387650512141, 0.3333333333333333703, 0.3170188387650512141, 0.3333333333333333703, 0.3170188387650512141, 0.3333333333333333703, 0.3170188387650512141, 0.3333333333333333703, 0.3170188387650512141, 0.3333333333333333703, 0.3170188387650512141, 0.3333333333333333703, 0.3170188387650512141, 0.3333333333333333703, 0.3170188387650512141, 0.3333333333333333703, 0.3170188387650512141, 0.3333333333333333703, 0.3170188387650512141, 0.3333333333333333703, 0.3170188387650512141, 0.3333333333333333703, 0.3170188387650512141, 0.3333333333333333703, 0.3170188387650512141, 0.3333333333333333703, 0.3170188387650512141, 0.3333333333333333703, 0.3170188387650512141, 0.3333333333333333703, 0.3170188387650512141, 0.3333333333333333703, 0.3170188387650512141, 0.3333333333333333703, 0.3170188387650512141, 0.3333333333333333703, 0.3170188387650512141, 0.3333333333333333703, 0.3170188387650512141, 0.3333333333333333703, 0.3170188387650512141, 0.3333333333333333703, 0.3170188387650512141, 0.3333333333333333703, 0.3170188387650512141, 0.3333333333333333703, 0.3170188387650512141, 0.3333333333333333703, 0.3170188387650512141, 0.3333333333333333703, 0.3170188387650512141, 0.3333333333333333703, 0.3170188387650512141, 0.3333333333333333703, 0.3170188387650512141, 0.3333333333333333703, 0.3170188387650512141, 0.3333333333333333703, 0.3170188387650512141, 0.3333333333333333703, 0.3170188387650512141, 0.3333333333333333703, 0.3170188387650512141, 0.3333333333333333703, 0.3170188387650512141, 0.3333333333333333703, 0.3170188387650512141, 0.3333333333333333703, 0.3170188387650512141, 0.3333333333333333703, 0.3170188387650512141, 0.3333333333333333703, 0.3170188387650512141, 0.3333333333333333703, 0.3170188387650512141, 0.3333333333333333703, 0.3170188387650512141, 0.3333333333333333703, 0.3170188387650512141, 0.3333333333333333703, 0.3170188387650512141, 0.3333333333333333703, 0.3170188387650512141, 0.3333333333333333703, 0.3170188387650512141, 0.3333333333333333703, 0.3170188387650512141, 0.3333333333333333703, 0.3170188387650512141, 0.3333333333333333703, 0.3170188387650512141, 0.3333333333333333703, 0.3170188387650512141, 0.3333333333333333703, 0.3170188387650512141, 0.3333333333333333703, 0.3170188387650512141, 0.3333333333333333703, 0.3170188387650512141, 0.3333333333333333703, 0.3170188387650512141, 0.3333333333333333703, 0.3170188387650512141, 0.3333333333333333703, 0.3170188387650512141, 0.3333333333333333703, 0.3170188387650512141, 0.3333333333333333703, 0.3170188387650512141, 0.3333333333333333703, 0.3170188387650512141, 0.3333333333333333703, 0.3170188387650512141, 0.3333333333333333703, 0.3170188387650512141, 0.3333333333333333703, 0.3170188387650512141, 0.3333333333333333703, 0.3170188387650512141, 0.3333333333333333703, 0.3170188387650512141, 0.3333333333333333703, 0.3170188387650512141, 0.3333333333333333703, 0.3170188387650512141, 0.3333333333333333703, 0.3170188387650512141, 0.3333333333333333703, 0.3170188387650512141, 0.3333333333333333703, 0.3170188387650512141, 0.3333333333333333703, 0.3170188387650512141, 0.3333333333333333703, 0.3170188387650512141, 0.3333333333333333703, 0.3170188387650512141, 0.3333333333333333703, 0.3170188387650512141, 0.3333333333333333703, 0.3170188387650512141, 0.3333333333333333703, 0.3170188387650512141, 0.3333333333333333703, 0.3170188387650512141, 0.3333333333333333703, 0.3170188387650512141, 0.3333333333333333703, 0.3170188387650512141, 0.3333333333333333703, 0.3170188387650512141, 0.3333333333333333703, 0.3170188387650512141, 0.3333333333333333703, 0.3170188387650512141, 0.3333333333333333703, 0.3170188387650512141, 0.3333333333333333703, 0.3170188387650512141, 0.3333333333333333703, 0.3170188387650512141, 0.3333333333333333703, 0.3170188387650512141, 0.3333333333333333703, 0.3170188387650512141, 0.3333333333333333703, 0.3170188387650512141, 0.3333333333333333703, 0.3170188387650512141, 0.3333333333333333703, 0.3170188387650512141, 0.3333333333333333703, 0.3170188387650512141, 0.3333333333333333703, 0.3170188387650512141, 0.3333333333333333703, 0.3170188387650512141, 0.3333333333333333703, 0.3170188387650512141, 0.3333333333333333703, 0.3170188387650512141, 0.3333333333333333703, 0.3170188387650512141, 0.3333333333333333703, 0.3170188387650512141, 0.3333333333333333703, 0.3170188387650512141, 0.3333333333333333703, 0.3170188387650512141, 0.3333333333333333703, 0.3170188387650512141, 0.3333333333333333703, 0.3170188387650512141, 0.3333333333333333703, 0.3170188387650512141, 0.3333333333333333703, 0.3170188387650512141, 0.3333333333333333703, 0.3170188387650512141, 0.3333333333333333703, 0.3170188387650512141, 0.3333333333333333703, 0.3170188387650512141, 0.3333333333333333703, 0.3170188387650512141, 0.3333333333333333703, 0.3170188387650512141, 0.3333333333333333703, 0.3170188387650512141, 0.3333333333333333703, 0.3170188387650512141, 0.3333333333333333703, 0.3170188387650512141, 0.3333333333333333703, 0.3170188387650512141, 0.3333333333333333703, 0.3170188387650512141, 0.3333333333333333703, 0.3170188387650512141, 0.3333333333333333703, 0.3170188387650512141, 0.3333333333333333703, 0.3170188387650512141, 0.3333333333333333703, 0.3170188387650512141, 0.3333333333333333703, 0.3170188387650512141, 0.3333333333333333703, 0.3170188387650512141, 0.3333333333333333703, 0.3170188387650512141, 0.3333333333333333703, 0.3170188387650512141, 0.3333333333333333703, 0.3170188387650512141, 0.3333333333333333703, 0.3170188387650512141, 0.3333333333333333703, 0.3170188387650512141, 0.3333333333333333703, 0.3170188387650512141, 0.3333333333333333703, 0.3170188387650512141, 0.3333333333333333703, 0.3170188387650512141, 0.3333333333333333703, 0.3170188387650512141, 0.3333333333333333703, 0.3170188387650512141, 0.3333333333333333703, 0.3170188387650512141, 0.3333333333333333703, 0.3170188387650512141, 0.3333333333333333703, 0.3170188387650512141, 0.3333333333333333703, 0.3170188387650512141, 0.3333333333333333703, 0.3170188387650512141, 0.3333333333333333703, 0.3170188387650512141, 0.3333333333333333703, 0.3170188387650512141, 0.3333333333333333703, 0.3170188387650512141, 0.3333333333333333703, 0.3170188387650512141, 0.3333333333333333703, 0.3170188387650512141, 0.3333333333333333703, 0.3170188387650512141, 0.3333333333333333703, 0.3170188387650512141, 0.3333333333333333703, 0.3170188387650512141, 0.3333333333333333703, 0.3170188387650512141, 0.3333333333333333703, 0.3170188387650512141, 0.3333333333333333703, 0.3170188387650512141, 0.3333333333333333703, 0.3170188387650512141, 0.3333333333333333703, 0.3170188387650512141, 0.3333333333333333703, 0.3170188387650512141, 0.3333333333333333703, 0.3170188387650512141, 0.3333333333333333703, 0.3170188387650512141, 0.3333333333333333703, 0.3170188387650512141, 0.3333333333333333703, 0.3170188387650512141, 0.3333333333333333703, 0.3170188387650512141, 0.3333333333333333703, 0.3170188387650512141, 0.3333333333333333703, 0.3170188387650512141, 0.3333333333333333703, 0.3170188387650512141, 0.3333333333333333703, 0.3170188387650512141, 0.3333333333333333703, 0.3170188387650512141, 0.3333333333333333703, 0.3170188387650512141, 0.3333333333333333703, 0.3170188387650512141, 0.3333333333333333703, 0.3170188387650512141, 0.3333333333333333703, 0.3170188387650512141, 0.3333333333333333703, 0.3170188387650512141, 0.3333333333333333703, 0.3170188387650512141, 0.3333333333333333703, 0.3170188387650512141, 0.3333333333333333703, 0.3170188387650512141, 0.3333333333333333703, 0.3170188387650512141, 0.3333333333333333703, 0.3170188387650512141, 0.3333333333333333703, 0.3170188387650512141, 0.3333333333333333703, 0.3170188387650512141, 0.3333333333333333703, 0.3170188387650512141, 0.3333333333333333703, 0.3170188387650512141, 0.3333333333333333703, 0.3170188387650512141, 0.3333333333333333703, 0.3170188387650512141, 0.3333333333333333703, 0.3170188387650512141, 0.3333333333333333703, 0.3170188387650512141, 0.3333333333333333703, 0.3170188387650512141, 0.3333333333333333703, 0.3170188387650512141, 0.3333333333333333703, 0.3170188387650512141, 0.3333333333333333703, 0.3170188387650512141, 0.3333333333333333703, 0.3170188387650512141, 0.3333333333333333703, 0.3170188387650512141, 0.3333333333333333703, 0.3170188387650512141, 0.3333333333333333703, 0.3170188387650512141, 0.3333333333333333703, 0.3170188387650512141, 0.3333333333333333703, 0.3170188387650512141, 0.3333333333333333703, 0.3170188387650512141, 0.3333333333333333703, 0.3170188387650512141, 0.3333333333333333703, 0.3170188387650512141, 0.3333333333333333703, 0.3170188387650512141, 0.3333333333333333703, 0.3170188387650512141, 0.3333333333333333703, 0.3170188387650512141, 0.3333333333333333703, 0.3170188387650512141, 0.3333333333333333703, 0.3170188387650512141, 0.3333333333333333703, 0.3170188387650512141, 0.3333333333333333703, 0.3170188387650512141, 0.3333333333333333703, 0.3170188387650512141, 0.3333333333333333703, 0.3170188387650512141, 0.3333333333333333703, 0.3170188387650512141, 0.3333333333333333703, 0.3170188387650512141, 0.3333333333333333703, 0.3170188387650512141, 0.3333333333333333703, 0.3170188387650512141, 0.3333333333333333703, 0.3170188387650512141, 0.3333333333333333703, 0.3170188387650512141, 0.3333333333333333703, 0.3170188387650512141, 0.3333333333333333703, 0.3170188387650512141, 0.3333333333333333703, 0.3170188387650512141, 0.3333333333333333703, 0.3170188387650512141, 0.3333333333333333703, 0.3170188387650512141, 0.3333333333333333703, 0.3170188387650512141, 0.3333333333333333703, 0.3170188387650512141, 0.3333333333333333703, 0.3170188387650512141, 0.3333333333333333703, 0.3170188387650512141, 0.3333333333333333703, 0.3170188387650512141, 0.3333333333333333703, 0.3170188387650512141, 0.3333333333333333703, 0.3170188387650512141, 0.3333333333333333703, 0.3170188387650512141, 0.3333333333333333703, 0.3170188387650512141, 0.3333333333333333703, 0.3170188387650512141, 0.3333333333333333703, 0.3170188387650512141, 0.3333333333333333703, 0.3170188387650512141, 0.3333333333333333703, 0.3170188387650512141, 0.3333333333333333703, 0.3170188387650512141, 0.3333333333333333703, 0.3333333333333333703, 0.3333333333333333703),
 ( 0.3333333333333333703, 0.3170188387650512141, 0.3333333333333333703, 0.3170188387650512141, 0.3333333333333333703, 0.3170188387650512141, 0.3333333333333333703, 0.3170188387650512141, 0.3333333333333333703, 0.3170188387650512141, 0.3333333333333333703, 0.3170188387650512141, 0.3333333333333333703, 0.3170188387650512141, 0.3333333333333333703, 0.3170188387650512141, 0.3333333333333333703, 0.3170188387650512141, 0.3333333333333333703, 0.3170188387650512141, 0.3333333333333333703, 0.3170188387650512141, 0.3333333333333333703, 0.3170188387650512141, 0.3333333333333333703, 0.3170188387650512141, 0.3333333333333333703, 0.3170188387650512141, 0.3333333333333333703, 0.3170188387650512141, 0.3333333333333333703, 0.3170188387650512141, 0.3333333333333333703, 0.3170188387650512141, 0.3333333333333333703, 0.3170188387650512141, 0.3333333333333333703, 0.3170188387650512141, 0.3333333333333333703, 0.3170188387650512141, 0.3333333333333333703, 0.3170188387650512141, 0.3333333333333333703, 0.3170188387650512141, 0.3333333333333333703, 0.3170188387650512141, 0.3333333333333333703, 0.3170188387650512141, 0.3333333333333333703, 0.3170188387650512141, 0.3333333333333333703, 0.3170188387650512141, 0.3333333333333333703, 0.3170188387650512141, 0.3333333333333333703, 0.3170188387650512141, 0.3333333333333333703, 0.3170188387650512141, 0.3333333333333333703, 0.3170188387650512141, 0.3333333333333333703, 0.3170188387650512141, 0.3333333333333333703, 0.3170188387650512141, 0.3333333333333333703, 0.3170188387650512141, 0.3333333333333333703, 0.3170188387650512141, 0.3333333333333333703, 0.3170188387650512141, 0.3333333333333333703, 0.3170188387650512141, 0.3333333333333333703, 0.3170188387650512141, 0.3333333333333333703, 0.3170188387650512141, 0.3333333333333333703, 0.3170188387650512141, 0.3333333333333333703, 0.3170188387650512141, 0.3333333333333333703, 0.3170188387650512141, 0.3333333333333333703, 0.3170188387650512141, 0.3333333333333333703, 0.3170188387650512141, 0.3333333333333333703, 0.3170188387650512141, 0.3333333333333333703, 0.3170188387650512141, 0.3333333333333333703, 0.3170188387650512141, 0.3333333333333333703, 0.3170188387650512141, 0.3333333333333333703, 0.3170188387650512141, 0.3333333333333333703, 0.3170188387650512141, 0.3333333333333333703, 0.3170188387650512141, 0.3333333333333333703, 0.3170188387650512141, 0.3333333333333333703, 0.3170188387650512141, 0.3333333333333333703, 0.3170188387650512141, 0.3333333333333333703, 0.3170188387650512141, 0.3333333333333333703, 0.3170188387650512141, 0.3333333333333333703, 0.3170188387650512141, 0.3333333333333333703, 0.3170188387650512141, 0.3333333333333333703, 0.3170188387650512141, 0.3333333333333333703, 0.3170188387650512141, 0.3333333333333333703, 0.3170188387650512141, 0.3333333333333333703, 0.3170188387650512141, 0.3333333333333333703, 0.3170188387650512141, 0.3333333333333333703, 0.3170188387650512141, 0.3333333333333333703, 0.3170188387650512141, 0.3333333333333333703, 0.3170188387650512141, 0.3333333333333333703, 0.3170188387650512141, 0.3333333333333333703, 0.3170188387650512141, 0.3333333333333333703, 0.3170188387650512141, 0.3333333333333333703, 0.3170188387650512141, 0.3333333333333333703, 0.3170188387650512141, 0.3333333333333333703, 0.3170188387650512141, 0.3333333333333333703, 0.3170188387650512141, 0.3333333333333333703, 0.3170188387650512141, 0.3333333333333333703, 0.3170188387650512141, 0.3333333333333333703, 0.3170188387650512141, 0.3333333333333333703, 0.3170188387650512141, 0.3333333333333333703, 0.3170188387650512141, 0.3333333333333333703, 0.3170188387650512141, 0.3333333333333333703, 0.3170188387650512141, 0.3333333333333333703, 0.3170188387650512141, 0.3333333333333333703, 0.3170188387650512141, 0.3333333333333333703, 0.3170188387650512141, 0.3333333333333333703, 0.3170188387650512141, 0.3333333333333333703, 0.3170188387650512141, 0.3333333333333333703, 0.3170188387650512141, 0.3333333333333333703, 0.3170188387650512141, 0.3333333333333333703, 0.3170188387650512141, 0.3333333333333333703, 0.3170188387650512141, 0.3333333333333333703, 0.3170188387650512141, 0.3333333333333333703, 0.3170188387650512141, 0.3333333333333333703, 0.3170188387650512141, 0.3333333333333333703, 0.3170188387650512141, 0.3333333333333333703, 0.3170188387650512141, 0.3333333333333333703, 0.3170188387650512141, 0.3333333333333333703, 0.3170188387650512141, 0.3333333333333333703, 0.3170188387650512141, 0.3333333333333333703, 0.3170188387650512141, 0.3333333333333333703, 0.3170188387650512141, 0.3333333333333333703, 0.3170188387650512141, 0.3333333333333333703, 0.3170188387650512141, 0.3333333333333333703, 0.3170188387650512141, 0.3333333333333333703, 0.3170188387650512141, 0.3333333333333333703, 0.3170188387650512141, 0.3333333333333333703, 0.3170188387650512141, 0.3333333333333333703, 0.3170188387650512141, 0.3333333333333333703, 0.3170188387650512141, 0.3333333333333333703, 0.3170188387650512141, 0.3333333333333333703, 0.3170188387650512141, 0.3333333333333333703, 0.3170188387650512141, 0.3333333333333333703, 0.3170188387650512141, 0.3333333333333333703, 0.3170188387650512141, 0.3333333333333333703, 0.3170188387650512141, 0.3333333333333333703, 0.3170188387650512141, 0.3333333333333333703, 0.3170188387650512141, 0.3333333333333333703, 0.3170188387650512141, 0.3333333333333333703, 0.3170188387650512141, 0.3333333333333333703, 0.3170188387650512141, 0.3333333333333333703, 0.3170188387650512141, 0.3333333333333333703, 0.3170188387650512141, 0.3333333333333333703, 0.3170188387650512141, 0.3333333333333333703, 0.3170188387650512141, 0.3333333333333333703, 0.3170188387650512141, 0.3333333333333333703, 0.3170188387650512141, 0.3333333333333333703, 0.3170188387650512141, 0.3333333333333333703, 0.3170188387650512141, 0.3333333333333333703, 0.3170188387650512141, 0.3333333333333333703, 0.3170188387650512141, 0.3333333333333333703, 0.3170188387650512141, 0.3333333333333333703, 0.3170188387650512141, 0.3333333333333333703, 0.3170188387650512141, 0.3333333333333333703, 0.3170188387650512141, 0.3333333333333333703, 0.3170188387650512141, 0.3333333333333333703, 0.3170188387650512141, 0.3333333333333333703, 0.3170188387650512141, 0.3333333333333333703, 0.3170188387650512141, 0.3333333333333333703, 0.3170188387650512141, 0.3333333333333333703, 0.3170188387650512141, 0.3333333333333333703, 0.3170188387650512141, 0.3333333333333333703, 0.3170188387650512141, 0.3333333333333333703, 0.3170188387650512141, 0.3333333333333333703, 0.3170188387650512141, 0.3333333333333333703, 0.3170188387650512141, 0.3333333333333333703, 0.3170188387650512141, 0.3333333333333333703, 0.3170188387650512141, 0.3333333333333333703, 0.3170188387650512141, 0.3333333333333333703, 0.3170188387650512141, 0.3333333333333333703, 0.3170188387650512141, 0.3333333333333333703, 0.3170188387650512141, 0.3333333333333333703, 0.3170188387650512141, 0.3333333333333333703, 0.3170188387650512141, 0.3333333333333333703, 0.3170188387650512141, 0.3333333333333333703, 0.3170188387650512141, 0.3333333333333333703, 0.3170188387650512141, 0.3333333333333333703, 0.3170188387650512141, 0.3333333333333333703, 0.3170188387650512141, 0.3333333333333333703, 0.3170188387650512141, 0.3333333333333333703, 0.3170188387650512141, 0.3333333333333333703, 0.3170188387650512141, 0.3333333333333333703, 0.3170188387650512141, 0.3333333333333333703, 0.3170188387650512141, 0.3333333333333333703, 0.3170188387650512141, 0.3333333333333333703, 0.3170188387650512141, 0.3333333333333333703, 0.3170188387650512141, 0.3333333333333333703, 0.3170188387650512141, 0.3333333333333333703, 0.3170188387650512141, 0.3333333333333333703, 0.3170188387650512141, 0.3333333333333333703, 0.3170188387650512141, 0.3333333333333333703, 0.3170188387650512141, 0.3333333333333333703, 0.3170188387650512141, 0.3333333333333333703, 0.3170188387650512141, 0.3333333333333333703, 0.3170188387650512141, 0.3333333333333333703, 0.3170188387650512141, 0.3333333333333333703, 0.3170188387650512141, 0.3333333333333333703, 0.3170188387650512141, 0.3333333333333333703, 0.3170188387650512141, 0.3333333333333333703, 0.3170188387650512141, 0.3333333333333333703, 0.3170188387650512141, 0.3333333333333333703, 0.3170188387650512141, 0.3333333333333333703, 0.3170188387650512141, 0.3333333333333333703, 0.3170188387650512141, 0.3333333333333333703, 0.3170188387650512141, 0.3333333333333333703, 0.3170188387650512141, 0.3333333333333333703, 0.3170188387650512141, 0.3333333333333333703, 0.3170188387650512141, 0.3333333333333333703, 0.3170188387650512141, 0.3333333333333333703, 0.3170188387650512141, 0.3333333333333333703, 0.3170188387650512141, 0.3333333333333333703, 0.3170188387650512141, 0.3333333333333333703, 0.3170188387650512141, 0.3333333333333333703, 0.3170188387650512141, 0.3333333333333333703, 0.3170188387650512141, 0.3333333333333333703, 0.3170188387650512141, 0.3333333333333333703, 0.3170188387650512141, 0.3333333333333333703, 0.3170188387650512141, 0.3333333333333333703, 0.3170188387650512141, 0.3333333333333333703, 0.3170188387650512141, 0.3333333333333333703, 0.3170188387650512141, 0.3333333333333333703, 0.3170188387650512141, 0.3333333333333333703, 0.3170188387650512141, 0.3333333333333333703, 0.3170188387650512141, 0.3333333333333333703, 0.3170188387650512141, 0.3333333333333333703, 0.3170188387650512141, 0.3333333333333333703, 0.3170188387650512141, 0.3333333333333333703, 0.3170188387650512141, 0.3333333333333333703, 0.3170188387650512141, 0.3333333333333333703, 0.3170188387650512141, 0.3333333333333333703, 0.3170188387650512141, 0.3333333333333333703, 0.3170188387650512141, 0.3333333333333333703, 0.3170188387650512141, 0.3333333333333333703, 0.3170188387650512141, 0.3333333333333333703, 0.3170188387650512141, 0.3333333333333333703, 0.3170188387650512141, 0.3333333333333333703, 0.3170188387650512141, 0.3333333333333333703, 0.3170188387650512141, 0.3333333333333333703, 0.3170188387650512141, 0.3333333333333333703, 0.3170188387650512141, 0.3333333333333333703, 0.3170188387650512141, 0.3333333333333333703, 0.3170188387650512141, 0.3333333333333333703, 0.3170188387650512141, 0.3333333333333333703, 0.3170188387650512141, 0.3333333333333333703, 0.3170188387650512141, 0.3333333333333333703, 0.3170188387650512141, 0.3333333333333333703, 0.3170188387650512141, 0.3333333333333333703, 0.3170188387650512141, 0.3333333333333333703, 0.3170188387650512141, 0.3333333333333333703, 0.3170188387650512141, 0.3333333333333333703, 0.3170188387650512141, 0.3333333333333333703, 0.3170188387650512141, 0.3333333333333333703, 0.3170188387650512141, 0.3333333333333333703, 0.3170188387650512141, 0.3333333333333333703, 0.3170188387650512141, 0.3333333333333333703, 0.3170188387650512141, 0.3333333333333333703, 0.3170188387650512141, 0.3333333333333333703, 0.3170188387650512141, 0.3333333333333333703, 0.3170188387650512141, 0.3333333333333333703, 0.3170188387650512141, 0.3333333333333333703, 0.3170188387650512141, 0.3333333333333333703, 0.3170188387650512141, 0.3333333333333333703, 0.3170188387650512141, 0.3333333333333333703, 0.3170188387650512141, 0.3333333333333333703, 0.3170188387650512141, 0.3333333333333333703, 0.3170188387650512141, 0.3333333333333333703, 0.3170188387650512141, 0.3333333333333333703, 0.3170188387650512141, 0.3333333333333333703, 0.3170188387650512141, 0.3333333333333333703, 0.3170188387650512141, 0.3333333333333333703, 0.3170188387650512141, 0.3333333333333333703, 0.3170188387650512141, 0.3333333333333333703, 0.3170188387650512141, 0.3333333333333333703, 0.3170188387650512141, 0.3333333333333333703, 0.3170188387650512141, 0.3333333333333333703, 0.3170188387650512141, 0.3333333333333333703, 0.3170188387650512141, 0.3333333333333333703, 0.3170188387650512141, 0.3333333333333333703, 0.3170188387650512141, 0.3333333333333333703, 0.3170188387650512141, 0.3333333333333333703, 0.3170188387650512141, 0.3333333333333333703, 0.3170188387650512141, 0.3333333333333333703, 0.3170188387650512141, 0.3333333333333333703, 0.3170188387650512141, 0.3333333333333333703, 0.3170188387650512141, 0.3333333333333333703, 0.3170188387650512141, 0.3333333333333333703, 0.3170188387650512141, 0.3333333333333333703, 0.3170188387650512141, 0.3333333333333333703, 0.3170188387650512141, 0.3333333333333333703, 0.3170188387650512141, 0.3333333333333333703, 0.3170188387650512141, 0.3333333333333333703, 0.3170188387650512141, 0.3333333333333333703, 0.3170188387650512141, 0.3333333333333333703, 0.3170188387650512141, 0.3333333333333333703, 0.3170188387650512141, 0.3333333333333333703, 0.3170188387650512141, 0.3333333333333333703, 0.3170188387650512141, 0.3333333333333333703, 0.3170188387650512141, 0.3333333333333333703, 0.3170188387650512141, 0.3333333333333333703, 0.3170188387650512141, 0.3333333333333333703, 0.3170188387650512141, 0.3333333333333333703, 0.3170188387650512141, 0.3333333333333333703, 0.3170188387650512141, 0.3333333333333333703, 0.3170188387650512141, 0.3333333333333333703, 0.3170188387650512141, 0.3333333333333333703, 0.3170188387650512141, 0.3333333333333333703, 0.3170188387650512141, 0.3333333333333333703, 0.3170188387650512141, 0.3333333333333333703, 0.3170188387650512141, 0.3333333333333333703, 0.3170188387650512141, 0.3333333333333333703, 0.3170188387650512141, 0.3333333333333333703, 0.3170188387650512141, 0.3333333333333333703, 0.3170188387650512141, 0.3333333333333333703, 0.3170188387650512141, 0.3333333333333333703, 0.3170188387650512141, 0.3333333333333333703, 0.3170188387650512141, 0.3333333333333333703, 0.3170188387650512141, 0.3333333333333333703, 0.3170188387650512141, 0.3333333333333333703, 0.3170188387650512141, 0.3333333333333333703, 0.3170188387650512141, 0.3333333333333333703, 0.3170188387650512141, 0.3333333333333333703, 0.3170188387650512141, 0.3333333333333333703, 0.3170188387650512141, 0.3333333333333333703, 0.3170188387650512141, 0.3333333333333333703, 0.3170188387650512141, 0.3333333333333333703, 0.3170188387650512141, 0.3333333333333333703, 0.3170188387650512141, 0.3333333333333333703, 0.3170188387650512141, 0.3333333333333333703, 0.3170188387650512141, 0.3333333333333333703, 0.3170188387650512141, 0.3333333333333333703, 0.3170188387650512141, 0.3333333333333333703, 0.3170188387650512141, 0.3333333333333333703, 0.3170188387650512141, 0.3333333333333333703, 0.3170188387650512141, 0.3333333333333333703, 0.3170188387650512141, 0.3333333333333333703, 0.3170188387650512141, 0.3333333333333333703, 0.3170188387650512141, 0.3333333333333333703, 0.3170188387650512141, 0.3333333333333333703, 0.3170188387650512141, 0.3333333333333333703, 0.3170188387650512141, 0.3333333333333333703, 0.3170188387650512141, 0.3333333333333333703, 0.3170188387650512141, 0.3333333333333333703, 0.3170188387650512141, 0.3333333333333333703, 0.3170188387650512141, 0.3333333333333333703, 0.3170188387650512141, 0.3333333333333333703, 0.3170188387650512141, 0.3333333333333333703, 0.3170188387650512141, 0.3333333333333333703, 0.3170188387650512141, 0.3333333333333333703, 0.3170188387650512141, 0.3333333333333333703, 0.3170188387650512141, 0.3333333333333333703, 0.3170188387650512141, 0.3333333333333333703, 0.3170188387650512141, 0.3333333333333333703, 0.3170188387650512141, 0.3333333333333333703, 0.3170188387650512141, 0.3333333333333333703, 0.3170188387650512141, 0.3333333333333333703, 0.3170188387650512141, 0.3333333333333333703, 0.3170188387650512141, 0.3333333333333333703, 0.3170188387650512141, 0.3333333333333333703, 0.3170188387650512141, 0.3333333333333333703, 0.3170188387650512141, 0.3333333333333333703, 0.3170188387650512141, 0.3333333333333333703, 0.3170188387650512141, 0.3333333333333333703, 0.3170188387650512141, 0.3333333333333333703, 0.3170188387650512141, 0.3333333333333333703, 0.3170188387650512141, 0.3333333333333333703, 0.3170188387650512141, 0.3333333333333333703, 0.3170188387650512141, 0.3333333333333333703, 0.3170188387650512141, 0.3333333333333333703, 0.3170188387650512141, 0.3333333333333333703, 0.3333333333333333703, 0.3333333333333333703),
 ( 1.000000000000000000, 0.9510565162951535312, 1.000000000000000000, 0.9510565162951535312, 1.000000000000000000, 0.9510565162951535312, 1.000000000000000000, 0.9510565162951535312, 1.000000000000000000, 0.9510565162951535312, 1.000000000000000000, 0.9510565162951535312, 1.000000000000000000, 0.9510565162951535312, 1.000000000000000000, 0.9510565162951535312, 1.000000000000000000, 0.9510565162951535312, 1.000000000000000000, 0.9510565162951535312, 1.000000000000000000, 0.9510565162951535312, 1.000000000000000000, 0.9510565162951535312, 1.000000000000000000, 0.9510565162951535312, 1.000000000000000000, 0.9510565162951535312, 1.000000000000000000, 0.9510565162951535312, 1.000000000000000000, 0.9510565162951535312, 1.000000000000000000, 0.9510565162951535312, 1.000000000000000000, 0.9510565162951535312, 1.000000000000000000, 0.9510565162951535312, 1.000000000000000000, 0.9510565162951535312, 1.000000000000000000, 0.9510565162951535312, 1.000000000000000000, 0.9510565162951535312, 1.000000000000000000, 0.9510565162951535312, 1.000000000000000000, 0.9510565162951535312, 1.000000000000000000, 0.9510565162951535312, 1.000000000000000000, 0.9510565162951535312, 1.000000000000000000, 0.9510565162951535312, 1.000000000000000000, 0.9510565162951535312, 1.000000000000000000, 0.9510565162951535312, 1.000000000000000000, 0.9510565162951535312, 1.000000000000000000, 0.9510565162951535312, 1.000000000000000000, 0.9510565162951535312, 1.000000000000000000, 0.9510565162951535312, 1.000000000000000000, 0.9510565162951535312, 1.000000000000000000, 0.9510565162951535312, 1.000000000000000000, 0.9510565162951535312, 1.000000000000000000, 0.9510565162951535312, 1.000000000000000000, 0.9510565162951535312, 1.000000000000000000, 0.9510565162951535312, 1.000000000000000000, 0.9510565162951535312, 1.000000000000000000, 0.9510565162951535312, 1.000000000000000000, 0.9510565162951535312, 1.000000000000000000, 0.9510565162951535312, 1.000000000000000000, 0.9510565162951535312, 1.000000000000000000, 0.9510565162951535312, 1.000000000000000000, 0.9510565162951535312, 1.000000000000000000, 0.9510565162951535312, 1.000000000000000000, 0.9510565162951535312, 1.000000000000000000, 0.9510565162951535312, 1.000000000000000000, 0.9510565162951535312, 1.000000000000000000, 0.9510565162951535312, 1.000000000000000000, 0.9510565162951535312, 1.000000000000000000, 0.9510565162951535312, 1.000000000000000000, 0.9510565162951535312, 1.000000000000000000, 0.9510565162951535312, 1.000000000000000000, 0.9510565162951535312, 1.000000000000000000, 0.9510565162951535312, 1.000000000000000000, 0.9510565162951535312, 1.000000000000000000, 0.9510565162951535312, 1.000000000000000000, 0.9510565162951535312, 1.000000000000000000, 0.9510565162951535312, 1.000000000000000000, 0.9510565162951535312, 1.000000000000000000, 0.9510565162951535312, 1.000000000000000000, 0.9510565162951535312, 1.000000000000000000, 0.9510565162951535312, 1.000000000000000000, 0.9510565162951535312, 1.000000000000000000, 0.9510565162951535312, 1.000000000000000000, 0.9510565162951535312, 1.000000000000000000, 0.9510565162951535312, 1.000000000000000000, 0.9510565162951535312, 1.000000000000000000, 0.9510565162951535312, 1.000000000000000000, 0.9510565162951535312, 1.000000000000000000, 0.9510565162951535312, 1.000000000000000000, 0.9510565162951535312, 1.000000000000000000, 0.9510565162951535312, 1.000000000000000000, 0.9510565162951535312, 1.000000000000000000, 0.9510565162951535312, 1.000000000000000000, 0.9510565162951535312, 1.000000000000000000, 0.9510565162951535312, 1.000000000000000000, 0.9510565162951535312, 1.000000000000000000, 0.9510565162951535312, 1.000000000000000000, 0.9510565162951535312, 1.000000000000000000, 0.9510565162951535312, 1.000000000000000000, 0.9510565162951535312, 1.000000000000000000, 0.9510565162951535312, 1.000000000000000000, 0.9510565162951535312, 1.000000000000000000, 0.9510565162951535312, 1.000000000000000000, 0.9510565162951535312, 1.000000000000000000, 0.9510565162951535312, 1.000000000000000000, 0.9510565162951535312, 1.000000000000000000, 0.9510565162951535312, 1.000000000000000000, 0.9510565162951535312, 1.000000000000000000, 0.9510565162951535312, 1.000000000000000000, 0.9510565162951535312, 1.000000000000000000, 0.9510565162951535312, 1.000000000000000000, 0.9510565162951535312, 1.000000000000000000, 0.9510565162951535312, 1.000000000000000000, 0.9510565162951535312, 1.000000000000000000, 0.9510565162951535312, 1.000000000000000000, 0.9510565162951535312, 1.000000000000000000, 0.9510565162951535312, 1.000000000000000000, 0.9510565162951535312, 1.000000000000000000, 0.9510565162951535312, 1.000000000000000000, 0.9510565162951535312, 1.000000000000000000, 0.9510565162951535312, 1.000000000000000000, 0.9510565162951535312, 1.000000000000000000, 0.9510565162951535312, 1.000000000000000000, 0.9510565162951535312, 1.000000000000000000, 0.9510565162951535312, 1.000000000000000000, 0.9510565162951535312, 1.000000000000000000, 0.9510565162951535312, 1.000000000000000000, 0.9510565162951535312, 1.000000000000000000, 0.9510565162951535312, 1.000000000000000000, 0.9510565162951535312, 1.000000000000000000, 0.9510565162951535312, 1.000000000000000000, 0.9510565162951535312, 1.000000000000000000, 0.9510565162951535312, 1.000000000000000000, 0.9510565162951535312, 1.000000000000000000, 0.9510565162951535312, 1.000000000000000000, 0.9510565162951535312, 1.000000000000000000, 0.9510565162951535312, 1.000000000000000000, 0.9510565162951535312, 1.000000000000000000, 0.9510565162951535312, 1.000000000000000000, 0.9510565162951535312, 1.000000000000000000, 0.9510565162951535312, 1.000000000000000000, 0.9510565162951535312, 1.000000000000000000, 0.9510565162951535312, 1.000000000000000000, 0.9510565162951535312, 1.000000000000000000, 0.9510565162951535312, 1.000000000000000000, 0.9510565162951535312, 1.000000000000000000, 0.9510565162951535312, 1.000000000000000000, 0.9510565162951535312, 1.000000000000000000, 0.9510565162951535312, 1.000000000000000000, 0.9510565162951535312, 1.000000000000000000, 0.9510565162951535312, 1.000000000000000000, 0.9510565162951535312, 1.000000000000000000, 0.9510565162951535312, 1.000000000000000000, 0.9510565162951535312, 1.000000000000000000, 0.9510565162951535312, 1.000000000000000000, 0.9510565162951535312, 1.000000000000000000, 0.9510565162951535312, 1.000000000000000000, 0.9510565162951535312, 1.000000000000000000, 0.9510565162951535312, 1.000000000000000000, 0.9510565162951535312, 1.000000000000000000, 0.9510565162951535312, 1.000000000000000000, 0.9510565162951535312, 1.000000000000000000, 0.9510565162951535312, 1.000000000000000000, 0.9510565162951535312, 1.000000000000000000, 0.9510565162951535312, 1.000000000000000000, 0.9510565162951535312, 1.000000000000000000, 0.9510565162951535312, 1.000000000000000000, 0.9510565162951535312, 1.000000000000000000, 0.9510565162951535312, 1.000000000000000000, 0.9510565162951535312, 1.000000000000000000, 0.9510565162951535312, 1.000000000000000000, 0.9510565162951535312, 1.000000000000000000, 0.9510565162951535312, 1.000000000000000000, 0.9510565162951535312, 1.000000000000000000, 0.9510565162951535312, 1.000000000000000000, 0.9510565162951535312, 1.000000000000000000, 0.9510565162951535312, 1.000000000000000000, 0.9510565162951535312, 1.000000000000000000, 0.9510565162951535312, 1.000000000000000000, 0.9510565162951535312, 1.000000000000000000, 0.9510565162951535312, 1.000000000000000000, 0.9510565162951535312, 1.000000000000000000, 0.9510565162951535312, 1.000000000000000000, 0.9510565162951535312, 1.000000000000000000, 0.9510565162951535312, 1.000000000000000000, 0.9510565162951535312, 1.000000000000000000, 0.9510565162951535312, 1.000000000000000000, 0.9510565162951535312, 1.000000000000000000, 0.9510565162951535312, 1.000000000000000000, 0.9510565162951535312, 1.000000000000000000, 0.9510565162951535312, 1.000000000000000000, 0.9510565162951535312, 1.000000000000000000, 0.9510565162951535312, 1.000000000000000000, 0.9510565162951535312, 1.000000000000000000, 0.9510565162951535312, 1.000000000000000000, 0.9510565162951535312, 1.000000000000000000, 0.9510565162951535312, 1.000000000000000000, 0.9510565162951535312, 1.000000000000000000, 0.9510565162951535312, 1.000000000000000000, 0.9510565162951535312, 1.000000000000000000, 0.9510565162951535312, 1.000000000000000000, 0.9510565162951535312, 1.000000000000000000, 0.9510565162951535312, 1.000000000000000000, 0.9510565162951535312, 1.000000000000000000, 0.9510565162951535312, 1.000000000000000000, 0.9510565162951535312, 1.000000000000000000, 0.9510565162951535312, 1.000000000000000000, 0.9510565162951535312, 1.000000000000000000, 0.9510565162951535312, 1.000000000000000000, 0.9510565162951535312, 1.000000000000000000, 0.9510565162951535312, 1.000000000000000000, 0.9510565162951535312, 1.000000000000000000, 0.9510565162951535312, 1.000000000000000000, 0.9510565162951535312, 1.000000000000000000, 0.9510565162951535312, 1.000000000000000000, 0.9510565162951535312, 1.000000000000000000, 0.9510565162951535312, 1.000000000000000000, 0.9510565162951535312, 1.000000000000000000, 0.9510565162951535312, 1.000000000000000000, 0.9510565162951535312, 1.000000000000000000, 0.9510565162951535312, 1.000000000000000000, 0.9510565162951535312, 1.000000000000000000, 0.9510565162951535312, 1.000000000000000000, 0.9510565162951535312, 1.000000000000000000, 0.9510565162951535312, 1.000000000000000000, 0.9510565162951535312, 1.000000000000000000, 0.9510565162951535312, 1.000000000000000000, 0.9510565162951535312, 1.000000000000000000, 0.9510565162951535312, 1.000000000000000000, 0.9510565162951535312, 1.000000000000000000, 0.9510565162951535312, 1.000000000000000000, 0.9510565162951535312, 1.000000000000000000, 0.9510565162951535312, 1.000000000000000000, 0.9510565162951535312, 1.000000000000000000, 0.9510565162951535312, 1.000000000000000000, 0.9510565162951535312, 1.000000000000000000, 0.9510565162951535312, 1.000000000000000000, 0.9510565162951535312, 1.000000000000000000, 0.9510565162951535312, 1.000000000000000000, 0.9510565162951535312, 1.000000000000000000, 0.9510565162951535312, 1.000000000000000000, 0.9510565162951535312, 1.000000000000000000, 0.9510565162951535312, 1.000000000000000000, 0.9510565162951535312, 1.000000000000000000, 0.9510565162951535312, 1.000000000000000000, 0.9510565162951535312, 1.000000000000000000, 0.9510565162951535312, 1.000000000000000000, 0.9510565162951535312, 1.000000000000000000, 0.9510565162951535312, 1.000000000000000000, 0.9510565162951535312, 1.000000000000000000, 0.9510565162951535312, 1.000000000000000000, 0.9510565162951535312, 1.000000000000000000, 0.9510565162951535312, 1.000000000000000000, 0.9510565162951535312, 1.000000000000000000, 0.9510565162951535312, 1.000000000000000000, 0.9510565162951535312, 1.000000000000000000, 0.9510565162951535312, 1.000000000000000000, 0.9510565162951535312, 1.000000000000000000, 0.9510565162951535312, 1.000000000000000000, 0.9510565162951535312, 1.000000000000000000, 0.9510565162951535312, 1.000000000000000000, 0.9510565162951535312, 1.000000000000000000, 0.9510565162951535312, 1.000000000000000000, 0.9510565162951535312, 1.000000000000000000, 0.9510565162951535312, 1.000000000000000000, 0.9510565162951535312, 1.000000000000000000, 0.9510565162951535312, 1.000000000000000000, 0.9510565162951535312, 1.000000000000000000, 0.9510565162951535312, 1.000000000000000000, 0.9510565162951535312, 1.000000000000000000, 0.9510565162951535312, 1.000000000000000000, 0.9510565162951535312, 1.000000000000000000, 0.9510565162951535312, 1.000000000000000000, 0.9510565162951535312, 1.000000000000000000, 0.9510565162951535312, 1.000000000000000000, 0.9510565162951535312, 1.000000000000000000, 0.9510565162951535312, 1.000000000000000000, 0.9510565162951535312, 1.000000000000000000, 0.9510565162951535312, 1.000000000000000000, 0.9510565162951535312, 1.000000000000000000, 0.9510565162951535312, 1.000000000000000000, 0.9510565162951535312, 1.000000000000000000, 0.9510565162951535312, 1.000000000000000000, 0.9510565162951535312, 1.000000000000000000, 0.9510565162951535312, 1.000000000000000000, 0.9510565162951535312, 1.000000000000000000, 0.9510565162951535312, 1.000000000000000000, 0.9510565162951535312, 1.000000000000000000, 0.9510565162951535312, 1.000000000000000000, 0.9510565162951535312, 1.000000000000000000, 0.9510565162951535312, 1.000000000000000000, 0.9510565162951535312, 1.000000000000000000, 0.9510565162951535312, 1.000000000000000000, 0.9510565162951535312, 1.000000000000000000, 0.9510565162951535312, 1.000000000000000000, 0.9510565162951535312, 1.000000000000000000, 0.9510565162951535312, 1.000000000000000000, 0.9510565162951535312, 1.000000000000000000, 0.9510565162951535312, 1.000000000000000000, 0.9510565162951535312, 1.000000000000000000, 0.9510565162951535312, 1.000000000000000000, 0.9510565162951535312, 1.000000000000000000, 0.9510565162951535312, 1.000000000000000000, 0.9510565162951535312, 1.000000000000000000, 0.9510565162951535312, 1.000000000000000000, 0.9510565162951535312, 1.000000000000000000, 0.9510565162951535312, 1.000000000000000000, 0.9510565162951535312, 1.000000000000000000, 0.9510565162951535312, 1.000000000000000000, 0.9510565162951535312, 1.000000000000000000, 0.9510565162951535312, 1.000000000000000000, 0.9510565162951535312, 1.000000000000000000, 0.9510565162951535312, 1.000000000000000000, 0.9510565162951535312, 1.000000000000000000, 0.9510565162951535312, 1.000000000000000000, 0.9510565162951535312, 1.000000000000000000, 0.9510565162951535312, 1.000000000000000000, 0.9510565162951535312, 1.000000000000000000, 0.9510565162951535312, 1.000000000000000000, 0.9510565162951535312, 1.000000000000000000, 0.9510565162951535312, 1.000000000000000000, 0.9510565162951535312, 1.000000000000000000, 0.9510565162951535312, 1.000000000000000000, 0.9510565162951535312, 1.000000000000000000, 0.9510565162951535312, 1.000000000000000000, 0.9510565162951535312, 1.000000000000000000, 0.9510565162951535312, 1.000000000000000000, 0.9510565162951535312, 1.000000000000000000, 0.9510565162951535312, 1.000000000000000000, 0.9510565162951535312, 1.000000000000000000, 0.9510565162951535312, 1.000000000000000000, 0.9510565162951535312, 1.000000000000000000, 0.9510565162951535312, 1.000000000000000000, 0.9510565162951535312, 1.000000000000000000, 0.9510565162951535312, 1.000000000000000000, 0.9510565162951535312, 1.000000000000000000, 0.9510565162951535312, 1.000000000000000000, 0.9510565162951535312, 1.000000000000000000, 0.9510565162951535312, 1.000000000000000000, 0.9510565162951535312, 1.000000000000000000, 0.9510565162951535312, 1.000000000000000000, 0.9510565162951535312, 1.000000000000000000, 0.9510565162951535312, 1.000000000000000000, 0.9510565162951535312, 1.000000000000000000, 0.9510565162951535312, 1.000000000000000000, 0.9510565162951535312, 1.000000000000000000, 0.9510565162951535312, 1.000000000000000000, 0.9510565162951535312, 1.000000000000000000, 0.9510565162951535312, 1.000000000000000000, 0.9510565162951535312, 1.000000000000000000, 0.9510565162951535312, 1.000000000000000000, 0.9510565162951535312, 1.000000000000000000, 0.9510565162951535312, 1.000000000000000000, 0.9510565162951535312, 1.000000000000000000, 0.9510565162951535312, 1.000000000000000000, 0.9510565162951535312, 1.000000000000000000, 0.9510565162951535312, 1.000000000000000000, 0.9510565162951535312, 1.000000000000000000, 0.9510565162951535312, 1.000000000000000000, 0.9510565162951535312, 1.000000000000000000, 0.9510565162951535312, 1.000000000000000000, 1.000000000000000000, 1.000000000000000000) ) ) 
 REPRESENTATION_ITEM ( '' )  SURFACE ( )  );
#21390=CARTESIAN_POINT ( 'NONE',  ( 4.984841277089891776, 200.2242689037093726, 58.44886208192144039 ) ) ;
#21400=CARTESIAN_POINT ( 'NONE',  ( -2.426778023690262742, 214.6231898156240163, 73.10113791807857808 ) ) ;
#21407=CARTESIAN_POINT ( 'NONE',  ( -2.517493886309087880, 214.5937144450984135, 42.09886208192144608 ) ) ;
#21408=CARTESIAN_POINT ( 'NONE',  ( 6.139770520408368348, 198.4640165459539674, 80.45113791807857240 ) ) ;
#21409=CARTESIAN_POINT ( 'NONE',  ( -3.135527875058821579, 197.5041725223112223, 65.90113791807857524 ) ) ;
#21411=CARTESIAN_POINT ( 'NONE',  ( 6.500168698208129925, 211.6636982574063381, 25.70113791807857240 ) ) ;
#21414=DIRECTION ( 'NONE',  ( 0.3362851123284906207, 0.04491457122451913281, 0.9406885799869860731 ) ) ;
#21416=CARTESIAN_POINT ( 'NONE',  ( 0.05014649552807549926, 219.6175466908591716, 46.25113791807856956 ) ) ;
#21419=CARTESIAN_POINT ( 'NONE',  ( 9.984503880673470277, 203.7031108863295401, 95.15113791807854682 ) ) ;
#21420=CARTESIAN_POINT ( 'NONE',  ( -3.044812012440131443, 216.5253028482142952, 64.10113791807857808 ) ) ;
#21421=CARTESIAN_POINT ( 'NONE',  ( -7.456977232089471386, 217.1783343296987709, 29.94886208192143684 ) ) ;
#21422=CARTESIAN_POINT ( 'NONE',  ( 9.984503880673420539, 210.2968891136705736, 42.84886208192143897 ) ) ;
#21424=CARTESIAN_POINT ( 'NONE',  ( 9.736236675707914401, 214.0148392665762458, 76.70113791807857240 ) ) ;
#21425=CARTESIAN_POINT ( 'NONE',  ( 2.517493886308900919, 214.5937144450984420, 88.40113791807857524 ) ) ;
#21427=CARTESIAN_POINT ( 'NONE',  ( 8.062137200540822946, 212.9164362838583315, 45.69886208192143329 ) ) ;
#21430=CARTESIAN_POINT ( 'NONE',  ( -12.00000000000000711, 206.9523078486584780, 59.49886208192143044 ) ) ;
#21433=CARTESIAN_POINT ( 'NONE',  ( -7.984503880673422316, 204.3529502787951628, 29.34886208192143897 ) ) ;
#21440=CARTESIAN_POINT ( 'NONE',  ( -8.015496119326531499, 204.4483345814780364, 51.35113791807857098 ) ) ;
#21444=CARTESIAN_POINT ( 'NONE',  ( 3.044812012439969795, 216.5253028482143520, 33.39886208192143613 ) ) ;
#21449=CARTESIAN_POINT ( 'NONE',  ( 0.05014649552828262524, 198.5883022060938572, 13.74886208192143577 ) ) ;
#21450=CARTESIAN_POINT ( 'NONE',  ( 10.01549611932653860, 210.2015048109876716, 55.85113791807857808 ) ) ;
#21452=CARTESIAN_POINT ( 'NONE',  ( 6.220909254589536808, 215.4770327129947702, 40.55113791807855250 ) ) ;
#21456=CARTESIAN_POINT ( 'NONE',  ( 2.517493886309087436, 199.4062855549015865, 88.59886208192143897 ) ) ;
#21460=CARTESIAN_POINT ( 'NONE',  ( -12.01549611932652972, 203.1486557965464499, 24.35113791807856742 ) ) ;
#21463=CARTESIAN_POINT ( 'NONE',  ( 8.118202686958039038, 212.8392687619912635, 70.70113791807857240 ) ) ;
#21464=CARTESIAN_POINT ( 'NONE',  ( -9.984503880673475606, 210.2968891136704315, 42.65113791807856813 ) ) ;
#21467=CARTESIAN_POINT ( 'NONE',  ( -8.118202686958138514, 212.8392687619910930, 11.79886208192143471 ) ) ;
#21470=CARTESIAN_POINT ( 'NONE',  ( -12.01549611932652972, 203.1486557965464499, 45.35113791807857098 ) ) ;
#21472=CARTESIAN_POINT ( 'NONE',  ( 3.135527875058981895, 197.5041725223112792, 19.59886208192143542 ) ) ;
#21476=CARTESIAN_POINT ( 'NONE',  ( 9.984503880673470277, 203.7031108863295401, 83.15113791807853261 ) ) ;
#21478=EDGE_CURVE ( 'NONE', #31012, #20137, #12926, .T. ) ;
#21482=CARTESIAN_POINT ( 'NONE',  ( 4.984841277089725686, 213.7757310962907411, 22.55113791807857027 ) ) ;
#21484=CARTESIAN_POINT ( 'NONE',  ( -12.10169002831357510, 232.5389149829038331, 105.4832055762867782 ) ) ;
#21491=CARTESIAN_POINT ( 'NONE',  ( -3.044812012439970683, 197.4746971517856196, 79.89886208192143613 ) ) ;
#21493=CARTESIAN_POINT ( 'NONE',  ( 9.984503880673470277, 203.7031108863295401, 23.15113791807856813 ) ) ;
#21494=CARTESIAN_POINT ( 'NONE',  ( -12.00000000000000711, 206.9523078486584780, 77.49886208192144466 ) ) ;
#21498=CARTESIAN_POINT ( 'NONE',  ( 0.05014649552810505201, 217.5146222423826714, 94.25113791807855534 ) ) ;
#21501=CARTESIAN_POINT ( 'NONE',  ( -6.139770520408369237, 215.5359834540460042, 39.95113791807857240 ) ) ;
#21506=CARTESIAN_POINT ( 'NONE',  ( -3.662846001190052991, 218.4274158808045740, 7.101137918078566535 ) ) ;
#21511=CARTESIAN_POINT ( 'NONE',  ( 3.044812012439969795, 216.5253028482143520, 93.39886208192143613 ) ) ;
#21512=CARTESIAN_POINT ( 'NONE',  ( -7.375838497908014268, 196.7627149292498530, 29.04886208192143471 ) ) ;
#21513=CARTESIAN_POINT ( 'NONE',  ( -10.40947905833197673, 207.8831653815483662, 102.6241284678525432 ) ) ;
#21514=CARTESIAN_POINT ( 'NONE',  ( 8.062137200540920645, 201.0835637161417822, 56.30113791807857382 ) ) ;
#21516=CARTESIAN_POINT ( 'NONE',  ( -2.426778023690076225, 199.3768101843759553, 10.89886208192143613 ) ) ;
#21519=CARTESIAN_POINT ( 'NONE',  ( 7.984503880673422316, 209.6470497212048372, 87.84886208192142476 ) ) ;
#21520=CARTESIAN_POINT ( 'NONE',  ( 2.426778023690261410, 199.3768101843759837, 41.60113791807857808 ) ) ;
#21526=CARTESIAN_POINT ( 'NONE',  ( -8.000000000000008882, 207.0476921513413515, 96.50113791807856956 ) ) ;
#21529=CARTESIAN_POINT ( 'NONE',  ( -8.015496119326597224, 209.5516654185217362, 71.64886208192143613 ) ) ;
#21533=CARTESIAN_POINT ( 'NONE',  ( -0.05014649552810635652, 196.4853777576173002, 8.751137918078567779 ) ) ;
#21537=CARTESIAN_POINT ( 'NONE',  ( 7.375838497908181246, 196.7627149292499666, 80.45113791807857240 ) ) ;
#21538=CARTESIAN_POINT ( 'NONE',  ( 9.984503880673473830, 203.7031108863295401, 101.1511379180785752 ) ) ;
#21542=CARTESIAN_POINT ( 'NONE',  ( -3.135527875058982783, 216.4958274776886924, 6.098862081921434530 ) ) ;
#21543=CARTESIAN_POINT ( 'NONE',  ( -3.662846001189865142, 195.5725841191952838, 64.89886208192143613 ) ) ;
#21544=CARTESIAN_POINT ( 'NONE',  ( 0.05014649552828275014, 196.4853777576173002, 64.74886208192143044 ) ) ;
#21545=CARTESIAN_POINT ( 'NONE',  ( -7.456977232089471386, 217.1783343296987709, 8.948862081921433287 ) ) ;
#21547=CARTESIAN_POINT ( 'NONE',  ( -9.984503880673473830, 210.2968891136704315, 18.65113791807856813 ) ) ;
#21548=CARTESIAN_POINT ( 'NONE',  ( -10.01549611932659722, 210.2015048109875011, 86.64886208192139350 ) ) ;
#21552=CARTESIAN_POINT ( 'NONE',  ( -8.015496119326597224, 209.5516654185217362, 59.64886208192145034 ) ) ;
#21560=CARTESIAN_POINT ( 'NONE',  ( 6.444103211791042618, 202.2591342207267644, 68.30113791807856671 ) ) ;
#21565=CARTESIAN_POINT ( 'NONE',  ( 8.015496119326595448, 204.4483345814782638, 46.14886208192143613 ) ) ;
#21566=CARTESIAN_POINT ( 'NONE',  ( -6.220909254589537696, 198.5229672870051161, 78.05113791807858092 ) ) ;
#21567=CARTESIAN_POINT ( 'NONE',  ( -9.984503880673473830, 210.2968891136704315, 66.65113791807857524 ) ) ;
#21570=CARTESIAN_POINT ( 'NONE',  ( -4.903702542908602524, 213.8346818373418898, 24.95113791807856884 ) ) ;
#21574=CARTESIAN_POINT ( 'NONE',  ( 9.736236675707914401, 214.0148392665762458, 43.70113791807857240 ) ) ;
#21575=FACE_OUTER_BOUND ( 'NONE', #11209, .T. ) ;
#21576=CARTESIAN_POINT ( 'NONE',  ( -6.220909254589537696, 198.5229672870051161, 96.05113791807858092 ) ) ;
#21577=CARTESIAN_POINT ( 'NONE',  ( 8.062137200540920645, 201.0835637161417822, 71.30113791807856671 ) ) ;
#21578=CARTESIAN_POINT ( 'NONE',  ( -9.680171189290716072, 199.9079932115567146, 32.19886208192144039 ) ) ;
#21579=CARTESIAN_POINT ( 'NONE',  ( 8.118202686958138514, 201.1607312380088501, 37.29886208192143471 ) ) ;
#21581=CARTESIAN_POINT ( 'NONE',  ( 7.375838497908181246, 196.7627149292499666, 80.45113791807857240 ) ) ;
#21583=CARTESIAN_POINT ( 'NONE',  ( -8.015496119326531499, 204.4483345814780364, 102.3511379180785639 ) ) ;
#21585=CARTESIAN_POINT ( 'NONE',  ( -3.044812012439970683, 197.4746971517856196, 49.89886208192143613 ) ) ;
#21589=CARTESIAN_POINT ( 'NONE',  ( 7.375838497908012492, 217.2372850707501186, 66.54886208192144181 ) ) ;
#21592=CARTESIAN_POINT ( 'NONE',  ( 6.500168698208244500, 202.3363017425938324, 28.29886208192143826 ) ) ;
#21599=CARTESIAN_POINT ( 'NONE',  ( 4.903702542908601636, 200.1653181626581102, 56.45113791807857950 ) ) ;
#21600=CARTESIAN_POINT ( 'NONE',  ( -9.984503880673420539, 203.7031108863293980, 29.34886208192144252 ) ) ;
#21607=CARTESIAN_POINT ( 'NONE',  ( -7.984503880673422316, 204.3529502787951628, 11.34886208192143542 ) ) ;
#21609=CARTESIAN_POINT ( 'NONE',  ( -8.062137200540920645, 212.9164362838581894, 48.80113791807857382 ) ) ;
#21611=CARTESIAN_POINT ( 'NONE',  ( 8.118202686958039038, 212.8392687619912635, 37.70113791807857240 ) ) ;
#21615=CARTESIAN_POINT ( 'NONE',  ( -8.000000000000008882, 206.9523078486584780, 104.4988620819214304 ) ) ;
#21619=CARTESIAN_POINT ( 'NONE',  ( -9.736236675707914401, 199.9851607334237542, 21.20113791807856529 ) ) ;
#21623=CARTESIAN_POINT ( 'NONE',  ( 9.984503880673470277, 203.7031108863295401, 65.15113791807856103 ) ) ;
#21624=CARTESIAN_POINT ( 'NONE',  ( -3.044812012440131443, 216.5253028482142952, 40.10113791807857098 ) ) ;
#21628=CARTESIAN_POINT ( 'NONE',  ( 3.753561863808876797, 195.6020594897209719, 1.598862081921433864 ) ) ;
#21629=CARTESIAN_POINT ( 'NONE',  ( -8.062137200540822946, 201.0835637161416400, 8.198862081921435063 ) ) ;
#21632=CARTESIAN_POINT ( 'NONE',  ( 3.662846001190051659, 195.5725841191953691, 47.60113791807857808 ) ) ;
#21634=CARTESIAN_POINT ( 'NONE',  ( 9.379977934355958169, 208.8253170565643302, -1.014254689207424676 ) ) ;
#21635=CARTESIAN_POINT ( 'NONE',  ( -8.062137200540822946, 201.0835637161416400, 20.19886208192143684 ) ) ;
#21638=CARTESIAN_POINT ( 'NONE',  ( -0.05014649552810635652, 196.4853777576173002, 77.75113791807856956 ) ) ;
#21644=EDGE_LOOP ( 'NONE', ( #19585, #5177, #23785, #2, #6331 ) ) ;
#21645=CARTESIAN_POINT ( 'NONE',  ( -6.444103211791042618, 211.7408657792732356, 18.80113791807856671 ) ) ;
#21647=CARTESIAN_POINT ( 'NONE',  ( 10.00000000000000711, 207.0476921513415220, 3.998862081921434442 ) ) ;
#21654=CARTESIAN_POINT ( 'NONE',  ( 6.139770520408223575, 215.5359834540460611, 87.54886208192142760 ) ) ;
#21656=CARTESIAN_POINT ( 'NONE',  ( -0.05014649552810635652, 196.4853777576173002, 26.75113791807856956 ) ) ;
#21660=CARTESIAN_POINT ( 'NONE',  ( -11.98450388067341876, 203.0532714938636047, 80.34886208192143897 ) ) ;
#21664=CARTESIAN_POINT ( 'NONE',  ( 3.044812012440130555, 197.4746971517856764, 95.60113791807857808 ) ) ;
#21670=CARTESIAN_POINT ( 'NONE',  ( 6.139770520408368348, 198.4640165459539674, 35.45113791807857240 ) ) ;
#21676=CARTESIAN_POINT ( 'NONE',  ( 11.98450388067348271, 203.0532714938637753, 20.15113791807856458 ) ) ;
#21677=EDGE_CURVE ( 'NONE', #6436, #17153, #31951, .T. ) ;
#21682=CARTESIAN_POINT ( 'NONE',  ( 11.98450388067341876, 210.9467285061363953, 33.84886208192142476 ) ) ;
#21684=CARTESIAN_POINT ( 'NONE',  ( -3.135527875058821579, 197.5041725223112223, 50.90113791807856813 ) ) ;
#21686=CARTESIAN_POINT ( 'NONE',  ( 7.984503880673422316, 209.6470497212048372, 12.84886208192143719 ) ) ;
#21689=CARTESIAN_POINT ( 'NONE',  ( -4.903702542908436435, 200.1653181626580249, 104.0488620819214560 ) ) ;
#21691=CARTESIAN_POINT ( 'NONE',  ( -4.984841277089726574, 200.2242689037092305, 39.05113791807855961 ) ) ;
#21696=CARTESIAN_POINT ( 'NONE',  ( 3.135527875058981895, 197.5041725223112792, 61.59886208192143897 ) ) ;
#21699=CARTESIAN_POINT ( 'NONE',  ( -7.949154985843430055, 215.5765611960900117, 102.9933096652613642 ) ) ;
#21702=CARTESIAN_POINT ( 'NONE',  ( -6.500168698208244500, 211.6636982574061676, 74.79886208192142760 ) ) ;
#21705=CARTESIAN_POINT ( 'NONE',  ( 8.062137200540920645, 201.0835637161417822, 8.301137918078566713 ) ) ;
#21710=CARTESIAN_POINT ( 'NONE',  ( 0.05014649552807549926, 219.6175466908591716, 79.25113791807856956 ) ) ;
#21712=CARTESIAN_POINT ( 'NONE',  ( -3.135527875058821579, 197.5041725223112223, 101.9011379180785752 ) ) ;
#21715=CARTESIAN_POINT ( 'NONE',  ( -3.662846001189865142, 195.5725841191952838, 103.8988620819214361 ) ) ;
#21716=CARTESIAN_POINT ( 'NONE',  ( -11.98450388067341876, 203.0532714938636047, 65.34886208192142476 ) ) ;
#21717=CARTESIAN_POINT ( 'NONE',  ( -6.139770520408224463, 198.4640165459539105, 71.04886208192141339 ) ) ;
#21718=CARTESIAN_POINT ( 'NONE',  ( 3.753561863808876797, 195.6020594897209719, 7.598862081921434530 ) ) ;
#21720=CARTESIAN_POINT ( 'NONE',  ( -8.118202686958039038, 201.1607312380087080, 27.20113791807856884 ) ) ;
#21721=CARTESIAN_POINT ( 'NONE',  ( 10.00000000000000711, 207.0476921513415220, 84.99886208192143044 ) ) ;
#21726=CARTESIAN_POINT ( 'NONE',  ( 4.903702542908435547, 213.8346818373419751, 72.54886208192141339 ) ) ;
#21734=CARTESIAN_POINT ( 'NONE',  ( -8.000000000000008882, 207.0476921513413515, 66.50113791807856956 ) ) ;
#21738=CARTESIAN_POINT ( 'NONE',  ( -2.426778023690076225, 199.3768101843759553, 46.89886208192144323 ) ) ;
#21739=CARTESIAN_POINT ( 'NONE',  ( 0.05014649552810505201, 217.5146222423826714, 85.25113791807854113 ) ) ;
#21740=CARTESIAN_POINT ( 'NONE',  ( -0.05014649552810635652, 196.4853777576173002, 65.75113791807856956 ) ) ;
#21742=CARTESIAN_POINT ( 'NONE',  ( 0.05014649552807626948, 215.4116977939061144, 25.25113791807856956 ) ) ;
#21746=CARTESIAN_POINT ( 'NONE',  ( -12.01549611932652972, 203.1486557965464499, 51.35113791807857098 ) ) ;
#21748=CARTESIAN_POINT ( 'NONE',  ( 6.220909254589536808, 215.4770327129947702, 97.55113791807855250 ) ) ;
#21750=CARTESIAN_POINT ( 'NONE',  ( -10.00000000000000711, 207.0476921513413515, 72.50113791807858377 ) ) ;
#21751=CARTESIAN_POINT ( 'NONE',  ( -12.01549611932659722, 210.8513442034533227, 35.64886208192142902 ) ) ;
#21752=CARTESIAN_POINT ( 'NONE',  ( 10.01549611932659367, 203.7984951890124421, 40.14886208192143613 ) ) ;
#21754=CARTESIAN_POINT ( 'NONE',  ( -3.753561863808691168, 195.6020594897209435, 77.90113791807856103 ) ) ;
#21755=CARTESIAN_POINT ( 'NONE',  ( 6.500168698208129925, 211.6636982574063381, 94.70113791807858661 ) ) ;
#21756=CARTESIAN_POINT ( 'NONE',  ( -6.220909254589682469, 215.4770327129946850, 59.94886208192141908 ) ) ;
#21759=CARTESIAN_POINT ( 'NONE',  ( 11.98450388067341876, 210.9467285061363953, 60.84886208192143187 ) ) ;
#21762=CARTESIAN_POINT ( 'NONE',  ( -6.444103211790928043, 202.2591342207265939, 38.19886208192144750 ) ) ;
#21768=CARTESIAN_POINT ( 'NONE',  ( -6.444103211791042618, 211.7408657792732356, 51.80113791807858092 ) ) ;
#21770=CARTESIAN_POINT ( 'NONE',  ( 6.220909254589681581, 198.5229672870052582, 37.44886208192143329 ) ) ;
#21777=CARTESIAN_POINT ( 'NONE',  ( 7.984503880673422316, 209.6470497212048372, 15.84886208192143719 ) ) ;
#21778=CARTESIAN_POINT ( 'NONE',  ( -9.984503880673473830, 210.2968891136704315, 51.65113791807855392 ) ) ;
#21779=CARTESIAN_POINT ( 'NONE',  ( -0.05014649552810635652, 196.4853777576173002, 41.75113791807855534 ) ) ;
#21782=CARTESIAN_POINT ( 'NONE',  ( -2.517493886309087880, 214.5937144450984135, 99.09886208192145318 ) ) ;
#21786=CARTESIAN_POINT ( 'NONE',  ( -3.753561863808691168, 195.6020594897209435, 14.90113791807856636 ) ) ;
#21788=CARTESIAN_POINT ( 'NONE',  ( -0.05014649552810635652, 196.4853777576173002, 68.75113791807855534 ) ) ;
#21790=CARTESIAN_POINT ( 'NONE',  ( 10.00000000000000711, 206.9523078486586201, 38.00113791807857666 ) ) ;
#21793=CARTESIAN_POINT ( 'NONE',  ( 9.680171189290716072, 214.0920067884432854, 6.698862081921434175 ) ) ;
#21794=CARTESIAN_POINT ( 'NONE',  ( -3.135527875058982783, 216.4958274776886924, 6.098862081921434530 ) ) ;
#21797=CARTESIAN_POINT ( 'NONE',  ( 11.98450388067348271, 203.0532714938637753, 47.15113791807857524 ) ) ;
#21798=CARTESIAN_POINT ( 'NONE',  ( 7.984503880673485376, 204.3529502787953902, 68.15113791807856103 ) ) ;
#21800=CARTESIAN_POINT ( 'NONE',  ( -3.135527875058982783, 216.4958274776886924, 33.09886208192143187 ) ) ;
#21803=CARTESIAN_POINT ( 'NONE',  ( 6.220909254589536808, 215.4770327129947702, 82.55113791807858092 ) ) ;
#21808=CARTESIAN_POINT ( 'NONE',  ( 6.444103211791042618, 202.2591342207267644, 23.30113791807857027 ) ) ;
#21811=CARTESIAN_POINT ( 'NONE',  ( -3.044812012439970683, 197.4746971517856196, 1.898862081921434353 ) ) ;
#21819=CARTESIAN_POINT ( 'NONE',  ( 0.05014649552828275708, 196.4853777576173002, 91.74886208192144466 ) ) ;
#21822=CARTESIAN_POINT ( 'NONE',  ( -9.984503880673473830, 210.2968891136704315, 21.65113791807856458 ) ) ;
#21824=CARTESIAN_POINT ( 'NONE',  ( 3.753561863808876797, 195.6020594897209719, 76.59886208192142476 ) ) ;
#21828=CARTESIAN_POINT ( 'NONE',  ( 6.220909254589536808, 215.4770327129947702, 94.55113791807858092 ) ) ;
#21831=CARTESIAN_POINT ( 'NONE',  ( 8.062137200540920645, 201.0835637161417822, 41.30113791807857382 ) ) ;
#21836=CARTESIAN_POINT ( 'NONE',  ( -9.680171189290831535, 214.0920067884431148, 18.80113791807856671 ) ) ;
#21841=CARTESIAN_POINT ( 'NONE',  ( 3.662846001189864698, 218.4274158808046593, 30.39886208192143613 ) ) ;
#21843=CARTESIAN_POINT ( 'NONE',  ( -3.044812012440131443, 216.5253028482142952, 55.10113791807857098 ) ) ;
#21845=CARTESIAN_POINT ( 'NONE',  ( -2.426778023690076225, 199.3768101843759553, 16.89886208192143613 ) ) ;
#21847=ADVANCED_FACE ( 'NONE', ( #9777 ), #11295, .T. ) ;
#21849=ORIENTED_EDGE ( 'NONE', *, *, #18151, .F. ) ;
#21850=CARTESIAN_POINT ( 'NONE',  ( 0.05014649552828262524, 198.5883022060938572, 100.7488620819214304 ) ) ;
#21853=CARTESIAN_POINT ( 'NONE',  ( 8.015496119326531499, 209.5516654185219636, 37.85113791807857098 ) ) ;
#21857=CARTESIAN_POINT ( 'NONE',  ( 3.044812012439969795, 216.5253028482143520, 63.39886208192144323 ) ) ;
#21861=CARTESIAN_POINT ( 'NONE',  ( -6.444103211791042618, 211.7408657792732356, 96.80113791807858092 ) ) ;
#21864=CARTESIAN_POINT ( 'NONE',  ( -4.984841277089891776, 213.7757310962905990, 71.94886208192144750 ) ) ;
#21868=CARTESIAN_POINT ( 'NONE',  ( -3.044812012440131443, 216.5253028482142952, 10.10113791807856565 ) ) ;
#21874=CARTESIAN_POINT ( 'NONE',  ( 12.01549611932652972, 210.8513442034534933, 79.85113791807857808 ) ) ;
#21875=CARTESIAN_POINT ( 'NONE',  ( 10.01549611932653860, 210.2015048109876716, 94.85113791807857808 ) ) ;
#21878=CARTESIAN_POINT ( 'NONE',  ( -9.736236675708031640, 214.0148392665760753, 101.7988620819214560 ) ) ;
#21879=CARTESIAN_POINT ( 'NONE',  ( -3.753561863808878130, 218.3979405102790281, 57.09886208192143897 ) ) ;
#21880=CARTESIAN_POINT ( 'NONE',  ( 8.118202686958138514, 201.1607312380088501, 79.29886208192144181 ) ) ;
#21881=CARTESIAN_POINT ( 'NONE',  ( -3.662846001189865142, 195.5725841191952838, 4.898862081921434353 ) ) ;
#21883=CARTESIAN_POINT ( 'NONE',  ( 3.135527875058820690, 216.4958274776887492, 22.40113791807856458 ) ) ;
#21884=CARTESIAN_POINT ( 'NONE',  ( -6.139770520408224463, 198.4640165459539389, 92.04886208192139918 ) ) ;
#21891=CARTESIAN_POINT ( 'NONE',  ( 0.05014649552828262524, 198.5883022060938572, 67.74886208192143044 ) ) ;
#21899=CARTESIAN_POINT ( 'NONE',  ( -4.903702542908602524, 213.8346818373418898, 69.95113791807858661 ) ) ;
#21903=CARTESIAN_POINT ( 'NONE',  ( 6.500168698208244500, 202.3363017425938324, 43.29886208192144181 ) ) ;
#21904=CARTESIAN_POINT ( 'NONE',  ( 3.044812012440130555, 197.4746971517856764, 86.60113791807857808 ) ) ;
#21905=CARTESIAN_POINT ( 'NONE',  ( 3.135527875058820690, 216.4958274776887492, 70.40113791807857524 ) ) ;
#21911=CARTESIAN_POINT ( 'NONE',  ( -7.456977232089304408, 196.8216656703010301, 45.05113791807857382 ) ) ;
#21914=CARTESIAN_POINT ( 'NONE',  ( -3.135527875058821579, 197.5041725223112223, 95.90113791807858945 ) ) ;
#21915=CARTESIAN_POINT ( 'NONE',  ( -3.135527875058821579, 197.5041725223112223, 68.90113791807857524 ) ) ;
#21916=CARTESIAN_POINT ( 'NONE',  ( -9.680171189290716072, 199.9079932115567146, 29.19886208192143684 ) ) ;
#21917=CARTESIAN_POINT ( 'NONE',  ( 3.044812012439969795, 216.5253028482143520, 39.39886208192143613 ) ) ;
#21920=CARTESIAN_POINT ( 'NONE',  ( -11.98450388067348804, 210.9467285061362247, 75.65113791807856103 ) ) ;
#21921=CARTESIAN_POINT ( 'NONE',  ( -7.984503880673488041, 209.6470497212046098, 96.65113791807858945 ) ) ;
#21923=CARTESIAN_POINT ( 'NONE',  ( -8.118202686958138514, 212.8392687619910930, 62.79886208192144181 ) ) ;
#21927=CARTESIAN_POINT ( 'NONE',  ( -11.98450388067341876, 203.0532714938636047, 65.34886208192142476 ) ) ;
#21930=CARTESIAN_POINT ( 'NONE',  ( 4.984841277089891776, 200.2242689037093726, 40.44886208192144750 ) ) ;
#21936=CARTESIAN_POINT ( 'NONE',  ( -7.984503880673488041, 209.6470497212046098, 54.65113791807857524 ) ) ;
#21940=CARTESIAN_POINT ( 'NONE',  ( -9.984503880673420539, 203.7031108863293980, 32.34886208192143187 ) ) ;
#21948=CARTESIAN_POINT ( 'NONE',  ( -0.05014649552828365914, 215.4116977939061144, 18.24886208192143755 ) ) ;
#21950=CARTESIAN_POINT ( 'NONE',  ( -6.139770520408369237, 215.5359834540460042, 57.95113791807856529 ) ) ;
#21951=CARTESIAN_POINT ( 'NONE',  ( 6.139770520408368348, 198.4640165459539674, 41.45113791807857240 ) ) ;
#21954=CARTESIAN_POINT ( 'NONE',  ( 2.517493886309087436, 199.4062855549015865, 97.59886208192145318 ) ) ;
#21959=CARTESIAN_POINT ( 'NONE',  ( -12.00000000000000711, 207.0476921513413515, 18.50113791807856956 ) ) ;
#21961=CARTESIAN_POINT ( 'NONE',  ( 8.118202686958039038, 212.8392687619912635, 64.70113791807857240 ) ) ;
#21962=CARTESIAN_POINT ( 'NONE',  ( -10.00000000000000711, 207.0476921513413515, 39.50113791807856956 ) ) ;
#21965=CARTESIAN_POINT ( 'NONE',  ( -10.00000000000000178, 206.7692714347156198, 108.3323677711372000 ) ) ;
#21966=CARTESIAN_POINT ( 'NONE',  ( -3.662846001189865142, 195.5725841191952838, 7.898862081921435241 ) ) ;
#21967=CARTESIAN_POINT ( 'NONE',  ( -6.220909254589682469, 215.4770327129947134, 5.948862081921435063 ) ) ;
#21970=CARTESIAN_POINT ( 'NONE',  ( 9.736236675707914401, 214.0148392665762458, 52.70113791807856529 ) ) ;
#21971=CARTESIAN_POINT ( 'NONE',  ( -4.984841277089726574, 200.2242689037092305, 69.05113791807856671 ) ) ;
#21973=CARTESIAN_POINT ( 'NONE',  ( 3.044812012439969795, 216.5253028482143520, 27.39886208192143613 ) ) ;
#21975=SHAPE_REPRESENTATION ( 'spring', ( #2404 ), #11135 ) ;
#21977=CARTESIAN_POINT ( 'NONE',  ( -3.044812012440131443, 216.5253028482142952, 79.10113791807857808 ) ) ;
#21982=CARTESIAN_POINT ( 'NONE',  ( -2.517493886308901807, 199.4062855549015012, 20.90113791807856813 ) ) ;
#21985=CARTESIAN_POINT ( 'NONE',  ( -0.05014649552828403384, 217.5146222423826714, 6.248862081921433109 ) ) ;
#21989=CARTESIAN_POINT ( 'NONE',  ( -8.015496119326531499, 204.4483345814780364, 48.35113791807857098 ) ) ;
#21994=CARTESIAN_POINT ( 'NONE',  ( -3.135527875058982783, 216.4958274776886924, 93.09886208192145318 ) ) ;
#21996=CARTESIAN_POINT ( 'NONE',  ( 8.118202686958039038, 212.8392687619912635, 34.70113791807857240 ) ) ;
#21998=CARTESIAN_POINT ( 'NONE',  ( -9.680171189290716072, 199.9079932115567146, 83.19886208192144750 ) ) ;
#22004=CARTESIAN_POINT ( 'NONE',  ( 3.135527875058820690, 216.4958274776887492, 91.40113791807857524 ) ) ;
#22007=CARTESIAN_POINT ( 'NONE',  ( -6.220909254589537696, 198.5229672870051161, 33.05113791807857382 ) ) ;
#22013=CARTESIAN_POINT ( 'NONE',  ( -7.375838497908182134, 217.2372850707499765, 15.95113791807856707 ) ) ;
#22017=CARTESIAN_POINT ( 'NONE',  ( -11.98450388067341876, 203.0532714938636047, 38.34886208192142476 ) ) ;
#22018=CARTESIAN_POINT ( 'NONE',  ( 6.139770520408368348, 198.4640165459539674, 2.451137918078566180 ) ) ;
#22019=CARTESIAN_POINT ( 'NONE',  ( 6.220909254589536808, 215.4770327129947702, 55.55113791807855961 ) ) ;
#22021=CARTESIAN_POINT ( 'NONE',  ( 6.500168698208244500, 202.3363017425938324, 10.29886208192143471 ) ) ;
#22025=CARTESIAN_POINT ( 'NONE',  ( -0.05014649552828365914, 215.4116977939061144, 102.2488620819214447 ) ) ;
#22028=CARTESIAN_POINT ( 'NONE',  ( 8.000000000000008882, 206.9523078486586485, 44.00113791807857666 ) ) ;
#22033=CARTESIAN_POINT ( 'NONE',  ( 0.05014649552828275708, 196.4853777576173002, 64.74886208192143044 ) ) ;
#22035=DIRECTION ( 'NONE',  ( 0.000000000000000000, -0.04769215134145524809, -0.9988620819214351076 ) ) ;
#22036=CARTESIAN_POINT ( 'NONE',  ( -7.984503880673488041, 209.6470497212046098, 99.65113791807858945 ) ) ;
#22039=CARTESIAN_POINT ( 'NONE',  ( 8.015496119326595448, 204.4483345814782638, 82.14886208192143613 ) ) ;
#22044=CARTESIAN_POINT ( 'NONE',  ( 3.044812012440130555, 197.4746971517856764, 20.60113791807856742 ) ) ;
#22048=CARTESIAN_POINT ( 'NONE',  ( 11.98450388067348271, 203.0532714938637753, 86.15113791807856103 ) ) ;
#22052=EDGE_LOOP ( 'NONE', ( #8484, #27040, #9501, #871, #5995 ) ) ;
#22053=CARTESIAN_POINT ( 'NONE',  ( 9.680171189290716072, 214.0920067884432854, 57.69886208192144039 ) ) ;
#22054=CARTESIAN_POINT ( 'NONE',  ( -0.05014649552828402690, 217.5146222423826714, 72.24886208192143044 ) ) ;
#22055=CARTESIAN_POINT ( 'NONE',  ( 7.375838497908012492, 217.2372850707501186, 9.548862081921432932 ) ) ;
#22057=CARTESIAN_POINT ( 'NONE',  ( -6.139770520408369237, 215.5359834540460042, 21.95113791807856884 ) ) ;
#22059=CARTESIAN_POINT ( 'NONE',  ( -3.135527875058982783, 216.4958274776886924, 90.09886208192143897 ) ) ;
#22061=ORIENTED_EDGE ( 'NONE', *, *, #164, .F. ) ;
#22065=CARTESIAN_POINT ( 'NONE',  ( 2.426778023690075337, 214.6231898156240447, 75.39886208192143613 ) ) ;
#22072=CARTESIAN_POINT ( 'NONE',  ( -2.426778023690262742, 214.6231898156240163, 67.10113791807857808 ) ) ;
#22075=CARTESIAN_POINT ( 'NONE',  ( 2.426778023690075337, 214.6231898156240447, 45.39886208192144323 ) ) ;
#22077=CARTESIAN_POINT ( 'NONE',  ( 3.135527875058820690, 216.4958274776887492, 76.40113791807857524 ) ) ;
#22083=CARTESIAN_POINT ( 'NONE',  ( 7.375838497908181246, 196.7627149292499666, 59.45113791807857240 ) ) ;
#22086=CARTESIAN_POINT ( 'NONE',  ( 9.736236675707914401, 214.0148392665762458, 4.701137918078565292 ) ) ;
#22088=CARTESIAN_POINT ( 'NONE',  ( -3.135527875058821579, 197.5041725223112223, 65.90113791807857524 ) ) ;
#22089=CARTESIAN_POINT ( 'NONE',  ( 12.00000000000000711, 207.0476921513415220, 33.99886208192143044 ) ) ;
#22090=CARTESIAN_POINT ( 'NONE',  ( 3.044812012439969795, 216.5253028482143520, 48.39886208192143613 ) ) ;
#22092=CARTESIAN_POINT ( 'NONE',  ( 9.680171189290831535, 199.9079932115568852, 80.30113791807858092 ) ) ;
#22093=CARTESIAN_POINT ( 'NONE',  ( 2.426778023690261410, 199.3768101843759837, 98.60113791807857808 ) ) ;
#22094=CARTESIAN_POINT ( 'NONE',  ( 3.135527875058981895, 197.5041725223112792, 64.59886208192143897 ) ) ;
#22097=CARTESIAN_POINT ( 'NONE',  ( 12.00000000000000711, 207.0476921513415220, 63.99886208192143044 ) ) ;
#22100=CARTESIAN_POINT ( 'NONE',  ( 8.015496119326595448, 204.4483345814782638, 40.14886208192143613 ) ) ;
#22105=CLOSED_SHELL ( 'NONE', ( #33035, #8972, #24585, #14136, #26238, #8564, #27276, #16752, #1253, #18298, #12229, #21847, #26376, #10038, #20969, #11682, #29366, #30567, #14736, #10807 ) ) ;
#22107=CARTESIAN_POINT ( 'NONE',  ( -2.517493886308901807, 199.4062855549015012, 47.90113791807857524 ) ) ;
#22108=CARTESIAN_POINT ( 'NONE',  ( 8.062137200540822946, 212.9164362838583315, 45.69886208192143329 ) ) ;
#22110=ORIENTED_EDGE ( 'NONE', *, *, #7897, .F. ) ;
#22115=CARTESIAN_POINT ( 'NONE',  ( -2.426778023690076225, 199.3768101843759553, 13.89886208192143613 ) ) ;
#22116=CARTESIAN_POINT ( 'NONE',  ( 0.05014649552810505201, 217.5146222423826714, 61.25113791807856245 ) ) ;
#22117=CARTESIAN_POINT ( 'NONE',  ( -10.00000000000000711, 207.0476921513413515, 51.50113791807857666 ) ) ;
#22119=CARTESIAN_POINT ( 'NONE',  ( -8.101690028313589309, 224.0100459381558267, 105.4832055762867782 ) ) ;
#22123=CARTESIAN_POINT ( 'NONE',  ( 3.662846001190051659, 195.5725841191953691, 23.60113791807857098 ) ) ;
#22125=CARTESIAN_POINT ( 'NONE',  ( 3.044812012440130555, 197.4746971517856764, 71.60113791807857808 ) ) ;
#22126=CARTESIAN_POINT ( 'NONE',  ( 8.118202686958039038, 212.8392687619912635, 37.70113791807857240 ) ) ;
#22129=CARTESIAN_POINT ( 'NONE',  ( -7.456977232089471386, 217.1783343296987709, 2.948862081921434175 ) ) ;
#22130=CARTESIAN_POINT ( 'NONE',  ( 8.062137200540822946, 212.9164362838583315, 21.69886208192143684 ) ) ;
#22133=CARTESIAN_POINT ( 'NONE',  ( -9.680171189290831535, 214.0920067884431148, 51.80113791807857382 ) ) ;
#22134=CARTESIAN_POINT ( 'NONE',  ( -0.05014649552807731031, 198.5883022060938572, 65.75113791807856956 ) ) ;
#22135=CARTESIAN_POINT ( 'NONE',  ( 3.135527875058981895, 197.5041725223112792, 31.59886208192143187 ) ) ;
#22139=CARTESIAN_POINT ( 'NONE',  ( -6.220909254589537696, 198.5229672870051161, 87.05113791807856671 ) ) ;
#22144=CARTESIAN_POINT ( 'NONE',  ( -2.426778023690262742, 214.6231898156240163, 25.10113791807856742 ) ) ;
#22148=CARTESIAN_POINT ( 'NONE',  ( -10.01549611932659722, 210.2015048109875011, 5.648862081921435241 ) ) ;
#22151=CARTESIAN_POINT ( 'NONE',  ( -0.05014649552807731031, 198.5883022060938572, 50.75113791807857666 ) ) ;
#22156=CARTESIAN_POINT ( 'NONE',  ( -9.984503880673420539, 203.7031108863293980, 92.34886208192141055 ) ) ;
#22158=CARTESIAN_POINT ( 'NONE',  ( 3.135527875058820690, 216.4958274776887492, 28.40113791807856813 ) ) ;
#22160=CARTESIAN_POINT ( 'NONE',  ( 12.00000000000000711, 207.0476921513415220, 75.99886208192144466 ) ) ;
#22166=CARTESIAN_POINT ( 'NONE',  ( 9.984503880673470277, 203.7031108863295401, 95.15113791807854682 ) ) ;
#22169=CARTESIAN_POINT ( 'NONE',  ( 10.01549611932653860, 210.2015048109876716, 34.85113791807856387 ) ) ;
#22174=ORIENTED_EDGE ( 'NONE', *, *, #7029, .T. ) ;
#22176=CARTESIAN_POINT ( 'NONE',  ( -7.456977232089304408, 196.8216656703010301, 15.05113791807856849 ) ) ;
#22183=CARTESIAN_POINT ( 'NONE',  ( -12.01549611932659722, 210.8513442034533227, 41.64886208192143613 ) ) ;
#22184=CARTESIAN_POINT ( 'NONE',  ( 3.135527875058820690, 216.4958274776887492, 1.401137918078565914 ) ) ;
#22185=CARTESIAN_POINT ( 'NONE',  ( 3.135527875058820690, 216.4958274776887492, 61.40113791807857524 ) ) ;
#22186=CARTESIAN_POINT ( 'NONE',  ( -8.000000000000008882, 206.9523078486584780, 11.49886208192143577 ) ) ;
#22190=CARTESIAN_POINT ( 'NONE',  ( -7.984503880673422316, 204.3529502787951628, 98.34886208192145318 ) ) ;
#22192=CARTESIAN_POINT ( 'NONE',  ( -2.426778023690262742, 214.6231898156240163, 40.10113791807857098 ) ) ;
#22199=CARTESIAN_POINT ( 'NONE',  ( -8.062137200540822946, 201.0835637161416400, 59.19886208192144039 ) ) ;
#22202=CARTESIAN_POINT ( 'NONE',  ( -3.135527875058821579, 197.5041725223112223, -0.09886208192143428053 ) ) ;
#22207=CARTESIAN_POINT ( 'NONE',  ( -8.000000000000008882, 206.9523078486584780, 80.49886208192144466 ) ) ;
#22208=CARTESIAN_POINT ( 'NONE',  ( -4.927659837809095222, 206.3103720916592465, -5.504302862921502282 ) ) ;
#22212=CARTESIAN_POINT ( 'NONE',  ( -0.05014649552810635652, 196.4853777576173002, 23.75113791807856245 ) ) ;
#22216=CARTESIAN_POINT ( 'NONE',  ( -3.753561863808691168, 195.6020594897209435, 86.90113791807857524 ) ) ;
#22220=CARTESIAN_POINT ( 'NONE',  ( 9.736236675708031640, 199.9851607334238963, 70.29886208192142760 ) ) ;
#22221=CARTESIAN_POINT ( 'NONE',  ( 8.118202686958138514, 201.1607312380088501, 73.29886208192142760 ) ) ;
#22222=CARTESIAN_POINT ( 'NONE',  ( -12.00000000000000711, 206.9523078486584780, 14.49886208192143577 ) ) ;
#22225=CARTESIAN_POINT ( 'NONE',  ( 6.220909254589536808, 215.4770327129947702, 22.55113791807856671 ) ) ;
#22227=CARTESIAN_POINT ( 'NONE',  ( 3.135527875058981895, 197.5041725223112792, 88.59886208192143897 ) ) ;
#22230=CARTESIAN_POINT ( 'NONE',  ( -1.474514954580286030E-14, 206.9977241638431167, -6.000000000000014211 ) ) ;
#22233=CARTESIAN_POINT ( 'NONE',  ( -8.000000000000008882, 206.9523078486584780, 74.49886208192144466 ) ) ;
#22241=CARTESIAN_POINT ( 'NONE',  ( -8.000000000000008882, 207.0476921513413515, 81.50113791807856956 ) ) ;
#22244=CARTESIAN_POINT ( 'NONE',  ( 2.426778023690075337, 214.6231898156240447, 51.39886208192145745 ) ) ;
#22245=VECTOR ( 'NONE', #3818, 1000.000000000000114 ) ;
#22248=CARTESIAN_POINT ( 'NONE',  ( -6.220909254589537696, 198.5229672870051161, 30.05113791807856671 ) ) ;
#22249=CARTESIAN_POINT ( 'NONE',  ( -0.3755270751584372513, 206.3102596154024297, 117.9458888342408898 ) ) ;
#22254=CARTESIAN_POINT ( 'NONE',  ( -7.375838497908182134, 217.2372850707499765, 54.95113791807855819 ) ) ;
#22256=CARTESIAN_POINT ( 'NONE',  ( 3.135527875058820690, 216.4958274776887492, 100.4011379180785752 ) ) ;
#22257=CARTESIAN_POINT ( 'NONE',  ( 10.00000000000000711, 206.9523078486586201, 80.00113791807856956 ) ) ;
#22258=CIRCLE ( 'NONE', #13557, 0.9999999999999992228 ) ;
#22259=CARTESIAN_POINT ( 'NONE',  ( 0.05014649552828288198, 194.3824533091408000, 40.74886208192143044 ) ) ;
#22260=CARTESIAN_POINT ( 'NONE',  ( -10.00000000000000711, 206.9523078486584495, 47.49886208192143755 ) ) ;
#22262=CARTESIAN_POINT ( 'NONE',  ( -9.680171189290831535, 214.0920067884431148, 90.80113791807858092 ) ) ;
#22263=CARTESIAN_POINT ( 'NONE',  ( -8.015496119326531499, 204.4483345814780364, 99.35113791807857808 ) ) ;
#22264=CARTESIAN_POINT ( 'NONE',  ( 0.05014649552828275708, 196.4853777576173002, 64.74886208192143044 ) ) ;
#22268=CARTESIAN_POINT ( 'NONE',  ( 9.680171189290716072, 214.0920067884432854, 66.69886208192143329 ) ) ;
#22271=CARTESIAN_POINT ( 'NONE',  ( -7.984503880673422316, 204.3529502787951628, 44.34886208192144608 ) ) ;
#22277=LINE ( 'NONE', #6443, #31261 ) ;
#22278=CARTESIAN_POINT ( 'NONE',  ( -6.500168698208129925, 202.3363017425936050, 63.20113791807857240 ) ) ;
#22281=CARTESIAN_POINT ( 'NONE',  ( -9.984503880673420539, 203.7031108863293980, 47.34886208192143187 ) ) ;
#22287=CARTESIAN_POINT ( 'NONE',  ( -7.984503880673422316, 204.3529502787951628, 23.34886208192143542 ) ) ;
#22289=CARTESIAN_POINT ( 'NONE',  ( -10.00000000000000711, 207.0476921513413515, 57.50113791807856956 ) ) ;
#22290=CARTESIAN_POINT ( 'NONE',  ( -8.118202686958039038, 201.1607312380087080, 45.20113791807857240 ) ) ;
#22292=CARTESIAN_POINT ( 'NONE',  ( 10.01549611932653860, 210.2015048109876716, 22.85113791807856742 ) ) ;
#22293=CARTESIAN_POINT ( 'NONE',  ( -7.984503880673422316, 204.3529502787951628, 101.3488620819214390 ) ) ;
#22297=CARTESIAN_POINT ( 'NONE',  ( -12.01549611932652972, 203.1486557965464499, 27.35113791807856742 ) ) ;
#22299=CARTESIAN_POINT ( 'NONE',  ( -9.984503880673473830, 210.2968891136704315, 78.65113791807854682 ) ) ;
#22300=CARTESIAN_POINT ( 'NONE',  ( -3.044812012440131443, 216.5253028482142952, 49.10113791807857808 ) ) ;
#22303=CARTESIAN_POINT ( 'NONE',  ( 9.736236675708031640, 199.9851607334238963, 16.29886208192143471 ) ) ;
#22304=CARTESIAN_POINT ( 'NONE',  ( 8.118202686958138514, 201.1607312380088501, 19.29886208192143471 ) ) ;
#22307=CARTESIAN_POINT ( 'NONE',  ( 7.456977232089302632, 217.1783343296989131, 58.55113791807858092 ) ) ;
#22308=CARTESIAN_POINT ( 'NONE',  ( 2.517493886308900919, 214.5937144450984420, 67.40113791807856103 ) ) ;
#22309=CARTESIAN_POINT ( 'NONE',  ( -6.139770520408224463, 198.4640165459539389, 32.04886208192143471 ) ) ;
#22312=CARTESIAN_POINT ( 'NONE',  ( -10.01549611932653860, 203.7984951890123284, 90.35113791807857808 ) ) ;
#22317=CARTESIAN_POINT ( 'NONE',  ( -0.05014649552807731031, 198.5883022060938572, 32.75113791807856956 ) ) ;
#22319=CARTESIAN_POINT ( 'NONE',  ( 10.01549611932659545, 203.7984951890123853, 16.14886208192143613 ) ) ;
#22322=CARTESIAN_POINT ( 'NONE',  ( 0.05014649552807626948, 215.4116977939061144, 52.25113791807857666 ) ) ;
#22325=CARTESIAN_POINT ( 'NONE',  ( -10.01549611932659722, 210.2015048109875011, 89.64886208192143613 ) ) ;
#22327=CARTESIAN_POINT ( 'NONE',  ( 10.01549611932653860, 210.2015048109876716, 31.85113791807857453 ) ) ;
#22329=CARTESIAN_POINT ( 'NONE',  ( -10.01549611932653860, 203.7984951890123284, 15.35113791807856565 ) ) ;
#22335=CARTESIAN_POINT ( 'NONE',  ( 6.139770520408368348, 198.4640165459539674, 101.4511379180785866 ) ) ;
#22338=CARTESIAN_POINT ( 'NONE',  ( -8.118202686958039038, 201.1607312380087080, 45.20113791807857240 ) ) ;
#22344=CARTESIAN_POINT ( 'NONE',  ( -9.680171189290831535, 214.0920067884431148, 21.80113791807856671 ) ) ;
#22345=CARTESIAN_POINT ( 'NONE',  ( -11.00000000000000355, 207.1715494402557738, 103.3438596442687327 ) ) ;
#22348=CARTESIAN_POINT ( 'NONE',  ( -9.680171189290716072, 199.9079932115567146, 44.19886208192143329 ) ) ;
#22350=CARTESIAN_POINT ( 'NONE',  ( 9.984503880673470277, 203.7031108863295401, 65.15113791807856103 ) ) ;
#22351=CARTESIAN_POINT ( 'NONE',  ( -4.984841277089891776, 213.7757310962905990, 26.94886208192142973 ) ) ;
#22355=CARTESIAN_POINT ( 'NONE',  ( 6.444103211791042618, 202.2591342207267644, 8.301137918078564937 ) ) ;
#22357=CARTESIAN_POINT ( 'NONE',  ( -7.456977232089471386, 217.1783343296987709, 89.94886208192144750 ) ) ;
#22363=CARTESIAN_POINT ( 'NONE',  ( 0.05014649552828275708, 196.4853777576173002, 58.74886208192141623 ) ) ;
#22366=CARTESIAN_POINT ( 'NONE',  ( -3.044812012440131443, 216.5253028482142952, 1.101137918078565869 ) ) ;
#22371=CARTESIAN_POINT ( 'NONE',  ( -2.426778023690076225, 199.3768101843759553, 85.89886208192143613 ) ) ;
#22374=CARTESIAN_POINT ( 'NONE',  ( -12.00000000000000711, 206.9523078486584780, 83.49886208192144466 ) ) ;
#22376=CARTESIAN_POINT ( 'NONE',  ( -3.044812012440131443, 216.5253028482142952, 25.10113791807856742 ) ) ;
#22382=CARTESIAN_POINT ( 'NONE',  ( -0.05014649552807705357, 194.3824533091408000, 83.75113791807856956 ) ) ;
#22385=CARTESIAN_POINT ( 'NONE',  ( -12.00000000000000711, 206.9523078486584780, 74.49886208192144466 ) ) ;
#22386=CARTESIAN_POINT ( 'NONE',  ( -10.01549611932659545, 210.2015048109875011, 74.64886208192142192 ) ) ;
#22387=CARTESIAN_POINT ( 'NONE',  ( -7.456977232089471386, 217.1783343296987709, 17.94886208192143684 ) ) ;
#22389=CARTESIAN_POINT ( 'NONE',  ( -10.01549611932653860, 203.7984951890123284, 36.35113791807857098 ) ) ;
#22391=CARTESIAN_POINT ( 'NONE',  ( -10.01549611932659722, 210.2015048109875011, 98.64886208192143613 ) ) ;
#22395=CARTESIAN_POINT ( 'NONE',  ( 8.015496119326595448, 204.4483345814782638, 67.14886208192143613 ) ) ;
#22403=CARTESIAN_POINT ( 'NONE',  ( -8.015496119326531499, 204.4483345814780364, 81.35113791807857808 ) ) ;
#22409=CARTESIAN_POINT ( 'NONE',  ( -8.000000000000008882, 206.9523078486584780, 56.49886208192145176 ) ) ;
#22417=CARTESIAN_POINT ( 'NONE',  ( 12.00000000000000711, 206.9523078486586485, 62.00113791807856956 ) ) ;
#22419=CARTESIAN_POINT ( 'NONE',  ( -12.01549611932652972, 203.1486557965464499, 0.3511379180785654808 ) ) ;
#22420=CARTESIAN_POINT ( 'NONE',  ( 3.044812012440130555, 197.4746971517856764, 74.60113791807856387 ) ) ;
#22421=CARTESIAN_POINT ( 'NONE',  ( -7.375838497908014268, 196.7627149292498530, 38.04886208192144181 ) ) ;
#22423=CARTESIAN_POINT ( 'NONE',  ( -6.139770520408224463, 198.4640165459539105, 44.04886208192143471 ) ) ;
#22425=CARTESIAN_POINT ( 'NONE',  ( 9.736236675707914401, 214.0148392665762458, 91.70113791807857240 ) ) ;
#22426=CARTESIAN_POINT ( 'NONE',  ( 8.118202686958039038, 212.8392687619912635, 1.701137918078565736 ) ) ;
#22428=CARTESIAN_POINT ( 'NONE',  ( 8.118202686958138514, 201.1607312380088501, 55.29886208192144181 ) ) ;
#22431=CARTESIAN_POINT ( 'NONE',  ( -7.456977232089471386, 217.1783343296987709, 71.94886208192144750 ) ) ;
#22434=CARTESIAN_POINT ( 'NONE',  ( -2.426778023690076225, 199.3768101843759553, 40.89886208192144323 ) ) ;
#22441=CARTESIAN_POINT ( 'NONE',  ( -6.500168698208129925, 202.3363017425936050, 57.20113791807857240 ) ) ;
#22444=CARTESIAN_POINT ( 'NONE',  ( 3.135527875058981895, 197.5041725223112792, 43.59886208192143897 ) ) ;
#22449=CARTESIAN_POINT ( 'NONE',  ( -6.444103211790928043, 202.2591342207265939, 26.19886208192144039 ) ) ;
#22450=CARTESIAN_POINT ( 'NONE',  ( 8.118202686958039038, 212.8392687619912635, 58.70113791807857240 ) ) ;
#22451=CARTESIAN_POINT ( 'NONE',  ( 6.220909254589536808, 215.4770327129947702, 46.55113791807856671 ) ) ;
#22454=CARTESIAN_POINT ( 'NONE',  ( -8.118202686958039038, 201.1607312380087080, 18.20113791807856884 ) ) ;
#22455=CARTESIAN_POINT ( 'NONE',  ( -4.984841277089726574, 200.2242689037092305, 6.051137918078566713 ) ) ;
#22460=CARTESIAN_POINT ( 'NONE',  ( -3.662846001190052991, 218.4274158808045740, 31.10113791807856742 ) ) ;
#22464=CARTESIAN_POINT ( 'NONE',  ( -8.118202686958039038, 201.1607312380087080, 75.20113791807857240 ) ) ;
#22465=CARTESIAN_POINT ( 'NONE',  ( 3.044812012440130555, 197.4746971517856764, 44.60113791807857098 ) ) ;
#22469=CARTESIAN_POINT ( 'NONE',  ( 3.662846001189864698, 218.4274158808046593, 18.39886208192143613 ) ) ;
#22470=CARTESIAN_POINT ( 'NONE',  ( 8.062137200540822946, 212.9164362838583315, 15.69886208192143506 ) ) ;
#22473=CARTESIAN_POINT ( 'NONE',  ( 7.375838497908181246, 196.7627149292499666, 53.45113791807857240 ) ) ;
#22474=CARTESIAN_POINT ( 'NONE',  ( -0.05014649552807731031, 198.5883022060938572, 71.75113791807856956 ) ) ;
#22476=CARTESIAN_POINT ( 'NONE',  ( -3.135527875058982783, 216.4958274776886924, 30.09886208192143897 ) ) ;
#22489=CARTESIAN_POINT ( 'NONE',  ( 6.500168698208129925, 211.6636982574063381, 28.70113791807857240 ) ) ;
#22492=CARTESIAN_POINT ( 'NONE',  ( 9.984503880673420539, 210.2968891136705167, 12.84886208192143187 ) ) ;
#22496=CARTESIAN_POINT ( 'NONE',  ( -8.000000000000008882, 207.0476921513413515, 54.50113791807857666 ) ) ;
#22499=CARTESIAN_POINT ( 'NONE',  ( -8.062137200540822946, 201.0835637161416400, 104.1988620819214475 ) ) ;
#22501=CARTESIAN_POINT ( 'NONE',  ( -6.220909254589537696, 198.5229672870051161, 30.05113791807856671 ) ) ;
#22503=CARTESIAN_POINT ( 'NONE',  ( 10.01549611932653860, 210.2015048109876716, 13.85113791807856742 ) ) ;
#22509=CARTESIAN_POINT ( 'NONE',  ( 10.00000000000000711, 206.9523078486586201, 101.0011379180785696 ) ) ;
#22512=CARTESIAN_POINT ( 'NONE',  ( 9.984503880673470277, 203.7031108863295401, 47.15113791807857524 ) ) ;
#22520=CARTESIAN_POINT ( 'NONE',  ( -9.680171189290831535, 214.0920067884431148, 27.80113791807857027 ) ) ;
#22525=CARTESIAN_POINT ( 'NONE',  ( -8.062137200540822946, 201.0835637161416400, 5.198862081921435063 ) ) ;
#22529=CARTESIAN_POINT ( 'NONE',  ( -6.139770520408369237, 215.5359834540460042, 57.95113791807856529 ) ) ;
#22530=CARTESIAN_POINT ( 'NONE',  ( 2.517493886309087436, 199.4062855549015865, 19.59886208192143897 ) ) ;
#22534=CARTESIAN_POINT ( 'NONE',  ( 2.517493886308900919, 214.5937144450984420, 4.401137918078566358 ) ) ;
#22536=CARTESIAN_POINT ( 'NONE',  ( 9.680171189290716072, 214.0920067884432854, 87.69886208192144750 ) ) ;
#22541=CARTESIAN_POINT ( 'NONE',  ( -3.044812012440131443, 216.5253028482142952, 1.101137918078565869 ) ) ;
#22543=CARTESIAN_POINT ( 'NONE',  ( 6.220909254589681581, 198.5229672870052582, 70.44886208192144750 ) ) ;
#22546=CARTESIAN_POINT ( 'NONE',  ( 0.05014649552810505201, 217.5146222423826714, 1.251137918078566003 ) ) ;
#22549=CARTESIAN_POINT ( 'NONE',  ( 6.220909254589536808, 215.4770327129947702, 91.55113791807858092 ) ) ;
#22551=CARTESIAN_POINT ( 'NONE',  ( 6.444103211790928043, 211.7408657792734061, 81.69886208192144750 ) ) ;
#22554=CARTESIAN_POINT ( 'NONE',  ( -7.456977232089471386, 217.1783343296987709, 83.94886208192144750 ) ) ;
#22556=CARTESIAN_POINT ( 'NONE',  ( 0.05014649552810506589, 217.5146222423826714, 16.25113791807856600 ) ) ;
#22560=CARTESIAN_POINT ( 'NONE',  ( 9.680171189290831535, 199.9079932115568852, 86.30113791807858092 ) ) ;
#22563=CARTESIAN_POINT ( 'NONE',  ( 7.456977232089471386, 196.8216656703012006, 67.44886208192143329 ) ) ;
#22564=CARTESIAN_POINT ( 'NONE',  ( 6.139770520408223575, 215.5359834540460611, 75.54886208192142760 ) ) ;
#22565=CARTESIAN_POINT ( 'NONE',  ( 3.753561863808876797, 195.6020594897209719, 10.59886208192143542 ) ) ;
#22567=CARTESIAN_POINT ( 'NONE',  ( -10.01549611932653860, 203.7984951890123284, 30.35113791807856742 ) ) ;
#22569=CARTESIAN_POINT ( 'NONE',  ( 6.220909254589681581, 198.5229672870052582, 97.44886208192143329 ) ) ;
#22573=CARTESIAN_POINT ( 'NONE',  ( -8.015496119326597224, 209.5516654185217362, 77.64886208192143613 ) ) ;
#22580=CARTESIAN_POINT ( 'NONE',  ( -8.015496119326531499, 204.4483345814780364, 78.35113791807857808 ) ) ;
#22583=CARTESIAN_POINT ( 'NONE',  ( 4.903702542908435547, 213.8346818373419751, 57.54886208192142760 ) ) ;
#22589=CARTESIAN_POINT ( 'NONE',  ( 3.753561863808689836, 218.3979405102790565, 55.40113791807858235 ) ) ;
#22591=CARTESIAN_POINT ( 'NONE',  ( 9.736236675707914401, 214.0148392665762458, 1.701137918078565736 ) ) ;
#22592=CARTESIAN_POINT ( 'NONE',  ( 6.220909254589536808, 215.4770327129947987, 82.55113791807858092 ) ) ;
#22593=CARTESIAN_POINT ( 'NONE',  ( 3.753561863808876797, 195.6020594897209719, 43.59886208192143897 ) ) ;
#22594=CARTESIAN_POINT ( 'NONE',  ( -6.220909254589682469, 215.4770327129947134, 47.94886208192143329 ) ) ;
#22596=CARTESIAN_POINT ( 'NONE',  ( -3.753561863808691168, 195.6020594897209435, 89.90113791807857524 ) ) ;
#22597=CARTESIAN_POINT ( 'NONE',  ( -9.984503880673473830, 210.2968891136704315, 3.651137918078565026 ) ) ;
#22598=CARTESIAN_POINT ( 'NONE',  ( 10.00000000000000711, 207.0476921513415220, 66.99886208192143044 ) ) ;
#22603=CARTESIAN_POINT ( 'NONE',  ( 3.662846001189864698, 218.4274158808046593, 75.39886208192143613 ) ) ;
#22606=CARTESIAN_POINT ( 'NONE',  ( -8.015496119326597224, 209.5516654185217362, 50.64886208192145034 ) ) ;
#22607=EDGE_CURVE ( 'NONE', #9574, #13603, #11848, .T. ) ;
#22614=CARTESIAN_POINT ( 'NONE',  ( 8.062137200540822946, 212.9164362838583315, 42.69886208192143329 ) ) ;
#22619=CARTESIAN_POINT ( 'NONE',  ( -8.015496119326597224, 209.5516654185217362, 26.64886208192143968 ) ) ;
#22620=CARTESIAN_POINT ( 'NONE',  ( 6.220909254589536808, 215.4770327129947702, 58.55113791807858092 ) ) ;
#22621=CARTESIAN_POINT ( 'NONE',  ( -10.00000000000000711, 207.0476921513413515, 42.50113791807856956 ) ) ;
#22622=CARTESIAN_POINT ( 'NONE',  ( 3.044812012440130555, 197.4746971517856764, 20.60113791807856742 ) ) ;
#22623=CARTESIAN_POINT ( 'NONE',  ( 2.517493886308900919, 214.5937144450984420, 7.401137918078566358 ) ) ;
#22627=CARTESIAN_POINT ( 'NONE',  ( -0.05014649552807705357, 194.3824533091408000, 29.75113791807856956 ) ) ;
#22631=CARTESIAN_POINT ( 'NONE',  ( 0.05014649552810505201, 217.5146222423826714, 79.25113791807856956 ) ) ;
#22632=CARTESIAN_POINT ( 'NONE',  ( 6.220909254589536808, 215.4770327129947987, 46.55113791807856671 ) ) ;
#22636=CARTESIAN_POINT ( 'NONE',  ( -9.680171189290716072, 199.9079932115567146, 14.19886208192143684 ) ) ;
#22637=CARTESIAN_POINT ( 'NONE',  ( -8.062137200540822946, 201.0835637161416400, 17.19886208192143684 ) ) ;
#22640=CARTESIAN_POINT ( 'NONE',  ( -9.680171189290831535, 214.0920067884431148, 57.80113791807857382 ) ) ;
#22641=CARTESIAN_POINT ( 'NONE',  ( -0.05014649552807731031, 198.5883022060938572, 83.75113791807856956 ) ) ;
#22642=CARTESIAN_POINT ( 'NONE',  ( -3.135527875058982783, 216.4958274776886924, 45.09886208192143897 ) ) ;
#22655=CARTESIAN_POINT ( 'NONE',  ( -2.426778023690262742, 214.6231898156240163, 34.10113791807857098 ) ) ;
#22657=CARTESIAN_POINT ( 'NONE',  ( -10.00000000000000711, 206.9523078486584495, 14.49886208192143577 ) ) ;
#22660=CARTESIAN_POINT ( 'NONE',  ( 0.05014649552807626948, 215.4116977939061144, 49.25113791807856956 ) ) ;
#22664=CARTESIAN_POINT ( 'NONE',  ( -3.044812012439970683, 197.4746971517856196, 97.89886208192145034 ) ) ;
#22666=CARTESIAN_POINT ( 'NONE',  ( 8.062137200540920645, 201.0835637161417822, 32.30113791807857382 ) ) ;
#22669=CARTESIAN_POINT ( 'NONE',  ( -10.00000000000000711, 207.0476921513413515, 15.50113791807856600 ) ) ;
#22675=CARTESIAN_POINT ( 'NONE',  ( 7.375838497908181246, 196.7627149292499666, 2.451137918078565736 ) ) ;
#22679=CARTESIAN_POINT ( 'NONE',  ( 0.05014649552810505201, 217.5146222423826714, 46.25113791807855534 ) ) ;
#22686=CARTESIAN_POINT ( 'NONE',  ( 12.00000000000000711, 206.9523078486586485, 32.00113791807856956 ) ) ;
#22688=CARTESIAN_POINT ( 'NONE',  ( 6.139770520408223575, 215.5359834540460611, 3.548862081921434708 ) ) ;
#22692=CARTESIAN_POINT ( 'NONE',  ( 8.118202686958039038, 212.8392687619912635, 61.70113791807857240 ) ) ;
#22695=CARTESIAN_POINT ( 'NONE',  ( -8.015496119326597224, 209.5516654185217362, 20.64886208192143613 ) ) ;
#22699=CARTESIAN_POINT ( 'NONE',  ( -6.500168698208129925, 202.3363017425936050, 0.2011379180785659582 ) ) ;
#22703=CARTESIAN_POINT ( 'NONE',  ( -3.753561863808878130, 218.3979405102790281, 90.09886208192143897 ) ) ;
#22709=CARTESIAN_POINT ( 'NONE',  ( 3.044812012440130555, 197.4746971517856764, 2.601137918078566091 ) ) ;
#22710=CARTESIAN_POINT ( 'NONE',  ( 9.984503880673420539, 210.2968891136705167, 66.84886208192141055 ) ) ;
#22713=CARTESIAN_POINT ( 'NONE',  ( 10.01549611932653860, 210.2015048109876716, 1.851137918078565203 ) ) ;
#22717=CARTESIAN_POINT ( 'NONE',  ( -9.984503880673473830, 210.2968891136704315, 90.65113791807854682 ) ) ;
#22719=CARTESIAN_POINT ( 'NONE',  ( -3.135527875058821579, 197.5041725223112223, 74.90113791807857524 ) ) ;
#22724=CARTESIAN_POINT ( 'NONE',  ( -7.456977232089471386, 217.1783343296987709, 89.94886208192144750 ) ) ;
#22727=CARTESIAN_POINT ( 'NONE',  ( 10.01549611932653860, 210.2015048109876716, 19.85113791807856742 ) ) ;
#22731=CARTESIAN_POINT ( 'NONE',  ( -9.680171189290831535, 214.0920067884431148, 90.80113791807858092 ) ) ;
#22733=AXIS2_PLACEMENT_3D ( 'NONE', #22208, #6023, #919 ) ;
#22735=CARTESIAN_POINT ( 'NONE',  ( -7.375838497908014268, 196.7627149292498530, 74.04886208192142760 ) ) ;
#22736=CARTESIAN_POINT ( 'NONE',  ( -10.00000000000000711, 206.9523078486584495, 89.49886208192144466 ) ) ;
#22737=CARTESIAN_POINT ( 'NONE',  ( -9.736236675708031640, 214.0148392665760753, 11.79886208192143648 ) ) ;
#22739=CARTESIAN_POINT ( 'NONE',  ( 8.118202686958039038, 212.8392687619912635, 31.70113791807856884 ) ) ;
#22741=CARTESIAN_POINT ( 'NONE',  ( 10.01549611932659545, 203.7984951890123853, 100.1488620819214077 ) ) ;
#22743=VERTEX_POINT ( 'NONE', #12981 ) ;
#22745=CARTESIAN_POINT ( 'NONE',  ( -2.426778023690076225, 199.3768101843759553, 76.89886208192143613 ) ) ;
#22755=CARTESIAN_POINT ( 'NONE',  ( 8.000000000000008882, 206.9523078486586485, 83.00113791807856956 ) ) ;
#22760=CARTESIAN_POINT ( 'NONE',  ( -2.426778023690076225, 199.3768101843759553, 49.89886208192144323 ) ) ;
#22766=CARTESIAN_POINT ( 'NONE',  ( 3.662846001190051659, 195.5725841191953691, 56.60113791807857808 ) ) ;
#22769=CARTESIAN_POINT ( 'NONE',  ( -9.680171189290831535, 214.0920067884431148, 3.801137918078565825 ) ) ;
#22770=CARTESIAN_POINT ( 'NONE',  ( 10.01549611932653860, 210.2015048109876716, 73.85113791807857808 ) ) ;
#22772=CARTESIAN_POINT ( 'NONE',  ( -7.375838497908014268, 196.7627149292498530, 47.04886208192144181 ) ) ;
#22773=CARTESIAN_POINT ( 'NONE',  ( -8.118202686958138514, 212.8392687619910930, 47.79886208192143471 ) ) ;
#22775=CARTESIAN_POINT ( 'NONE',  ( -7.456977232089304408, 196.8216656703010301, 87.05113791807856671 ) ) ;
#22777=CARTESIAN_POINT ( 'NONE',  ( -6.139770520408369237, 215.5359834540460042, 6.951137918078566180 ) ) ;
#22778=CARTESIAN_POINT ( 'NONE',  ( 6.139770520408223575, 215.5359834540460611, 72.54886208192144181 ) ) ;
#22782=CARTESIAN_POINT ( 'NONE',  ( -12.00000000000000711, 206.9523078486584780, 74.49886208192144466 ) ) ;
#22785=CARTESIAN_POINT ( 'NONE',  ( 2.517493886309087436, 199.4062855549015865, 49.59886208192143897 ) ) ;
#22789=DIRECTION ( 'NONE',  ( 0.000000000000000000, 0.9988620819214347746, -0.04769215134146093105 ) ) ;
#22793=CARTESIAN_POINT ( 'NONE',  ( -9.984503880673420539, 203.7031108863293980, 38.34886208192143897 ) ) ;
#22799=CARTESIAN_POINT ( 'NONE',  ( -4.984841277089891776, 213.7757310962905990, 20.94886208192143684 ) ) ;
#22800=CARTESIAN_POINT ( 'NONE',  ( -10.00000000000000711, 207.0476921513413515, 75.50113791807858377 ) ) ;
#22803=CARTESIAN_POINT ( 'NONE',  ( 10.01549611932653860, 210.2015048109876716, 46.85113791807856387 ) ) ;
#22804=CARTESIAN_POINT ( 'NONE',  ( -8.062137200540920645, 212.9164362838581894, 15.80113791807856849 ) ) ;
#22805=CARTESIAN_POINT ( 'NONE',  ( 2.426778023690261410, 199.3768101843759837, 2.601137918078566535 ) ) ;
#22808=CARTESIAN_POINT ( 'NONE',  ( 3.662846001190051659, 195.5725841191953691, 26.60113791807856742 ) ) ;
#22810=CARTESIAN_POINT ( 'NONE',  ( 10.01549611932653860, 210.2015048109876716, 73.85113791807857808 ) ) ;
#22811=CARTESIAN_POINT ( 'NONE',  ( -10.00000000000000711, 207.0476921513413515, 48.50113791807856956 ) ) ;
#22814=CARTESIAN_POINT ( 'NONE',  ( 9.736236675708031640, 199.9851607334238963, 13.29886208192143826 ) ) ;
#22815=CARTESIAN_POINT ( 'NONE',  ( 3.044812012439969795, 216.5253028482143520, 21.39886208192143613 ) ) ;
#22818=CARTESIAN_POINT ( 'NONE',  ( 12.00000000000000711, 206.9523078486586485, 56.00113791807856956 ) ) ;
#22820=CARTESIAN_POINT ( 'NONE',  ( -7.984503880673488041, 209.6470497212046098, 81.65113791807856103 ) ) ;
#22821=CARTESIAN_POINT ( 'NONE',  ( 3.135527875058981895, 197.5041725223112792, 40.59886208192143187 ) ) ;
#22829=CARTESIAN_POINT ( 'NONE',  ( 0.05014649552807626948, 215.4116977939061144, 28.25113791807856245 ) ) ;
#22831=CARTESIAN_POINT ( 'NONE',  ( -9.984503880673420539, 203.7031108863293980, 14.34886208192143542 ) ) ;
#22834=CARTESIAN_POINT ( 'NONE',  ( -8.015496119326531499, 204.4483345814780364, 57.35113791807857098 ) ) ;
#22837=CARTESIAN_POINT ( 'NONE',  ( -8.062137200540822946, 201.0835637161416400, 101.1988620819214475 ) ) ;
#22839=CARTESIAN_POINT ( 'NONE',  ( 3.044812012440130555, 197.4746971517856764, 44.60113791807857098 ) ) ;
#22843=CARTESIAN_POINT ( 'NONE',  ( -10.00000000000000711, 207.0476921513413515, 18.50113791807856956 ) ) ;
#22848=CARTESIAN_POINT ( 'NONE',  ( -9.736236675707914401, 199.9851607334237542, 3.201137918078565736 ) ) ;
#22851=CARTESIAN_POINT ( 'NONE',  ( -8.118202686958039038, 201.1607312380087080, 51.20113791807857240 ) ) ;
#22858=CARTESIAN_POINT ( 'NONE',  ( -9.680171189290831535, 214.0920067884431148, 33.80113791807856671 ) ) ;
#22860=CARTESIAN_POINT ( 'NONE',  ( -6.139770520408224463, 198.4640165459539389, 14.04886208192143648 ) ) ;
#22863=CARTESIAN_POINT ( 'NONE',  ( 9.984503880673470277, 203.7031108863295401, 11.15113791807856636 ) ) ;
#22864=CARTESIAN_POINT ( 'NONE',  ( -10.01549611932653860, 203.7984951890123284, 57.35113791807856387 ) ) ;
#22867=CARTESIAN_POINT ( 'NONE',  ( 6.444103211790928043, 211.7408657792734061, 21.69886208192144039 ) ) ;
#22870=CARTESIAN_POINT ( 'NONE',  ( -7.984503880673488041, 209.6470497212046098, 6.651137918078566358 ) ) ;
#22873=CARTESIAN_POINT ( 'NONE',  ( 3.662846001189864698, 218.4274158808046593, 90.39886208192143613 ) ) ;
#22879=CARTESIAN_POINT ( 'NONE',  ( -6.220909254589682469, 215.4770327129946850, 68.94886208192140487 ) ) ;
#22882=CARTESIAN_POINT ( 'NONE',  ( 10.00000000000000711, 206.9523078486586201, 5.001137918078565114 ) ) ;
#22885=CARTESIAN_POINT ( 'NONE',  ( -3.044812012440131443, 216.5253028482142952, 88.10113791807857808 ) ) ;
#22887=CARTESIAN_POINT ( 'NONE',  ( -6.139770520408369237, 215.5359834540460042, 78.95113791807858661 ) ) ;
#22890=CARTESIAN_POINT ( 'NONE',  ( 12.00000000000000711, 207.0476921513415220, 87.99886208192144466 ) ) ;
#22892=CARTESIAN_POINT ( 'NONE',  ( 8.118202686958039038, 212.8392687619912635, 34.70113791807857240 ) ) ;
#22896=CARTESIAN_POINT ( 'NONE',  ( -11.98450388067348804, 210.9467285061362247, 93.65113791807857524 ) ) ;
#22899=CARTESIAN_POINT ( 'NONE',  ( -10.67684754974910888, 206.2195024190491210, 104.1863779807122370 ) ) ;
#22901=CARTESIAN_POINT ( 'NONE',  ( -3.135527875058982783, 216.4958274776886924, 90.09886208192143897 ) ) ;
#22902=CARTESIAN_POINT ( 'NONE',  ( -7.375838497908014268, 196.7627149292498530, 26.04886208192144181 ) ) ;
#22904=CARTESIAN_POINT ( 'NONE',  ( 3.044812012440130555, 197.4746971517856764, 32.60113791807857098 ) ) ;
#22907=CARTESIAN_POINT ( 'NONE',  ( 3.135527875058981895, 197.5041725223112792, 97.59886208192143897 ) ) ;
#22911=CARTESIAN_POINT ( 'NONE',  ( -6.444103211790928043, 202.2591342207265939, 83.19886208192144750 ) ) ;
#22920=CARTESIAN_POINT ( 'NONE',  ( -0.05014649552807731031, 198.5883022060938572, 80.75113791807856956 ) ) ;
#22921=DIRECTION ( 'NONE',  ( -1.000000000000000000, 0.000000000000000000, 0.000000000000000000 ) ) ;
#22924=CARTESIAN_POINT ( 'NONE',  ( -8.000000000000008882, 206.9523078486584780, 50.49886208192144466 ) ) ;
#22925=CARTESIAN_POINT ( 'NONE',  ( 8.062137200540920645, 201.0835637161417822, -0.6988620819214342861 ) ) ;
#22930=CARTESIAN_POINT ( 'NONE',  ( 9.736236675707914401, 214.0148392665762458, 67.70113791807857240 ) ) ;
#22932=CARTESIAN_POINT ( 'NONE',  ( -3.662846001190052991, 218.4274158808045740, 10.10113791807856742 ) ) ;
#22934=CARTESIAN_POINT ( 'NONE',  ( -6.220909254589537696, 198.5229672870051445, 75.05113791807858092 ) ) ;
#22935=CARTESIAN_POINT ( 'NONE',  ( -12.00000000000000711, 206.9523078486584780, 44.49886208192143755 ) ) ;
#22936=CARTESIAN_POINT ( 'NONE',  ( 3.135527875058981895, 197.5041725223112792, 55.59886208192143187 ) ) ;
#22938=CARTESIAN_POINT ( 'NONE',  ( 12.01549611932652972, 210.8513442034534933, 88.85113791807857808 ) ) ;
#22940=CARTESIAN_POINT ( 'NONE',  ( -0.05014649552810635652, 196.4853777576173002, 5.751137918078563338 ) ) ;
#22942=CARTESIAN_POINT ( 'NONE',  ( -3.044812012439970683, 197.4746971517856196, 67.89886208192143613 ) ) ;
#22945=CARTESIAN_POINT ( 'NONE',  ( -12.00000000000000711, 206.9523078486584780, 68.49886208192144466 ) ) ;
#22947=CARTESIAN_POINT ( 'NONE',  ( 8.062137200540920645, 201.0835637161417822, 92.30113791807858092 ) ) ;
#22950=CARTESIAN_POINT ( 'NONE',  ( 8.000000000000008882, 207.0476921513415220, 51.99886208192144466 ) ) ;
#22958=CARTESIAN_POINT ( 'NONE',  ( -9.984503880673420539, 203.7031108863293980, 56.34886208192141765 ) ) ;
#22963=CARTESIAN_POINT ( 'NONE',  ( -8.015496119326597224, 209.5516654185217362, 23.64886208192143968 ) ) ;
#22964=CARTESIAN_POINT ( 'NONE',  ( -6.220909254589537696, 198.5229672870051161, 66.05113791807858092 ) ) ;
#22966=CARTESIAN_POINT ( 'NONE',  ( -10.00000000000000711, 207.0476921513413515, 60.50113791807857666 ) ) ;
#22967=CARTESIAN_POINT ( 'NONE',  ( 6.220909254589536808, 215.4770327129947702, 28.55113791807855961 ) ) ;
#22969=CARTESIAN_POINT ( 'NONE',  ( -4.984841277089726574, 200.2242689037092305, 9.051137918078564937 ) ) ;
#22972=CARTESIAN_POINT ( 'NONE',  ( -11.98450388067348804, 210.9467285061362247, 33.65113791807856813 ) ) ;
#22974=CARTESIAN_POINT ( 'NONE',  ( -6.220909254589537696, 198.5229672870051161, 87.05113791807856671 ) ) ;
#22975=CARTESIAN_POINT ( 'NONE',  ( -6.220909254589537696, 198.5229672870051445, 51.05113791807856671 ) ) ;
#22977=CARTESIAN_POINT ( 'NONE',  ( -7.456977232089471386, 217.1783343296987709, 8.948862081921433287 ) ) ;
#22978=CARTESIAN_POINT ( 'NONE',  ( -6.220909254589682469, 215.4770327129947134, 29.94886208192143329 ) ) ;
#22982=CARTESIAN_POINT ( 'NONE',  ( -9.736236675707914401, 199.9851607334237542, 57.20113791807856529 ) ) ;
#22983=CARTESIAN_POINT ( 'NONE',  ( -0.05014649552807731031, 198.5883022060938572, 77.75113791807856956 ) ) ;
#22985=CARTESIAN_POINT ( 'NONE',  ( 6.139770520408223575, 215.5359834540460611, 39.54886208192143471 ) ) ;
#22988=CARTESIAN_POINT ( 'NONE',  ( -9.680171189290716072, 199.9079932115567146, 41.19886208192144039 ) ) ;
#22996=CARTESIAN_POINT ( 'NONE',  ( 4.903702542908601636, 200.1653181626581102, 32.45113791807857240 ) ) ;
#22998=CARTESIAN_POINT ( 'NONE',  ( -9.984503880673420539, 203.7031108863293980, 17.34886208192143542 ) ) ;
#23001=CARTESIAN_POINT ( 'NONE',  ( 2.517493886308900919, 214.5937144450984420, 61.40113791807856813 ) ) ;
#23005=CARTESIAN_POINT ( 'NONE',  ( 8.062137200540822946, 212.9164362838583315, 99.69886208192144750 ) ) ;
#23008=CARTESIAN_POINT ( 'NONE',  ( 0.05014649552810505201, 217.5146222423826714, 46.25113791807855534 ) ) ;
#23009=CARTESIAN_POINT ( 'NONE',  ( 3.135527875058820690, 216.4958274776887492, 22.40113791807856458 ) ) ;
#23010=CARTESIAN_POINT ( 'NONE',  ( 10.00000000000000711, 207.0476921513415220, 99.99886208192143044 ) ) ;
#23015=CARTESIAN_POINT ( 'NONE',  ( 9.736236675707914401, 214.0148392665762458, 1.701137918078565736 ) ) ;
#23017=CARTESIAN_POINT ( 'NONE',  ( -10.00000000000000711, 207.0476921513413515, 42.50113791807856956 ) ) ;
#23023=EDGE_LOOP ( 'NONE', ( #17577, #15319, #31870, #5298, #17744 ) ) ;
#23024=CARTESIAN_POINT ( 'NONE',  ( 12.00000000000000711, 206.9523078486586485, 26.00113791807856600 ) ) ;
#23026=CARTESIAN_POINT ( 'NONE',  ( 10.00000000000000711, 207.0476921513415220, 9.998862081921435774 ) ) ;
#23030=CARTESIAN_POINT ( 'NONE',  ( -10.01549611932653860, 203.7984951890123284, 9.351137918078569200 ) ) ;
#23031=CARTESIAN_POINT ( 'NONE',  ( -10.00000000000000711, 207.0476921513413515, 66.50113791807856956 ) ) ;
#23033=CARTESIAN_POINT ( 'NONE',  ( -2.426778023690076225, 199.3768101843759553, 19.89886208192143613 ) ) ;
#23037=CARTESIAN_POINT ( 'NONE',  ( 0.05014649552807626948, 215.4116977939061144, 4.251137918078566891 ) ) ;
#23039=CARTESIAN_POINT ( 'NONE',  ( 3.662846001189864698, 218.4274158808046593, 84.39886208192143613 ) ) ;
#23045=CARTESIAN_POINT ( 'NONE',  ( 6.139770520408368348, 198.4640165459539674, 11.45113791807856707 ) ) ;
#23048=CARTESIAN_POINT ( 'NONE',  ( 6.139770520408223575, 215.5359834540460611, 69.54886208192142760 ) ) ;
#23051=CARTESIAN_POINT ( 'NONE',  ( -0.05014649552810635652, 196.4853777576173002, 17.75113791807856245 ) ) ;
#23052=PRODUCT ( 'spring', 'spring', '', ( #13782 ) ) ;
#23056=CARTESIAN_POINT ( 'NONE',  ( -6.220909254589537696, 198.5229672870051161, 102.0511379180785383 ) ) ;
#23058=CARTESIAN_POINT ( 'NONE',  ( 6.220909254589536808, 215.4770327129947702, 76.55113791807855250 ) ) ;
#23061=CARTESIAN_POINT ( 'NONE',  ( 3.753561863808876797, 195.6020594897209719, 85.59886208192143897 ) ) ;
#23066=CARTESIAN_POINT ( 'NONE',  ( -12.01549611932652972, 203.1486557965464499, 99.35113791807857808 ) ) ;
#23070=CARTESIAN_POINT ( 'NONE',  ( -9.984503880673420539, 203.7031108863293980, 83.34886208192142476 ) ) ;
#23071=CARTESIAN_POINT ( 'NONE',  ( 3.753561863808876797, 195.6020594897209719, 22.59886208192143542 ) ) ;
#23073=CARTESIAN_POINT ( 'NONE',  ( 0.05014649552810505201, 217.5146222423826714, 28.25113791807855890 ) ) ;
#23075=CARTESIAN_POINT ( 'NONE',  ( -10.01549611932659722, 210.2015048109875011, 95.64886208192140771 ) ) ;
#23081=CARTESIAN_POINT ( 'NONE',  ( -8.000000000000008882, 206.9523078486584780, 80.49886208192144466 ) ) ;
#23089=CARTESIAN_POINT ( 'NONE',  ( -4.984841277089726574, 200.2242689037092305, 63.05113791807858092 ) ) ;
#23092=CARTESIAN_POINT ( 'NONE',  ( -4.903702542908602524, 213.8346818373418898, 90.95113791807855819 ) ) ;
#23096=CARTESIAN_POINT ( 'NONE',  ( -8.000000000000008882, 206.9523078486584780, 65.49886208192144466 ) ) ;
#23099=CARTESIAN_POINT ( 'NONE',  ( 10.00000000000000711, 206.9523078486586201, -0.9988620819214343305 ) ) ;
#23105=CARTESIAN_POINT ( 'NONE',  ( 12.00000000000000711, 206.9523078486586485, 68.00113791807856956 ) ) ;
#23107=CARTESIAN_POINT ( 'NONE',  ( 9.736236675707914401, 214.0148392665762458, 7.701137918078567068 ) ) ;
#23108=CARTESIAN_POINT ( 'NONE',  ( 8.062137200540920645, 201.0835637161417822, 86.30113791807856671 ) ) ;
#23109=CARTESIAN_POINT ( 'NONE',  ( -3.662846001189865142, 195.5725841191952838, 52.89886208192143613 ) ) ;
#23110=CARTESIAN_POINT ( 'NONE',  ( 8.062137200540822946, 212.9164362838583315, 57.69886208192144039 ) ) ;
#23112=CARTESIAN_POINT ( 'NONE',  ( 12.00000000000000711, 206.9523078486586485, 98.00113791807856956 ) ) ;
#23114=CARTESIAN_POINT ( 'NONE',  ( -8.062137200540920645, 212.9164362838581894, 0.8011379180785658249 ) ) ;
#23115=CARTESIAN_POINT ( 'NONE',  ( -3.044812012439970683, 197.4746971517856196, 70.89886208192143613 ) ) ;
#23118=CARTESIAN_POINT ( 'NONE',  ( -7.375838497908014268, 196.7627149292498530, 77.04886208192142760 ) ) ;
#23119=CARTESIAN_POINT ( 'NONE',  ( -3.135527875058821579, 197.5041725223112223, 89.90113791807857524 ) ) ;
#23122=CARTESIAN_POINT ( 'NONE',  ( -4.903702542908436435, 200.1653181626580249, 50.04886208192144181 ) ) ;
#23131=CARTESIAN_POINT ( 'NONE',  ( 10.00000000000000711, 207.0476921513415220, 48.99886208192143044 ) ) ;
#23136=CARTESIAN_POINT ( 'NONE',  ( 6.444103211790928043, 211.7408657792734061, 33.69886208192144039 ) ) ;
#23138=CARTESIAN_POINT ( 'NONE',  ( 8.118202686958039038, 212.8392687619912635, 67.70113791807858661 ) ) ;
#23141=CARTESIAN_POINT ( 'NONE',  ( -6.139770520408369237, 215.5359834540460042, 54.95113791807856529 ) ) ;
#23142=CARTESIAN_POINT ( 'NONE',  ( 10.00000000000000711, 206.9523078486586201, 26.00113791807856956 ) ) ;
#23143=CARTESIAN_POINT ( 'NONE',  ( -8.015496119326531499, 204.4483345814780364, 9.351137918078563871 ) ) ;
#23147=CARTESIAN_POINT ( 'NONE',  ( -7.456977232089304408, 196.8216656703010301, 39.05113791807855961 ) ) ;
#23149=CARTESIAN_POINT ( 'NONE',  ( -10.00000000000000711, 207.0476921513413515, 87.50113791807858377 ) ) ;
#23150=CARTESIAN_POINT ( 'NONE',  ( -0.05014649552810635652, 196.4853777576173002, 62.75113791807856956 ) ) ;
#23152=CARTESIAN_POINT ( 'NONE',  ( 12.00000000000000711, 207.0476921513415220, 27.99886208192144110 ) ) ;
#23153=CARTESIAN_POINT ( 'NONE',  ( -8.118202686958138514, 212.8392687619910930, 29.79886208192143826 ) ) ;
#23157=CARTESIAN_POINT ( 'NONE',  ( 7.456977232089302632, 217.1783343296989131, 67.55113791807856671 ) ) ;
#23158=CARTESIAN_POINT ( 'NONE',  ( 8.000000000000008882, 206.9523078486586485, 83.00113791807856956 ) ) ;
#23159=CARTESIAN_POINT ( 'NONE',  ( 3.135527875058981895, 197.5041725223112792, 37.59886208192143187 ) ) ;
#23162=CARTESIAN_POINT ( 'NONE',  ( 12.00000000000000711, 207.0476921513415220, 42.99886208192143044 ) ) ;
#23168=CARTESIAN_POINT ( 'NONE',  ( 7.984503880673485376, 204.3529502787953902, 44.15113791807857524 ) ) ;
#23171=CARTESIAN_POINT ( 'NONE',  ( -0.05014649552828403384, 217.5146222423826714, 21.24886208192143400 ) ) ;
#23176=CARTESIAN_POINT ( 'NONE',  ( 2.517493886309087436, 199.4062855549015865, 4.598862081921435419 ) ) ;
#23177=CARTESIAN_POINT ( 'NONE',  ( 10.00000000000000711, 206.9523078486586201, 38.00113791807857666 ) ) ;
#23179=CARTESIAN_POINT ( 'NONE',  ( 3.044812012440130555, 197.4746971517856764, 23.60113791807857098 ) ) ;
#23180=CARTESIAN_POINT ( 'NONE',  ( -9.662634960638639470, 203.2645104739510771, 104.3237470305089403 ) ) ;
#23181=CARTESIAN_POINT ( 'NONE',  ( -0.05014649552828365914, 215.4116977939061144, 81.24886208192143044 ) ) ;
#23185=CARTESIAN_POINT ( 'NONE',  ( -9.736236675707914401, 199.9851607334237542, 12.20113791807856707 ) ) ;
#23188=CARTESIAN_POINT ( 'NONE',  ( 10.01549611932653860, 210.2015048109876716, 58.85113791807856387 ) ) ;
#23195=CARTESIAN_POINT ( 'NONE',  ( 7.456977232089302632, 217.1783343296989131, 40.55113791807856671 ) ) ;
#23197=CARTESIAN_POINT ( 'NONE',  ( -3.135527875058982783, 216.4958274776886924, 9.098862081921435419 ) ) ;
#23200=CARTESIAN_POINT ( 'NONE',  ( -8.062137200540920645, 212.9164362838581894, 6.801137918078565825 ) ) ;
#23201=CARTESIAN_POINT ( 'NONE',  ( 10.01549611932653860, 210.2015048109876716, 70.85113791807854966 ) ) ;
#23204=CARTESIAN_POINT ( 'NONE',  ( -8.015496119326597224, 209.5516654185217362, 35.64886208192143613 ) ) ;
#23208=CARTESIAN_POINT ( 'NONE',  ( -6.500168698208129925, 202.3363017425936050, 12.20113791807856707 ) ) ;
#23210=CARTESIAN_POINT ( 'NONE',  ( -12.01549611932659722, 210.8513442034533227, 95.64886208192143613 ) ) ;
#23214=CARTESIAN_POINT ( 'NONE',  ( -10.00000000000000711, 207.0476921513413515, 9.501137918078566003 ) ) ;
#23215=CARTESIAN_POINT ( 'NONE',  ( -0.05014649552828403384, 217.5146222423826714, 75.24886208192144466 ) ) ;
#23218=CARTESIAN_POINT ( 'NONE',  ( 8.062137200540920645, 201.0835637161417822, 14.30113791807856671 ) ) ;
#23222=CARTESIAN_POINT ( 'NONE',  ( -3.135527875058821579, 197.5041725223112223, 101.9011379180785752 ) ) ;
#23224=CARTESIAN_POINT ( 'NONE',  ( -3.044812012440131443, 216.5253028482142952, 79.10113791807857808 ) ) ;
#23227=CARTESIAN_POINT ( 'NONE',  ( 11.98450388067341876, 210.9467285061363953, 99.84886208192143897 ) ) ;
#23233=CARTESIAN_POINT ( 'NONE',  ( 9.736236675707914401, 214.0148392665762458, 94.70113791807858661 ) ) ;
#23238=CARTESIAN_POINT ( 'NONE',  ( 8.118202686958138514, 201.1607312380088501, 88.29886208192142760 ) ) ;
#23240=CARTESIAN_POINT ( 'NONE',  ( 7.456977232089471386, 196.8216656703012006, 19.44886208192143329 ) ) ;
#23242=CARTESIAN_POINT ( 'NONE',  ( 8.118202686958039038, 212.8392687619912635, 43.70113791807857240 ) ) ;
#23244=CARTESIAN_POINT ( 'NONE',  ( 8.015496119326595448, 204.4483345814782638, 4.148862081921435241 ) ) ;
#23248=CARTESIAN_POINT ( 'NONE',  ( -4.903702542908436435, 200.1653181626580249, 77.04886208192142760 ) ) ;
#23253=CARTESIAN_POINT ( 'NONE',  ( 0.05014649552807626948, 215.4116977939061144, 64.25113791807856956 ) ) ;
#23256=CARTESIAN_POINT ( 'NONE',  ( 6.500168698208129925, 211.6636982574063381, 88.70113791807857240 ) ) ;
#23257=CARTESIAN_POINT ( 'NONE',  ( -0.3755270751584372513, 206.3102596154024297, 117.9458888342408898 ) ) ;
#23262=CARTESIAN_POINT ( 'NONE',  ( -2.426778023690076225, 199.3768101843759553, 64.89886208192143613 ) ) ;
#23266=CARTESIAN_POINT ( 'NONE',  ( 3.135527875058820690, 216.4958274776887492, 1.401137918078565914 ) ) ;
#23270=CARTESIAN_POINT ( 'NONE',  ( -11.98450388067348804, 210.9467285061362247, 69.65113791807856103 ) ) ;
#23272=CARTESIAN_POINT ( 'NONE',  ( -0.05014649552807705357, 194.3824533091408000, 5.751137918078564226 ) ) ;
#23273=CARTESIAN_POINT ( 'NONE',  ( 9.984503880673473830, 203.7031108863295401, 83.15113791807856103 ) ) ;
#23275=CARTESIAN_POINT ( 'NONE',  ( -11.98450388067341876, 203.0532714938636047, 53.34886208192144608 ) ) ;
#23276=CARTESIAN_POINT ( 'NONE',  ( -8.118202686958138514, 212.8392687619910930, 53.79886208192143471 ) ) ;
#23278=CARTESIAN_POINT ( 'NONE',  ( 12.00000000000000711, 206.9523078486586485, 92.00113791807858377 ) ) ;
#23282=CARTESIAN_POINT ( 'NONE',  ( -10.01549611932653860, 203.7984951890123284, 9.351137918078569200 ) ) ;
#23283=CARTESIAN_POINT ( 'NONE',  ( -10.00000000000000711, 206.9523078486584495, 65.49886208192143044 ) ) ;
#23286=CARTESIAN_POINT ( 'NONE',  ( -12.00000000000000711, 206.9523078486584780, 77.49886208192144466 ) ) ;
#23287=CARTESIAN_POINT ( 'NONE',  ( 8.118202686958039038, 212.8392687619912635, 91.70113791807857240 ) ) ;
#23290=CARTESIAN_POINT ( 'NONE',  ( -7.984503880673422316, 204.3529502787951628, 47.34886208192143897 ) ) ;
#23299=CARTESIAN_POINT ( 'NONE',  ( 6.220909254589681581, 198.5229672870052582, 52.44886208192143329 ) ) ;
#23303=CARTESIAN_POINT ( 'NONE',  ( -8.015496119326597224, 209.5516654185217362, 32.64886208192144323 ) ) ;
#23305=CARTESIAN_POINT ( 'NONE',  ( -3.135527875058821579, 197.5041725223112223, 68.90113791807857524 ) ) ;
#23307=CARTESIAN_POINT ( 'NONE',  ( 6.220909254589536808, 215.4770327129947702, 55.55113791807855961 ) ) ;
#23310=CARTESIAN_POINT ( 'NONE',  ( -0.05014649552810635652, 196.4853777576173002, 29.75113791807856956 ) ) ;
#23311=CARTESIAN_POINT ( 'NONE',  ( 8.015496119326531499, 209.5516654185219636, 16.85113791807856742 ) ) ;
#23315=CARTESIAN_POINT ( 'NONE',  ( 11.98450388067348271, 203.0532714938637753, 41.15113791807857524 ) ) ;
#23316=CARTESIAN_POINT ( 'NONE',  ( -5.913191805370921372, 206.1729016772225123, -5.405163435505806468 ) ) ;
#23317=CARTESIAN_POINT ( 'NONE',  ( 10.00000000000000711, 206.9523078486586201, 89.00113791807858377 ) ) ;
#23318=CARTESIAN_POINT ( 'NONE',  ( -6.220909254589537696, 198.5229672870051445, 60.05113791807856671 ) ) ;
#23321=CARTESIAN_POINT ( 'NONE',  ( 3.753561863808876797, 195.6020594897209719, 22.59886208192143542 ) ) ;
#23322=CARTESIAN_POINT ( 'NONE',  ( -8.118202686958138514, 212.8392687619910930, 32.79886208192143471 ) ) ;
#23324=CARTESIAN_POINT ( 'NONE',  ( -3.753561863808691168, 195.6020594897209435, 71.90113791807856103 ) ) ;
#23325=CARTESIAN_POINT ( 'NONE',  ( 2.426778023690261410, 199.3768101843759837, 86.60113791807857808 ) ) ;
#23327=CARTESIAN_POINT ( 'NONE',  ( 10.00000000000000711, 207.0476921513415220, 42.99886208192143044 ) ) ;
#23329=CARTESIAN_POINT ( 'NONE',  ( -9.826550578524280155, 207.8102407865004011, 102.5369383530249223 ) ) ;
#23331=CARTESIAN_POINT ( 'NONE',  ( 7.456977232089471386, 196.8216656703012006, 52.44886208192144039 ) ) ;
#23335=EDGE_CURVE ( 'NONE', #28735, #9574, #9803, .T. ) ;
#23336=TOROIDAL_SURFACE ( 'NONE', #17340, 9.624472924841564136, 1.000000000000000444 ) ;
#23341=CARTESIAN_POINT ( 'NONE',  ( -4.984841277089726574, 200.2242689037092305, 45.05113791807857382 ) ) ;
#23344=CARTESIAN_POINT ( 'NONE',  ( -3.044812012439970683, 197.4746971517856196, 25.89886208192143613 ) ) ;
#23346=AXIS2_PLACEMENT_3D ( 'NONE', #33571, #7685, #26228 ) ;
#23351=CARTESIAN_POINT ( 'NONE',  ( -4.984841277089891776, 213.7757310962905990, 5.948862081921435063 ) ) ;
#23352=CARTESIAN_POINT ( 'NONE',  ( 6.139770520408368348, 198.4640165459539674, 38.45113791807855819 ) ) ;
#23354=CARTESIAN_POINT ( 'NONE',  ( -8.062137200540920645, 212.9164362838581894, 27.80113791807856671 ) ) ;
#23357=CARTESIAN_POINT ( 'NONE',  ( -4.984841277089891776, 213.7757310962905990, 92.94886208192144750 ) ) ;
#23361=CARTESIAN_POINT ( 'NONE',  ( -0.05014649552807705357, 194.3824533091408000, 11.75113791807856600 ) ) ;
#23364=CARTESIAN_POINT ( 'NONE',  ( -3.044812012440131443, 216.5253028482142952, 61.10113791807857098 ) ) ;
#23372=CARTESIAN_POINT ( 'NONE',  ( 0.05014649552807549926, 219.6175466908591716, 40.25113791807856245 ) ) ;
#23374=CARTESIAN_POINT ( 'NONE',  ( 0.05014649552828275708, 196.4853777576173002, 10.74886208192143755 ) ) ;
#23377=CARTESIAN_POINT ( 'NONE',  ( -6.139770520408369237, 215.5359834540460042, 9.951137918078567068 ) ) ;
#23378=CARTESIAN_POINT ( 'NONE',  ( -9.984503880673473830, 210.2968891136704315, 66.65113791807857524 ) ) ;
#23380=CARTESIAN_POINT ( 'NONE',  ( -0.05014649552828365914, 215.4116977939061144, 30.24886208192143755 ) ) ;
#23383=CARTESIAN_POINT ( 'NONE',  ( 4.984841277089725686, 213.7757310962907411, 10.55113791807856671 ) ) ;
#23385=CARTESIAN_POINT ( 'NONE',  ( -9.680171189290716072, 199.9079932115567146, 95.19886208192144750 ) ) ;
#23390=CARTESIAN_POINT ( 'NONE',  ( -3.044812012440131443, 216.5253028482142952, 4.101137918078565647 ) ) ;
#23391=CARTESIAN_POINT ( 'NONE',  ( -10.00000000000000711, 206.9523078486584495, 77.49886208192144466 ) ) ;
#23394=CARTESIAN_POINT ( 'NONE',  ( 0.05014649552810505201, 217.5146222423826714, 10.25113791807856778 ) ) ;
#23398=CARTESIAN_POINT ( 'NONE',  ( -9.949154985843399857, 217.7087784572769067, 102.9933096652613074 ) ) ;
#23400=CARTESIAN_POINT ( 'NONE',  ( -9.984503880673473830, 210.2968891136704315, 87.65113791807854682 ) ) ;
#23403=CARTESIAN_POINT ( 'NONE',  ( 3.753561863808876797, 195.6020594897209719, 97.59886208192145318 ) ) ;
#23408=CARTESIAN_POINT ( 'NONE',  ( 3.662846001190051659, 195.5725841191953691, 95.60113791807857808 ) ) ;
#23411=CARTESIAN_POINT ( 'NONE',  ( -6.220909254589682469, 215.4770327129947134, 86.94886208192141908 ) ) ;
#23412=CARTESIAN_POINT ( 'NONE',  ( -7.375838497908014268, 196.7627149292498530, 23.04886208192143826 ) ) ;
#23414=CARTESIAN_POINT ( 'NONE',  ( -8.062137200540920645, 212.9164362838581894, 39.80113791807857382 ) ) ;
#23416=CARTESIAN_POINT ( 'NONE',  ( 2.517493886309087436, 199.4062855549015865, 7.598862081921434530 ) ) ;
#23419=CARTESIAN_POINT ( 'NONE',  ( 4.984841277089891776, 200.2242689037093726, 91.44886208192143329 ) ) ;
#23422=CARTESIAN_POINT ( 'NONE',  ( 6.444103211791042618, 202.2591342207267644, 35.30113791807856671 ) ) ;
#23429=CARTESIAN_POINT ( 'NONE',  ( -6.444103211791042618, 211.7408657792732356, 84.80113791807858092 ) ) ;
#23432=CARTESIAN_POINT ( 'NONE',  ( -4.984841277089891776, 213.7757310962905990, 65.94886208192144750 ) ) ;
#23435=CARTESIAN_POINT ( 'NONE',  ( 3.135527875058820690, 216.4958274776887492, 4.401137918078565470 ) ) ;
#23439=CARTESIAN_POINT ( 'NONE',  ( -9.736236675707914401, 199.9851607334237542, 63.20113791807857240 ) ) ;
#23441=CARTESIAN_POINT ( 'NONE',  ( -3.753561863808691168, 195.6020594897209435, 14.90113791807856636 ) ) ;
#23442=CARTESIAN_POINT ( 'NONE',  ( 8.062137200540920645, 201.0835637161417822, 83.30113791807858092 ) ) ;
#23444=CARTESIAN_POINT ( 'NONE',  ( -12.01549611932659722, 210.8513442034533227, 56.64886208192142902 ) ) ;
#23445=CARTESIAN_POINT ( 'NONE',  ( 10.01549611932659367, 203.7984951890124421, 61.14886208192144323 ) ) ;
#23446=CARTESIAN_POINT ( 'NONE',  ( 12.00000000000000711, 206.9523078486586485, 101.0011379180785696 ) ) ;
#23448=CARTESIAN_POINT ( 'NONE',  ( 10.01549611932653860, 210.2015048109876716, 10.85113791807856387 ) ) ;
#23449=CARTESIAN_POINT ( 'NONE',  ( -10.01549611932659722, 210.2015048109875011, 77.64886208192143613 ) ) ;
#23451=CARTESIAN_POINT ( 'NONE',  ( -12.00000000000000711, 206.9523078486584780, 80.49886208192144466 ) ) ;
#23452=CARTESIAN_POINT ( 'NONE',  ( 3.135527875058820690, 216.4958274776887492, 100.4011379180785752 ) ) ;
#23455=CARTESIAN_POINT ( 'NONE',  ( -4.903702542908436435, 200.1653181626580249, 65.04886208192144181 ) ) ;
#23464=CARTESIAN_POINT ( 'NONE',  ( -10.01549611932659722, 210.2015048109875011, 50.64886208192143613 ) ) ;
#23469=CARTESIAN_POINT ( 'NONE',  ( 7.984503880673422316, 209.6470497212048372, 33.84886208192144608 ) ) ;
#23470=CARTESIAN_POINT ( 'NONE',  ( 0.05014649552810505201, 217.5146222423826714, 70.25113791807858377 ) ) ;
#23472=CARTESIAN_POINT ( 'NONE',  ( -0.05014649552810635652, 196.4853777576173002, 56.75113791807855534 ) ) ;
#23473=CARTESIAN_POINT ( 'NONE',  ( 8.062137200540920645, 201.0835637161417822, 23.30113791807856671 ) ) ;
#23474=CARTESIAN_POINT ( 'NONE',  ( -6.500168698208129925, 202.3363017425936050, 18.20113791807856529 ) ) ;
#23478=CARTESIAN_POINT ( 'NONE',  ( 11.98450388067348271, 203.0532714938637753, 38.15113791807856813 ) ) ;
#23481=CARTESIAN_POINT ( 'NONE',  ( -10.01549611932653860, 203.7984951890123284, 81.35113791807857808 ) ) ;
#23482=CARTESIAN_POINT ( 'NONE',  ( 10.01549611932653860, 210.2015048109876716, 55.85113791807857098 ) ) ;
#23483=CARTESIAN_POINT ( 'NONE',  ( 0.05014649552828288198, 194.3824533091408000, 19.74886208192143400 ) ) ;
#23484=CARTESIAN_POINT ( 'NONE',  ( 10.00000000000000711, 207.0476921513415220, 27.99886208192143755 ) ) ;
#23487=CARTESIAN_POINT ( 'NONE',  ( 9.736236675707914401, 214.0148392665762458, 64.70113791807857240 ) ) ;
#23488=CARTESIAN_POINT ( 'NONE',  ( 8.000000000000008882, 206.9523078486586485, 89.00113791807858377 ) ) ;
#23490=CARTESIAN_POINT ( 'NONE',  ( -9.984503880673420539, 203.7031108863293980, 50.34886208192141765 ) ) ;
#23493=CARTESIAN_POINT ( 'NONE',  ( 12.01549611932659367, 203.1486557965466773, 49.14886208192143613 ) ) ;
#23500=CARTESIAN_POINT ( 'NONE',  ( 4.984841277089725686, 213.7757310962907411, 46.55113791807856671 ) ) ;
#23502=CARTESIAN_POINT ( 'NONE',  ( 6.139770520408223575, 215.5359834540460611, 24.54886208192143471 ) ) ;
#23508=CARTESIAN_POINT ( 'NONE',  ( -4.984841277089891776, 213.7757310962905990, 8.948862081921433287 ) ) ;
#23509=CARTESIAN_POINT ( 'NONE',  ( 8.118202686958039038, 212.8392687619912635, 43.70113791807857240 ) ) ;
#23512=CARTESIAN_POINT ( 'NONE',  ( 9.984503880673470277, 203.7031108863295401, 29.15113791807856103 ) ) ;
#23513=CARTESIAN_POINT ( 'NONE',  ( -10.01549611932659545, 210.2015048109875011, 101.6488620819214361 ) ) ;
#23515=CARTESIAN_POINT ( 'NONE',  ( 8.000000000000008882, 207.0476921513415220, 87.99886208192144466 ) ) ;
#23520=CARTESIAN_POINT ( 'NONE',  ( -12.01549611932652972, 203.1486557965464499, 6.351137918078565647 ) ) ;
#23524=CARTESIAN_POINT ( 'NONE',  ( 8.118202686958039038, 212.8392687619912635, 55.70113791807857950 ) ) ;
#23525=CARTESIAN_POINT ( 'NONE',  ( -8.118202686958039038, 201.1607312380087080, 30.20113791807856884 ) ) ;
#23527=CARTESIAN_POINT ( 'NONE',  ( -10.00000000000000178, 206.9999999999998863, 103.5000000000000426 ) ) ;
#23528=CARTESIAN_POINT ( 'NONE',  ( 6.220909254589680693, 198.5229672870052582, 1.448862081921434397 ) ) ;
#23531=CARTESIAN_POINT ( 'NONE',  ( -9.680171189290831535, 214.0920067884431148, 36.80113791807856671 ) ) ;
#23534=CARTESIAN_POINT ( 'NONE',  ( 6.220909254589681581, 198.5229672870052582, 10.44886208192143506 ) ) ;
#23538=CARTESIAN_POINT ( 'NONE',  ( -8.118202686958039038, 201.1607312380087080, 75.20113791807857240 ) ) ;
#23540=CARTESIAN_POINT ( 'NONE',  ( 8.015496119326595448, 204.4483345814782638, 28.14886208192143968 ) ) ;
#23542=ORIENTED_EDGE ( 'NONE', *, *, #18364, .T. ) ;
#23543=CARTESIAN_POINT ( 'NONE',  ( -2.517493886308901807, 199.4062855549015012, 8.901137918078566358 ) ) ;
#23545=CARTESIAN_POINT ( 'NONE',  ( 12.01549611932659367, 203.1486557965466773, 103.1488620819214361 ) ) ;
#23550=CARTESIAN_POINT ( 'NONE',  ( -10.00000000000000711, 207.0476921513413515, 12.50113791807856778 ) ) ;
#23551=CARTESIAN_POINT ( 'NONE',  ( -8.062137200540822946, 201.0835637161416400, 80.19886208192143329 ) ) ;
#23554=CARTESIAN_POINT ( 'NONE',  ( 10.00000000000000711, 206.9523078486586201, 17.00113791807856600 ) ) ;
#23562=CARTESIAN_POINT ( 'NONE',  ( 8.118202686958039038, 212.8392687619912635, 88.70113791807857240 ) ) ;
#23567=CARTESIAN_POINT ( 'NONE',  ( -12.00000000000000711, 206.9523078486584780, 101.4988620819214304 ) ) ;
#23573=CARTESIAN_POINT ( 'NONE',  ( 11.98450388067348271, 203.0532714938637753, 92.15113791807856103 ) ) ;
#23578=CARTESIAN_POINT ( 'NONE',  ( 8.118202686958138514, 201.1607312380088501, 91.29886208192144181 ) ) ;
#23579=CARTESIAN_POINT ( 'NONE',  ( 0.05014649552828288198, 194.3824533091408000, 25.74886208192143755 ) ) ;
#23581=CARTESIAN_POINT ( 'NONE',  ( 10.01549611932653860, 210.2015048109876716, 46.85113791807856387 ) ) ;
#23583=CARTESIAN_POINT ( 'NONE',  ( -8.000000000000008882, 206.9523078486584780, 8.498862081921435774 ) ) ;
#23588=CARTESIAN_POINT ( 'NONE',  ( -0.05014649552828365914, 215.4116977939061144, 93.24886208192143044 ) ) ;
#23589=CARTESIAN_POINT ( 'NONE',  ( -2.426778023690262742, 214.6231898156240163, 31.10113791807856742 ) ) ;
#23597=CARTESIAN_POINT ( 'NONE',  ( 7.984503880673485376, 204.3529502787953902, 92.15113791807856103 ) ) ;
#23601=CARTESIAN_POINT ( 'NONE',  ( -6.500168698208244500, 211.6636982574061676, 59.79886208192143471 ) ) ;
#23604=CARTESIAN_POINT ( 'NONE',  ( -6.220909254589537696, 198.5229672870051445, 6.051137918078565825 ) ) ;
#23608=CARTESIAN_POINT ( 'NONE',  ( 7.456977232089302632, 217.1783343296989131, 70.55113791807856671 ) ) ;
#23610=CARTESIAN_POINT ( 'NONE',  ( -10.00000000000000711, 207.0476921513413515, 87.50113791807858377 ) ) ;
#23611=CARTESIAN_POINT ( 'NONE',  ( -12.01549611932659722, 210.8513442034533227, 53.64886208192142902 ) ) ;
#23612=CARTESIAN_POINT ( 'NONE',  ( -6.139770520408224463, 198.4640165459539105, 59.04886208192143471 ) ) ;
#23614=CARTESIAN_POINT ( 'NONE',  ( -7.456977232089304408, 196.8216656703010301, 96.05113791807858092 ) ) ;
#23616=CARTESIAN_POINT ( 'NONE',  ( -8.118202686958039038, 201.1607312380087080, 12.20113791807856707 ) ) ;
#23618=CARTESIAN_POINT ( 'NONE',  ( -8.062137200540822946, 201.0835637161416400, 80.19886208192143329 ) ) ;
#23620=CARTESIAN_POINT ( 'NONE',  ( -10.01549611932653860, 203.7984951890123284, 96.35113791807853545 ) ) ;
#23623=CARTESIAN_POINT ( 'NONE',  ( 4.903702542908435547, 213.8346818373419751, 63.54886208192144181 ) ) ;
#23630=CARTESIAN_POINT ( 'NONE',  ( 7.984503880673485376, 204.3529502787953902, 62.15113791807858945 ) ) ;
#23632=CARTESIAN_POINT ( 'NONE',  ( 3.135527875058981895, 197.5041725223112792, 49.59886208192143897 ) ) ;
#23637=CARTESIAN_POINT ( 'NONE',  ( -2.517493886309087880, 214.5937144450984135, 33.09886208192143897 ) ) ;
#23638=CARTESIAN_POINT ( 'NONE',  ( -8.062137200540920645, 212.9164362838581894, 78.80113791807858092 ) ) ;
#23640=CARTESIAN_POINT ( 'NONE',  ( -10.01549611932653860, 203.7984951890123284, 54.35113791807856387 ) ) ;
#23641=CARTESIAN_POINT ( 'NONE',  ( 0.05014649552810505201, 217.5146222423826714, 28.25113791807855890 ) ) ;
#23642=CARTESIAN_POINT ( 'NONE',  ( 2.517493886308900919, 214.5937144450984420, 13.40113791807856636 ) ) ;
#23646=CARTESIAN_POINT ( 'NONE',  ( -12.00000000000000711, 207.0476921513413515, 42.50113791807856245 ) ) ;
#23648=CARTESIAN_POINT ( 'NONE',  ( 9.984503880673470277, 203.7031108863295401, 89.15113791807857524 ) ) ;
#23650=CARTESIAN_POINT ( 'NONE',  ( -0.05014649552810635652, 196.4853777576173002, 59.75113791807857666 ) ) ;
#23651=CARTESIAN_POINT ( 'NONE',  ( 12.00000000000000711, 207.0476921513415220, 18.99886208192143400 ) ) ;
#23652=CARTESIAN_POINT ( 'NONE',  ( 3.135527875058981895, 197.5041725223112792, 25.59886208192143897 ) ) ;
#23654=CARTESIAN_POINT ( 'NONE',  ( 12.01549611932652972, 210.8513442034534933, 70.85113791807857808 ) ) ;
#23655=CARTESIAN_POINT ( 'NONE',  ( -6.500168698208129925, 202.3363017425936050, 84.20113791807858661 ) ) ;
#23656=CARTESIAN_POINT ( 'NONE',  ( -10.01549611932659722, 210.2015048109875011, 53.64886208192141481 ) ) ;
#23659=CARTESIAN_POINT ( 'NONE',  ( -12.01549611932659722, 210.8513442034533227, 50.64886208192143613 ) ) ;
#23664=CARTESIAN_POINT ( 'NONE',  ( 7.984503880673485376, 204.3529502787953902, 41.15113791807857524 ) ) ;
#23666=CARTESIAN_POINT ( 'NONE',  ( -9.984503880673420539, 203.7031108863293980, 26.34886208192142831 ) ) ;
#23672=CARTESIAN_POINT ( 'NONE',  ( -7.984503880673422316, 204.3529502787951628, 5.348862081921435419 ) ) ;
#23674=CARTESIAN_POINT ( 'NONE',  ( -10.01549611932653860, 203.7984951890123284, 54.35113791807856387 ) ) ;
#23677=CARTESIAN_POINT ( 'NONE',  ( 3.135527875058820690, 216.4958274776887492, 28.40113791807856813 ) ) ;
#23679=CARTESIAN_POINT ( 'NONE',  ( 4.984841277089891776, 200.2242689037093726, 91.44886208192143329 ) ) ;
#23683=CARTESIAN_POINT ( 'NONE',  ( -12.00000000000000711, 207.0476921513413515, 9.501137918078566003 ) ) ;
#23686=CARTESIAN_POINT ( 'NONE',  ( 9.984503880673470277, 203.7031108863295401, 59.15113791807858235 ) ) ;
#23688=CARTESIAN_POINT ( 'NONE',  ( 6.139770520408367460, 198.4640165459539389, 32.45113791807857240 ) ) ;
#23691=CARTESIAN_POINT ( 'NONE',  ( 8.062137200540822946, 212.9164362838583315, 3.698862081921434619 ) ) ;
#23694=CARTESIAN_POINT ( 'NONE',  ( 12.01549611932652972, 210.8513442034534933, 40.85113791807856387 ) ) ;
#23695=DIRECTION ( 'NONE',  ( -0.8289387912553660698, 0.000000000000000000, 0.5593393248754217062 ) ) ;
#23696=CARTESIAN_POINT ( 'NONE',  ( -3.135527875058982783, 216.4958274776886924, 24.09886208192143542 ) ) ;
#23700=CARTESIAN_POINT ( 'NONE',  ( 10.01549611932653860, 210.2015048109876716, 67.85113791807857808 ) ) ;
#23706=CARTESIAN_POINT ( 'NONE',  ( -7.984503880673488041, 209.6470497212046098, 15.65113791807856636 ) ) ;
#23708=CARTESIAN_POINT ( 'NONE',  ( 3.753561863808876797, 195.6020594897209719, 97.59886208192145318 ) ) ;
#23713=CARTESIAN_POINT ( 'NONE',  ( 6.139770520408368348, 198.4640165459539674, 8.451137918078565292 ) ) ;
#23714=CARTESIAN_POINT ( 'NONE',  ( 0.05014649552828275708, 196.4853777576173002, 79.74886208192143044 ) ) ;
#23718=CARTESIAN_POINT ( 'NONE',  ( -3.044812012440131443, 216.5253028482142952, 10.10113791807856565 ) ) ;
#23721=CARTESIAN_POINT ( 'NONE',  ( 3.135527875058820690, 216.4958274776887492, 97.40113791807858945 ) ) ;
#23723=CARTESIAN_POINT ( 'NONE',  ( -9.984503880673473830, 210.2968891136704315, 84.65113791807857524 ) ) ;
#23726=CARTESIAN_POINT ( 'NONE',  ( -9.680171189290716072, 199.9079932115567146, 92.19886208192143329 ) ) ;
#23734=CARTESIAN_POINT ( 'NONE',  ( -0.05014649552828402690, 217.5146222423826714, 96.24886208192144466 ) ) ;
#23735=CARTESIAN_POINT ( 'NONE',  ( -9.680171189290716072, 199.9079932115567146, 32.19886208192144039 ) ) ;
#23737=CARTESIAN_POINT ( 'NONE',  ( -3.135527875058821579, 197.5041725223112223, 41.90113791807856813 ) ) ;
#23739=CARTESIAN_POINT ( 'NONE',  ( -8.000000000000008882, 206.9523078486584780, 5.498862081921434886 ) ) ;
#23745=CARTESIAN_POINT ( 'NONE',  ( 2.517493886309087436, 199.4062855549015865, 94.59886208192145318 ) ) ;
#23747=CARTESIAN_POINT ( 'NONE',  ( -0.05014649552807731031, 198.5883022060938572, 26.75113791807856956 ) ) ;
#23755=CARTESIAN_POINT ( 'NONE',  ( -7.984503880673488041, 209.6470497212046098, 87.65113791807857524 ) ) ;
#23758=CARTESIAN_POINT ( 'NONE',  ( -4.903702542908436435, 200.1653181626580249, 77.04886208192142760 ) ) ;
#23762=CARTESIAN_POINT ( 'NONE',  ( -10.00000000000000711, 207.0476921513413515, 15.50113791807856600 ) ) ;
#23767=CARTESIAN_POINT ( 'NONE',  ( 11.98450388067348271, 203.0532714938637753, 77.15113791807857524 ) ) ;
#23769=CARTESIAN_POINT ( 'NONE',  ( 8.118202686958039038, 212.8392687619912635, 91.70113791807857240 ) ) ;
#23773=CARTESIAN_POINT ( 'NONE',  ( -0.05014649552828442242, 219.6175466908591716, 54.24886208192143755 ) ) ;
#23774=CARTESIAN_POINT ( 'NONE',  ( -8.062137200540822946, 201.0835637161416400, 71.19886208192144750 ) ) ;
#23775=CARTESIAN_POINT ( 'NONE',  ( -12.00000000000000711, 206.9523078486584780, 5.498862081921433997 ) ) ;
#23777=CARTESIAN_POINT ( 'NONE',  ( -3.044812012440131443, 216.5253028482142952, 13.10113791807856742 ) ) ;
#23778=CARTESIAN_POINT ( 'NONE',  ( 6.139770520408223575, 215.5359834540460611, 81.54886208192144181 ) ) ;
#23780=CARTESIAN_POINT ( 'NONE',  ( 10.01549611932653860, 210.2015048109876716, 97.85113791807857808 ) ) ;
#23781=ORIENTED_EDGE ( 'NONE', *, *, #21478, .F. ) ;
#23783=CARTESIAN_POINT ( 'NONE',  ( -8.015496119326597224, 209.5516654185217362, 65.64886208192142192 ) ) ;
#23785=ORIENTED_EDGE ( 'NONE', *, *, #14125, .F. ) ;
#23792=CARTESIAN_POINT ( 'NONE',  ( 4.984841277089725686, 213.7757310962907411, 58.55113791807858092 ) ) ;
#23794=CARTESIAN_POINT ( 'NONE',  ( -9.000000000000005329, 206.8877928634024101, 103.6076739047741029 ) ) ;
#23796=CARTESIAN_POINT ( 'NONE',  ( -2.426778023690076225, 199.3768101843759553, 34.89886208192144323 ) ) ;
#23797=CARTESIAN_POINT ( 'NONE',  ( 8.062137200540920645, 201.0835637161417822, 83.30113791807858092 ) ) ;
#23799=CARTESIAN_POINT ( 'NONE',  ( -0.05014649552810635652, 196.4853777576173002, 68.75113791807855534 ) ) ;
#23801=CARTESIAN_POINT ( 'NONE',  ( -6.444103211791042618, 211.7408657792732356, 18.80113791807856671 ) ) ;
#23805=CARTESIAN_POINT ( 'NONE',  ( 7.456977232089302632, 217.1783343296989131, 37.55113791807855961 ) ) ;
#23807=CARTESIAN_POINT ( 'NONE',  ( -8.062137200540920645, 212.9164362838581894, 96.80113791807858092 ) ) ;
#23808=CARTESIAN_POINT ( 'NONE',  ( 6.139770520408367460, 198.4640165459539389, 59.45113791807856529 ) ) ;
#23810=CARTESIAN_POINT ( 'NONE',  ( -11.98450388067341876, 203.0532714938636047, 26.34886208192143897 ) ) ;
#23811=CARTESIAN_POINT ( 'NONE',  ( -6.220909254589682469, 215.4770327129947134, 41.94886208192144039 ) ) ;
#23814=CARTESIAN_POINT ( 'NONE',  ( -7.375838497908182134, 217.2372850707499765, 63.95113791807857240 ) ) ;
#23815=CARTESIAN_POINT ( 'NONE',  ( 2.426778023690261410, 199.3768101843759837, 89.60113791807857808 ) ) ;
#23816=CARTESIAN_POINT ( 'NONE',  ( -6.139770520408224463, 198.4640165459539389, 47.04886208192142050 ) ) ;
#23820=CARTESIAN_POINT ( 'NONE',  ( -11.98450388067341876, 203.0532714938636047, 50.34886208192144608 ) ) ;
#23826=CARTESIAN_POINT ( 'NONE',  ( 2.517493886308900919, 214.5937144450984420, 43.40113791807856813 ) ) ;
#23830=CARTESIAN_POINT ( 'NONE',  ( 6.139770520408223575, 215.5359834540460611, 27.54886208192142760 ) ) ;
#23835=CARTESIAN_POINT ( 'NONE',  ( 6.444103211790928043, 211.7408657792734061, 3.698862081921435063 ) ) ;
#23836=CARTESIAN_POINT ( 'NONE',  ( 8.062137200540920645, 201.0835637161417822, 53.30113791807857382 ) ) ;
#23838=CARTESIAN_POINT ( 'NONE',  ( 10.01549611932653860, 210.2015048109876716, 25.85113791807856742 ) ) ;
#23842=CARTESIAN_POINT ( 'NONE',  ( -4.903702542908436435, 200.1653181626580249, 95.04886208192144181 ) ) ;
#23845=CARTESIAN_POINT ( 'NONE',  ( 7.375838497908181246, 196.7627149292499666, 8.451137918078563516 ) ) ;
#23848=CARTESIAN_POINT ( 'NONE',  ( -10.01549611932653860, 203.7984951890123284, 60.35113791807857808 ) ) ;
#23849=CARTESIAN_POINT ( 'NONE',  ( -6.220909254589537696, 198.5229672870051445, 27.05113791807856671 ) ) ;
#23855=CARTESIAN_POINT ( 'NONE',  ( 7.375838497908181246, 196.7627149292499666, 35.45113791807855819 ) ) ;
#23858=CARTESIAN_POINT ( 'NONE',  ( 3.135527875058981895, 197.5041725223112792, 25.59886208192143897 ) ) ;
#23863=CARTESIAN_POINT ( 'NONE',  ( -3.135527875058821579, 197.5041725223112223, 80.90113791807858945 ) ) ;
#23869=CARTESIAN_POINT ( 'NONE',  ( 7.984503880673485376, 204.3529502787953902, 14.15113791807856991 ) ) ;
#23872=CARTESIAN_POINT ( 'NONE',  ( 0.05014649552828288198, 194.3824533091408000, 97.74886208192141623 ) ) ;
#23879=CARTESIAN_POINT ( 'NONE',  ( -9.984503880673420539, 203.7031108863293980, 83.34886208192139634 ) ) ;
#23881=CARTESIAN_POINT ( 'NONE',  ( 8.118202686958039038, 212.8392687619912635, 22.70113791807856884 ) ) ;
#23889=CARTESIAN_POINT ( 'NONE',  ( 6.139770520408368348, 198.4640165459539674, 80.45113791807857240 ) ) ;
#23892=CARTESIAN_POINT ( 'NONE',  ( -12.01549611932659722, 210.8513442034533227, 98.64886208192146455 ) ) ;
#23903=CARTESIAN_POINT ( 'NONE',  ( 0.05014649552828275014, 196.4853777576173002, 91.74886208192144466 ) ) ;
#23904=CARTESIAN_POINT ( 'NONE',  ( -7.456977232089471386, 217.1783343296987709, 32.94886208192144039 ) ) ;
#23907=CARTESIAN_POINT ( 'NONE',  ( 6.139770520408368348, 198.4640165459539674, 56.45113791807857950 ) ) ;
#23910=CARTESIAN_POINT ( 'NONE',  ( -8.015496119326597224, 209.5516654185217362, 2.648862081921435241 ) ) ;
#23913=CARTESIAN_POINT ( 'NONE',  ( -6.444103211790928043, 202.2591342207265939, 95.19886208192144750 ) ) ;
#23914=CARTESIAN_POINT ( 'NONE',  ( 6.444103211791042618, 202.2591342207267644, 32.30113791807856671 ) ) ;
#23920=CARTESIAN_POINT ( 'NONE',  ( 2.426778023690261410, 199.3768101843759837, 101.6011379180785781 ) ) ;
#23923=CARTESIAN_POINT ( 'NONE',  ( 6.500168698208244500, 202.3363017425938324, 70.29886208192142760 ) ) ;
#23924=TOROIDAL_SURFACE ( 'NONE', #19576, 4.999999999999993783, 1.000000000000000222 ) ;
#23929=CARTESIAN_POINT ( 'NONE',  ( 0.05014649552810506589, 217.5146222423826714, 10.25113791807856600 ) ) ;
#23934=CARTESIAN_POINT ( 'NONE',  ( -12.01549611932652972, 203.1486557965464499, 75.35113791807856387 ) ) ;
#23937=CARTESIAN_POINT ( 'NONE',  ( -3.044812012440131443, 216.5253028482142952, 97.10113791807857808 ) ) ;
#23940=CARTESIAN_POINT ( 'NONE',  ( -3.753561863808878130, 218.3979405102790281, 63.09886208192143187 ) ) ;
#23941=CARTESIAN_POINT ( 'NONE',  ( -9.984503880673420539, 203.7031108863293980, 65.34886208192143897 ) ) ;
#23942=CARTESIAN_POINT ( 'NONE',  ( -11.98450388067341876, 203.0532714938636047, 8.348862081921435419 ) ) ;
#23944=CARTESIAN_POINT ( 'NONE',  ( -6.220909254589537696, 198.5229672870051161, 9.051137918078561384 ) ) ;
#23946=CARTESIAN_POINT ( 'NONE',  ( -10.00000000000000711, 206.9523078486584495, 80.49886208192143044 ) ) ;
#23948=CARTESIAN_POINT ( 'NONE',  ( -3.135527875058821579, 197.5041725223112223, 95.90113791807858945 ) ) ;
#23951=CARTESIAN_POINT ( 'NONE',  ( -4.903702542908436435, 200.1653181626580249, 59.04886208192144181 ) ) ;
#23955=CARTESIAN_POINT ( 'NONE',  ( -0.3755270751584372513, 206.7692714347155629, 108.3323677711371573 ) ) ;
#23959=CARTESIAN_POINT ( 'NONE',  ( -7.984503880673488041, 209.6470497212046098, 60.65113791807856813 ) ) ;
#23960=( LENGTH_UNIT ( ) NAMED_UNIT ( * ) SI_UNIT ( .MILLI., .METRE. ) );
#23964=CARTESIAN_POINT ( 'NONE',  ( 6.444103211790928043, 211.7408657792734061, 45.69886208192144750 ) ) ;
#23965=CARTESIAN_POINT ( 'NONE',  ( 8.118202686958039038, 212.8392687619912635, 76.70113791807857240 ) ) ;
#23966=CARTESIAN_POINT ( 'NONE',  ( 10.00000000000000711, 206.9523078486586201, 62.00113791807856956 ) ) ;
#23969=CARTESIAN_POINT ( 'NONE',  ( -7.984503880673488041, 209.6470497212046098, 15.65113791807856636 ) ) ;
#23973=CARTESIAN_POINT ( 'NONE',  ( -12.01549611932652972, 203.1486557965464499, 45.35113791807857098 ) ) ;
#23976=CARTESIAN_POINT ( 'NONE',  ( -3.044812012440131443, 216.5253028482142952, 91.10113791807857808 ) ) ;
#23978=CARTESIAN_POINT ( 'NONE',  ( -8.062137200540920645, 212.9164362838581894, 66.80113791807858092 ) ) ;
#23979=CARTESIAN_POINT ( 'NONE',  ( 3.662846001189864698, 218.4274158808046593, 33.39886208192143613 ) ) ;
#23980=CARTESIAN_POINT ( 'NONE',  ( 3.044812012439969795, 216.5253028482143520, 36.39886208192142902 ) ) ;
#23983=CARTESIAN_POINT ( 'NONE',  ( -7.375838497908182134, 217.2372850707499765, 78.95113791807858661 ) ) ;
#23984=CARTESIAN_POINT ( 'NONE',  ( 6.444103211791042618, 202.2591342207267644, 86.30113791807858092 ) ) ;
#23985=CARTESIAN_POINT ( 'NONE',  ( 3.044812012439969795, 216.5253028482143520, 51.39886208192143613 ) ) ;
#23988=CARTESIAN_POINT ( 'NONE',  ( 9.736236675708031640, 199.9851607334238963, 52.29886208192143471 ) ) ;
#23989=ORIENTED_EDGE ( 'NONE', *, *, #13443, .F. ) ;
#23994=CARTESIAN_POINT ( 'NONE',  ( 4.903702542908601636, 200.1653181626581102, 53.45113791807857950 ) ) ;
#23997=CARTESIAN_POINT ( 'NONE',  ( 8.118202686958138514, 201.1607312380088501, 34.29886208192143471 ) ) ;
#24002=CARTESIAN_POINT ( 'NONE',  ( 8.000000000000008882, 207.0476921513415220, 12.99886208192143400 ) ) ;
#24003=CARTESIAN_POINT ( 'NONE',  ( -8.118202686958039038, 201.1607312380087080, 48.20113791807857950 ) ) ;
#24005=CARTESIAN_POINT ( 'NONE',  ( 3.135527875058820690, 216.4958274776887492, 40.40113791807857524 ) ) ;
#24008=AXIS2_PLACEMENT_3D ( 'NONE', #4624, #25063, #4276 ) ;
#24009=CARTESIAN_POINT ( 'NONE',  ( -4.984841277089891776, 213.7757310962905990, 95.94886208192144750 ) ) ;
#24013=CARTESIAN_POINT ( 'NONE',  ( -0.05014649552807705357, 194.3824533091408000, 17.75113791807856956 ) ) ;
#24016=CARTESIAN_POINT ( 'NONE',  ( -0.05014649552810635652, 196.4853777576173002, 62.75113791807856956 ) ) ;
#24017=CARTESIAN_POINT ( 'NONE',  ( 10.01549611932653860, 210.2015048109876716, 40.85113791807857098 ) ) ;
#24021=CARTESIAN_POINT ( 'NONE',  ( -9.984503880673420539, 203.7031108863293980, 5.348862081921434530 ) ) ;
#24024=CARTESIAN_POINT ( 'NONE',  ( 11.98450388067348271, 203.0532714938637753, 53.15113791807857524 ) ) ;
#24026=CARTESIAN_POINT ( 'NONE',  ( 10.01549611932659545, 203.7984951890123853, 22.14886208192143613 ) ) ;
#24028=CARTESIAN_POINT ( 'NONE',  ( 6.139770520408368348, 198.4640165459539674, 83.45113791807858661 ) ) ;
#24033=CARTESIAN_POINT ( 'NONE',  ( -4.903702542908602524, 213.8346818373418898, 21.95113791807856884 ) ) ;
#24035=CARTESIAN_POINT ( 'NONE',  ( -3.044812012439970683, 197.4746971517856196, 7.898862081921434353 ) ) ;
#24042=CARTESIAN_POINT ( 'NONE',  ( 9.984503880673420539, 210.2968891136705167, 84.84886208192143897 ) ) ;
#24044=CARTESIAN_POINT ( 'NONE',  ( -6.139770520408369237, 215.5359834540460042, 24.95113791807855819 ) ) ;
#24046=CARTESIAN_POINT ( 'NONE',  ( -7.456977232089471386, 217.1783343296987709, 83.94886208192144750 ) ) ;
#24050=CARTESIAN_POINT ( 'NONE',  ( 6.220909254589536808, 215.4770327129947702, 82.55113791807858092 ) ) ;
#24053=CARTESIAN_POINT ( 'NONE',  ( 6.220909254589536808, 215.4770327129947702, 37.55113791807856671 ) ) ;
#24059=CARTESIAN_POINT ( 'NONE',  ( 12.00000000000000711, 206.9523078486586485, 8.001137918078566003 ) ) ;
#24063=VERTEX_POINT ( 'NONE', #5224 ) ;
#24064=CARTESIAN_POINT ( 'NONE',  ( 8.062137200540822946, 212.9164362838583315, 96.69886208192143329 ) ) ;
#24066=CARTESIAN_POINT ( 'NONE',  ( 12.00000000000000711, 207.0476921513415220, 36.99886208192143044 ) ) ;
#24068=CARTESIAN_POINT ( 'NONE',  ( 3.044812012440130555, 197.4746971517856764, 50.60113791807857808 ) ) ;
#24071=CARTESIAN_POINT ( 'NONE',  ( 2.426778023690075337, 214.6231898156240447, 12.39886208192143613 ) ) ;
#24075=CARTESIAN_POINT ( 'NONE',  ( -0.05014649552828365914, 215.4116977939061144, 90.24886208192144466 ) ) ;
#24076=CARTESIAN_POINT ( 'NONE',  ( 6.500168698208129925, 211.6636982574063381, 31.70113791807857240 ) ) ;
#24083=CARTESIAN_POINT ( 'NONE',  ( -4.903702542908602524, 213.8346818373418898, 96.95113791807857240 ) ) ;
#24087=CARTESIAN_POINT ( 'NONE',  ( 8.015496119326595448, 204.4483345814782638, 70.14886208192142192 ) ) ;
#24092=CARTESIAN_POINT ( 'NONE',  ( 6.139770520408367460, 198.4640165459539389, 14.45113791807856529 ) ) ;
#24096=CARTESIAN_POINT ( 'NONE',  ( -7.456977232089304408, 196.8216656703010301, 75.05113791807858092 ) ) ;
#24097=CARTESIAN_POINT ( 'NONE',  ( 6.220909254589536808, 215.4770327129947987, 100.5511379180785809 ) ) ;
#24101=CARTESIAN_POINT ( 'NONE',  ( 11.98450388067341876, 210.9467285061363953, 102.8488620819214390 ) ) ;
#24102=CARTESIAN_POINT ( 'NONE',  ( 3.753561863808876797, 195.6020594897209719, 64.59886208192142476 ) ) ;
#24104=CARTESIAN_POINT ( 'NONE',  ( -3.044812012439970683, 197.4746971517856196, 64.89886208192145034 ) ) ;
#24105=CARTESIAN_POINT ( 'NONE',  ( 7.456977232089471386, 196.8216656703012006, 7.448862081921435951 ) ) ;
#24107=CARTESIAN_POINT ( 'NONE',  ( -0.05014649552810635652, 196.4853777576173002, 20.75113791807855890 ) ) ;
#24108=CARTESIAN_POINT ( 'NONE',  ( 3.044812012439969795, 216.5253028482143520, 81.39886208192145034 ) ) ;
#24111=CARTESIAN_POINT ( 'NONE',  ( -9.949154985843399857, 217.7087784572769067, 102.9933096652613074 ) ) ;
#24115=CARTESIAN_POINT ( 'NONE',  ( 8.000000000000008882, 207.0476921513415220, 60.99886208192144466 ) ) ;
#24123=CARTESIAN_POINT ( 'NONE',  ( 8.015496119326531499, 209.5516654185219636, 73.85113791807857808 ) ) ;
#24124=SURFACE_STYLE_USAGE ( .BOTH. , #18685 ) ;
#24125=CARTESIAN_POINT ( 'NONE',  ( -9.017078565483988228, 206.7748875732014255, 103.7159841306440313 ) ) ;
#24129=CARTESIAN_POINT ( 'NONE',  ( -8.015496119326597224, 209.5516654185217362, 44.64886208192143613 ) ) ;
#24131=CARTESIAN_POINT ( 'NONE',  ( -3.044812012440131443, 216.5253028482142952, 76.10113791807856387 ) ) ;
#24132=CARTESIAN_POINT ( 'NONE',  ( 9.984503880673470277, 203.7031108863295401, 65.15113791807856103 ) ) ;
#24134=CARTESIAN_POINT ( 'NONE',  ( 7.984503880673485376, 204.3529502787953902, 23.15113791807856458 ) ) ;
#24136=CARTESIAN_POINT ( 'NONE',  ( 10.00000000000000888, 207.8771832641648984, -0.04188241574673567946 ) ) ;
#24138=CARTESIAN_POINT ( 'NONE',  ( -12.00000000000000711, 207.0476921513413515, 51.50113791807856956 ) ) ;
#24140=AXIS2_PLACEMENT_3D ( 'NONE', #24539, #1193, #31864 ) ;
#24141=CARTESIAN_POINT ( 'NONE',  ( 8.062137200540920645, 201.0835637161417822, 95.30113791807858092 ) ) ;
#24142=CARTESIAN_POINT ( 'NONE',  ( -10.00000000000000711, 207.0476921513413515, 66.50113791807856956 ) ) ;
#24143=CARTESIAN_POINT ( 'NONE',  ( 0.05014649552828288198, 194.3824533091408000, 28.74886208192144110 ) ) ;
#24144=CARTESIAN_POINT ( 'NONE',  ( 8.062137200540822946, 212.9164362838583315, 33.69886208192143329 ) ) ;
#24146=CARTESIAN_POINT ( 'NONE',  ( 12.00000000000000711, 206.9523078486586485, 80.00113791807856956 ) ) ;
#24147=CARTESIAN_POINT ( 'NONE',  ( -6.444103211791042618, 211.7408657792732356, 96.80113791807858092 ) ) ;
#24148=CARTESIAN_POINT ( 'NONE',  ( -3.044812012439970683, 197.4746971517856196, 52.89886208192143613 ) ) ;
#24151=CARTESIAN_POINT ( 'NONE',  ( -0.05014649552828442242, 219.6175466908591716, 63.24886208192142334 ) ) ;
#24154=CARTESIAN_POINT ( 'NONE',  ( -2.517493886309087880, 214.5937144450984135, 33.09886208192143897 ) ) ;
#24161=CARTESIAN_POINT ( 'NONE',  ( -6.444103211791042618, 211.7408657792732356, 54.80113791807857382 ) ) ;
#24166=CARTESIAN_POINT ( 'NONE',  ( 3.044812012439969795, 216.5253028482143520, 36.39886208192142902 ) ) ;
#24171=CARTESIAN_POINT ( 'NONE',  ( 4.984841277089891776, 200.2242689037093726, 16.44886208192143684 ) ) ;
#24173=CARTESIAN_POINT ( 'NONE',  ( -10.01549611932653860, 203.7984951890123284, 51.35113791807858519 ) ) ;
#24175=CARTESIAN_POINT ( 'NONE',  ( -3.044812012440131443, 216.5253028482142952, 37.10113791807857098 ) ) ;
#24179=CARTESIAN_POINT ( 'NONE',  ( 0.05014649552828262524, 198.5883022060938572, 103.7488620819214304 ) ) ;
#24182=CARTESIAN_POINT ( 'NONE',  ( -12.01549611932652972, 203.1486557965464499, 15.35113791807856387 ) ) ;
#24185=CARTESIAN_POINT ( 'NONE',  ( 10.01549611932653860, 210.2015048109876716, 61.85113791807857098 ) ) ;
#24186=CARTESIAN_POINT ( 'NONE',  ( -3.135527875058821579, 197.5041725223112223, 35.90113791807856813 ) ) ;
#24189=CARTESIAN_POINT ( 'NONE',  ( -3.753561863808691168, 195.6020594897209435, 101.9011379180785895 ) ) ;
#24190=CARTESIAN_POINT ( 'NONE',  ( 9.984503880673420539, 210.2968891136705736, 9.848862081921435419 ) ) ;
#24193=CARTESIAN_POINT ( 'NONE',  ( 7.456977232089302632, 217.1783343296989131, 52.55113791807856671 ) ) ;
#24195=CARTESIAN_POINT ( 'NONE',  ( 8.118202686958138514, 201.1607312380088501, 19.29886208192143471 ) ) ;
#24198=CARTESIAN_POINT ( 'NONE',  ( -10.00000000000000711, 207.0476921513413515, 84.50113791807856956 ) ) ;
#24204=CARTESIAN_POINT ( 'NONE',  ( 4.903702542908601636, 200.1653181626581102, 26.45113791807857240 ) ) ;
#24206=CARTESIAN_POINT ( 'NONE',  ( -9.984503880673420539, 203.7031108863293980, 5.348862081921433642 ) ) ;
#24213=CARTESIAN_POINT ( 'NONE',  ( -3.044812012439970683, 197.4746971517856196, 85.89886208192143613 ) ) ;
#24215=CARTESIAN_POINT ( 'NONE',  ( 9.984503880673470277, 203.7031108863295401, 26.15113791807856813 ) ) ;
#24217=CARTESIAN_POINT ( 'NONE',  ( -3.662846001189865142, 195.5725841191952838, 76.89886208192143613 ) ) ;
#24221=CARTESIAN_POINT ( 'NONE',  ( -8.118202686958039038, 201.1607312380087080, 90.20113791807857240 ) ) ;
#24224=CARTESIAN_POINT ( 'NONE',  ( -10.00000000000000711, 207.0476921513413515, 36.50113791807857666 ) ) ;
#24229=CARTESIAN_POINT ( 'NONE',  ( -9.736236675707914401, 199.9851607334237542, 24.20113791807856529 ) ) ;
#24233=CARTESIAN_POINT ( 'NONE',  ( 0.05014649552828288198, 194.3824533091408000, 37.74886208192143755 ) ) ;
#24235=CARTESIAN_POINT ( 'NONE',  ( 3.135527875058820690, 216.4958274776887492, 52.40113791807857524 ) ) ;
#24237=CARTESIAN_POINT ( 'NONE',  ( -6.444103211790928043, 202.2591342207265939, 17.19886208192143684 ) ) ;
#24240=CARTESIAN_POINT ( 'NONE',  ( -8.015496119326597224, 209.5516654185217362, 101.6488620819214361 ) ) ;
#24241=CARTESIAN_POINT ( 'NONE',  ( -4.984841277089726574, 200.2242689037092305, 42.05113791807857382 ) ) ;
#24245=CARTESIAN_POINT ( 'NONE',  ( 6.220909254589681581, 198.5229672870052582, 58.44886208192144039 ) ) ;
#24248=CARTESIAN_POINT ( 'NONE',  ( -2.517493886308901807, 199.4062855549015012, 98.90113791807858945 ) ) ;
#24251=CARTESIAN_POINT ( 'NONE',  ( 6.444103211790928043, 211.7408657792734061, 72.69886208192143329 ) ) ;
#24254=CARTESIAN_POINT ( 'NONE',  ( 6.220909254589536808, 215.4770327129947987, 13.55113791807856671 ) ) ;
#24258=CARTESIAN_POINT ( 'NONE',  ( 3.753561863808689836, 218.3979405102790565, 73.40113791807856103 ) ) ;
#24259=CARTESIAN_POINT ( 'NONE',  ( -0.05014649552810635652, 196.4853777576173002, 95.75113791807856956 ) ) ;
#24261=VERTEX_POINT ( 'NONE', #19676 ) ;
#24262=CARTESIAN_POINT ( 'NONE',  ( -10.00000000000000711, 206.9523078486584495, 2.498862081921433997 ) ) ;
#24263=CARTESIAN_POINT ( 'NONE',  ( 12.01549611932659367, 203.1486557965466773, 61.14886208192143613 ) ) ;
#24264=CARTESIAN_POINT ( 'NONE',  ( -8.118202686958138514, 212.8392687619910930, 62.79886208192144181 ) ) ;
#24265=CARTESIAN_POINT ( 'NONE',  ( -12.00000000000000711, 206.9523078486584780, 2.498862081921434442 ) ) ;
#24267=CARTESIAN_POINT ( 'NONE',  ( -3.135527875058821579, 197.5041725223112223, 26.90113791807856813 ) ) ;
#24268=CARTESIAN_POINT ( 'NONE',  ( -9.984503880673420539, 203.7031108863293980, 89.34886208192143897 ) ) ;
#24273=CARTESIAN_POINT ( 'NONE',  ( 7.984503880673422316, 209.6470497212048372, 69.84886208192143897 ) ) ;
#24280=CARTESIAN_POINT ( 'NONE',  ( -8.015496119326531499, 204.4483345814780364, 66.35113791807857808 ) ) ;
#24284=CARTESIAN_POINT ( 'NONE',  ( -9.452103778985696536, 206.1202243157721057, 104.3225283253248392 ) ) ;
#24288=CARTESIAN_POINT ( 'NONE',  ( -2.426778023690076225, 199.3768101843759553, 43.89886208192144323 ) ) ;
#24289=CARTESIAN_POINT ( 'NONE',  ( -3.135527875058821579, 197.5041725223112223, 83.90113791807857524 ) ) ;
#24290=CARTESIAN_POINT ( 'NONE',  ( 8.062137200540920645, 201.0835637161417822, 68.30113791807856671 ) ) ;
#24292=EDGE_CURVE ( 'NONE', #20665, #25118, #26503, .T. ) ;
#24294=CARTESIAN_POINT ( 'NONE',  ( 6.444103211791042618, 202.2591342207267644, 23.30113791807857027 ) ) ;
#24298=CARTESIAN_POINT ( 'NONE',  ( -9.736236675707914401, 199.9851607334237542, 45.20113791807857240 ) ) ;
#24300=CARTESIAN_POINT ( 'NONE',  ( -0.05014649552810635652, 196.4853777576173002, 95.75113791807856956 ) ) ;
#24301=CARTESIAN_POINT ( 'NONE',  ( 3.044812012440130555, 197.4746971517856764, 68.60113791807857808 ) ) ;
#24302=CARTESIAN_POINT ( 'NONE',  ( 0.05014649552828288198, 194.3824533091408000, 31.74886208192143755 ) ) ;
#24303=CARTESIAN_POINT ( 'NONE',  ( 9.984503880673420539, 210.2968891136705736, 33.84886208192143187 ) ) ;
#24305=CARTESIAN_POINT ( 'NONE',  ( -9.736236675707914401, 199.9851607334237542, 81.20113791807858661 ) ) ;
#24307=CARTESIAN_POINT ( 'NONE',  ( -4.984841277089726574, 200.2242689037092305, 99.05113791807858092 ) ) ;
#24309=CARTESIAN_POINT ( 'NONE',  ( 0.05014649552828275708, 196.4853777576173002, 58.74886208192141623 ) ) ;
#24312=CARTESIAN_POINT ( 'NONE',  ( 9.680171189290716072, 214.0920067884432854, 60.69886208192144039 ) ) ;
#24316=CARTESIAN_POINT ( 'NONE',  ( 0.05014649552828262524, 198.5883022060938572, 31.74886208192143755 ) ) ;
#24323=CARTESIAN_POINT ( 'NONE',  ( -0.05014649552807731031, 198.5883022060938572, 50.75113791807857666 ) ) ;
#24325=CARTESIAN_POINT ( 'NONE',  ( -10.00000000000000711, 206.9523078486584495, 29.49886208192143400 ) ) ;
#24329=SHAPE_REPRESENTATION_RELATIONSHIP ( 'NONE' , 'NONE' ,  #21975, #21009 ) ;
#24332=CARTESIAN_POINT ( 'NONE',  ( -2.517493886309087880, 214.5937144450984135, 12.09886208192143364 ) ) ;
#24334=CARTESIAN_POINT ( 'NONE',  ( 8.062137200540920645, 201.0835637161417822, 50.30113791807857382 ) ) ;
#24335=CARTESIAN_POINT ( 'NONE',  ( 10.01549611932653860, 210.2015048109876716, 40.85113791807857098 ) ) ;
#24340=CARTESIAN_POINT ( 'NONE',  ( 4.984841277089891776, 200.2242689037093726, 103.4488620819214475 ) ) ;
#24344=CARTESIAN_POINT ( 'NONE',  ( 12.01549611932652972, 210.8513442034534933, 19.85113791807856387 ) ) ;
#24348=CARTESIAN_POINT ( 'NONE',  ( 10.01549611932653860, 210.2015048109876716, 64.85113791807857808 ) ) ;
#24350=CARTESIAN_POINT ( 'NONE',  ( -0.05014649552810635652, 196.4853777576173002, 41.75113791807856245 ) ) ;
#24354=CARTESIAN_POINT ( 'NONE',  ( -9.736236675708031640, 214.0148392665760753, 5.798862081921434708 ) ) ;
#24355=CARTESIAN_POINT ( 'NONE',  ( -0.05014649552828402690, 217.5146222423826714, 12.24886208192143577 ) ) ;
#24358=CARTESIAN_POINT ( 'NONE',  ( -7.456977232089304408, 196.8216656703010301, 45.05113791807857382 ) ) ;
#24359=CARTESIAN_POINT ( 'NONE',  ( 0.05014649552807626948, 215.4116977939061144, 67.25113791807856956 ) ) ;
#24362=CARTESIAN_POINT ( 'NONE',  ( -3.135527875058982783, 216.4958274776886924, 21.09886208192143897 ) ) ;
#24365=CARTESIAN_POINT ( 'NONE',  ( 10.01549611932653860, 210.2015048109876716, 82.85113791807854966 ) ) ;
#24374=CARTESIAN_POINT ( 'NONE',  ( 0.05014649552807626948, 215.4116977939061144, 22.25113791807856956 ) ) ;
#24376=CARTESIAN_POINT ( 'NONE',  ( -8.118202686958138514, 212.8392687619910930, 5.798862081921434708 ) ) ;
#24384=CARTESIAN_POINT ( 'NONE',  ( -8.118202686958138514, 212.8392687619910930, 92.79886208192144181 ) ) ;
#24386=CARTESIAN_POINT ( 'NONE',  ( -10.00000000000000711, 207.0476921513413515, 27.50113791807856600 ) ) ;
#24388=CARTESIAN_POINT ( 'NONE',  ( -9.736236675708031640, 214.0148392665760753, 74.79886208192142760 ) ) ;
#24393=CARTESIAN_POINT ( 'NONE',  ( 3.135527875058820690, 216.4958274776887492, 94.40113791807857524 ) ) ;
#24397=CARTESIAN_POINT ( 'NONE',  ( 10.00000000000000711, 206.9523078486586201, 41.00113791807856956 ) ) ;
#24404=CARTESIAN_POINT ( 'NONE',  ( 11.98450388067348271, 203.0532714938637753, 17.15113791807856458 ) ) ;
#24406=VECTOR ( 'NONE', #33160, 1000.000000000000227 ) ;
#24409=CARTESIAN_POINT ( 'NONE',  ( -12.01549611932659722, 210.8513442034533227, 32.64886208192143613 ) ) ;
#24411=CARTESIAN_POINT ( 'NONE',  ( 9.984503880673470277, 203.7031108863295401, 53.15113791807857524 ) ) ;
#24413=CARTESIAN_POINT ( 'NONE',  ( -4.984841277089891776, 213.7757310962905990, 8.948862081921433287 ) ) ;
#24417=CARTESIAN_POINT ( 'NONE',  ( -2.517493886309087880, 214.5937144450984135, 102.0988620819214532 ) ) ;
#24419=CARTESIAN_POINT ( 'NONE',  ( 7.984503880673485376, 204.3529502787953902, 38.15113791807856813 ) ) ;
#24423=AXIS2_PLACEMENT_3D ( 'NONE', #23257, #22921, #15252 ) ;
#24424=CARTESIAN_POINT ( 'NONE',  ( -6.139770520408224463, 198.4640165459539389, 62.04886208192142050 ) ) ;
#24427=CARTESIAN_POINT ( 'NONE',  ( 2.426778023690261410, 199.3768101843759837, 95.60113791807857808 ) ) ;
#24431=CARTESIAN_POINT ( 'NONE',  ( -2.517493886309087880, 214.5937144450984135, 69.09886208192143897 ) ) ;
#24433=DIRECTION ( 'NONE',  ( -6.106226635438360972E-16, 0.04769215134144213358, -0.9988620819214358848 ) ) ;
#24435=CARTESIAN_POINT ( 'NONE',  ( -3.135527875058821579, 197.5041725223112223, 11.90113791807856636 ) ) ;
#24439=CARTESIAN_POINT ( 'NONE',  ( 3.753561863808689836, 218.3979405102790565, 76.40113791807856103 ) ) ;
#24440=CARTESIAN_POINT ( 'NONE',  ( -9.984503880673475606, 210.2968891136704315, 93.65113791807857524 ) ) ;
#24441=CARTESIAN_POINT ( 'NONE',  ( -10.47863426674271814, 207.9189531262114770, 102.6635298682156758 ) ) ;
#24443=CARTESIAN_POINT ( 'NONE',  ( 10.01549611932659545, 203.7984951890123853, 4.148862081921434353 ) ) ;
#24444=CARTESIAN_POINT ( 'NONE',  ( -0.05014649552828442242, 219.6175466908591716, 60.24886208192143755 ) ) ;
#24445=CARTESIAN_POINT ( 'NONE',  ( -10.00000000000000711, 206.9523078486584495, 68.49886208192143044 ) ) ;
#24446=CARTESIAN_POINT ( 'NONE',  ( 3.662846001189864698, 218.4274158808046593, 6.398862081921435241 ) ) ;
#24448=CARTESIAN_POINT ( 'NONE',  ( 3.044812012440130555, 197.4746971517856764, 23.60113791807857098 ) ) ;
#24449=CARTESIAN_POINT ( 'NONE',  ( -6.139770520408224463, 198.4640165459539389, 86.04886208192144181 ) ) ;
#24456=CARTESIAN_POINT ( 'NONE',  ( 8.015496119326595448, 204.4483345814782638, 70.14886208192142192 ) ) ;
#24463=CARTESIAN_POINT ( 'NONE',  ( 6.500168698208129925, 211.6636982574063381, 67.70113791807857240 ) ) ;
#24467=CARTESIAN_POINT ( 'NONE',  ( 4.984841277089891776, 200.2242689037093726, 46.44886208192144039 ) ) ;
#24468=CARTESIAN_POINT ( 'NONE',  ( 8.062137200540920645, 201.0835637161417822, 86.30113791807856671 ) ) ;
#24469=CARTESIAN_POINT ( 'NONE',  ( -0.05014649552810635652, 196.4853777576173002, 62.75113791807856956 ) ) ;
#24471=CARTESIAN_POINT ( 'NONE',  ( 8.000000000000008882, 206.9523078486586485, 23.00113791807856600 ) ) ;
#24475=CARTESIAN_POINT ( 'NONE',  ( -11.98450388067348804, 210.9467285061362247, 48.65113791807857524 ) ) ;
#24477=CARTESIAN_POINT ( 'NONE',  ( -8.062137200540920645, 212.9164362838581894, 93.80113791807858092 ) ) ;
#24478=CARTESIAN_POINT ( 'NONE',  ( -10.00000000000000711, 207.0476921513413515, 69.50113791807856956 ) ) ;
#24479=CARTESIAN_POINT ( 'NONE',  ( 0.05014649552828288198, 194.3824533091408000, 34.74886208192142334 ) ) ;
#24480=CARTESIAN_POINT ( 'NONE',  ( -3.135527875058982783, 216.4958274776886924, 36.09886208192143897 ) ) ;
#24482=CARTESIAN_POINT ( 'NONE',  ( -7.375838497908182134, 217.2372850707499765, 81.95113791807858661 ) ) ;
#24483=CARTESIAN_POINT ( 'NONE',  ( 6.444103211791042618, 202.2591342207267644, 95.30113791807858092 ) ) ;
#24484=CARTESIAN_POINT ( 'NONE',  ( 3.135527875058981895, 197.5041725223112792, 58.59886208192143897 ) ) ;
#24488=CARTESIAN_POINT ( 'NONE',  ( -0.05014649552828442242, 219.6175466908591716, 66.24886208192143044 ) ) ;
#24491=CARTESIAN_POINT ( 'NONE',  ( -2.517493886309087880, 214.5937144450984135, 39.09886208192143897 ) ) ;
#24498=CARTESIAN_POINT ( 'NONE',  ( -6.500168698208129925, 202.3363017425936050, 54.20113791807857240 ) ) ;
#24500=CARTESIAN_POINT ( 'NONE',  ( 8.118202686958138514, 201.1607312380088501, 28.29886208192143471 ) ) ;
#24507=CARTESIAN_POINT ( 'NONE',  ( -4.984841277089891776, 213.7757310962905990, 17.94886208192143684 ) ) ;
#24508=CARTESIAN_POINT ( 'NONE',  ( -8.062137200540920645, 212.9164362838581894, 63.80113791807858092 ) ) ;
#24510=CARTESIAN_POINT ( 'NONE',  ( -0.05014649552810635652, 196.4853777576173002, 35.75113791807857666 ) ) ;
#24512=CARTESIAN_POINT ( 'NONE',  ( 2.426778023690261410, 199.3768101843759837, -0.3988620819214340751 ) ) ;
#24516=CARTESIAN_POINT ( 'NONE',  ( 0.05014649552807549926, 219.6175466908591716, 19.25113791807856245 ) ) ;
#24519=CARTESIAN_POINT ( 'NONE',  ( -6.139770520408369237, 215.5359834540460042, 69.95113791807857240 ) ) ;
#24520=CARTESIAN_POINT ( 'NONE',  ( -10.00000000000000711, 207.0476921513413515, 36.50113791807857666 ) ) ;
#24524=CARTESIAN_POINT ( 'NONE',  ( 9.736236675708031640, 199.9851607334238963, 7.298862081921434708 ) ) ;
#24525=CARTESIAN_POINT ( 'NONE',  ( 8.118202686958138514, 201.1607312380088501, 10.29886208192143471 ) ) ;
#24529=CARTESIAN_POINT ( 'NONE',  ( -3.753561863808691168, 195.6020594897209435, 50.90113791807858235 ) ) ;
#24530=CARTESIAN_POINT ( 'NONE',  ( -8.000000000000008882, 207.0476921513413515, 69.50113791807856956 ) ) ;
#24532=CARTESIAN_POINT ( 'NONE',  ( 10.00000000000000711, 207.0476921513415220, 33.99886208192143044 ) ) ;
#24536=CARTESIAN_POINT ( 'NONE',  ( 3.044812012440130555, 197.4746971517856764, 80.60113791807857808 ) ) ;
#24539=CARTESIAN_POINT ( 'NONE',  ( 10.00000000000000888, 207.8771832641648984, -0.04188241574673567946 ) ) ;
#24541=CARTESIAN_POINT ( 'NONE',  ( 6.444103211791042618, 202.2591342207267644, 26.30113791807856316 ) ) ;
#24544=CARTESIAN_POINT ( 'NONE',  ( -3.662846001189865142, 195.5725841191952838, 103.8988620819214361 ) ) ;
#24548=CARTESIAN_POINT ( 'NONE',  ( -6.444103211791042618, 211.7408657792732356, 48.80113791807858092 ) ) ;
#24552=CARTESIAN_POINT ( 'NONE',  ( 9.984503880673420539, 210.2968891136705167, 93.84886208192143897 ) ) ;
#24554=CARTESIAN_POINT ( 'NONE',  ( 3.135527875058820690, 216.4958274776887492, 22.40113791807856458 ) ) ;
#24557=CARTESIAN_POINT ( 'NONE',  ( 3.662846001189864698, 218.4274158808046593, 81.39886208192143613 ) ) ;
#24560=CARTESIAN_POINT ( 'NONE',  ( -0.05014649552810635652, 196.4853777576173002, 95.75113791807856956 ) ) ;
#24563=EDGE_CURVE ( 'NONE', #24261, #28270, #16656, .T. ) ;
#24564=CARTESIAN_POINT ( 'NONE',  ( -0.05014649552810635652, 196.4853777576173002, 35.75113791807857666 ) ) ;
#24571=CARTESIAN_POINT ( 'NONE',  ( -9.736236675707914401, 199.9851607334237542, 18.20113791807856529 ) ) ;
#24576=CARTESIAN_POINT ( 'NONE',  ( -11.98450388067341876, 203.0532714938636047, 41.34886208192143187 ) ) ;
#24578=CARTESIAN_POINT ( 'NONE',  ( 0.05014649552810505201, 217.5146222423826714, 55.25113791807858377 ) ) ;
#24579=CARTESIAN_POINT ( 'NONE',  ( 6.444103211790928043, 211.7408657792734061, 12.69886208192143684 ) ) ;
#24583=CARTESIAN_POINT ( 'NONE',  ( 7.984503880673422316, 209.6470497212048372, 99.84886208192143897 ) ) ;
#24585=ADVANCED_FACE ( 'NONE', ( #20014 ), #29823, .T. ) ;
#24587=CARTESIAN_POINT ( 'NONE',  ( 7.984503880673485376, 204.3529502787953902, 44.15113791807857524 ) ) ;
#24591=FACE_OUTER_BOUND ( 'NONE', #25292, .T. ) ;
#24592=CARTESIAN_POINT ( 'NONE',  ( -6.139770520408224463, 198.4640165459539389, 59.04886208192143471 ) ) ;
#24594=DIRECTION ( 'NONE',  ( 0.000000000000000000, -0.04769215134144031559, 0.9988620819214357738 ) ) ;
#24595=CARTESIAN_POINT ( 'NONE',  ( -4.984841277089726574, 200.2242689037092305, 99.05113791807858092 ) ) ;
#24597=CIRCLE ( 'NONE', #14253, 0.9999999999999915623 ) ;
#24600=CARTESIAN_POINT ( 'NONE',  ( 2.426778023690075337, 214.6231898156240447, 84.39886208192143613 ) ) ;
#24604=CARTESIAN_POINT ( 'NONE',  ( -3.135527875058821579, 197.5041725223112223, 20.90113791807856813 ) ) ;
#24609=CARTESIAN_POINT ( 'NONE',  ( 0.05014649552807549926, 219.6175466908591716, 82.25113791807856956 ) ) ;
#24614=CARTESIAN_POINT ( 'NONE',  ( 0.05014649552828275708, 196.4853777576173002, 4.748862081921434886 ) ) ;
#24615=CARTESIAN_POINT ( 'NONE',  ( 12.01549611932659367, 203.1486557965466773, 58.14886208192143613 ) ) ;
#24616=CARTESIAN_POINT ( 'NONE',  ( -3.044812012439970683, 197.4746971517856196, 76.89886208192143613 ) ) ;
#24617=CARTESIAN_POINT ( 'NONE',  ( 7.456977232089471386, 196.8216656703012006, 10.44886208192143506 ) ) ;
#24619=CARTESIAN_POINT ( 'NONE',  ( -9.984503880673473830, 210.2968891136704315, 21.65113791807856458 ) ) ;
#24620=CARTESIAN_POINT ( 'NONE',  ( 6.139770520408223575, 215.5359834540460611, 87.54886208192142760 ) ) ;
#24626=CARTESIAN_POINT ( 'NONE',  ( -4.984841277089891776, 213.7757310962905990, 74.94886208192143329 ) ) ;
#24634=CARTESIAN_POINT ( 'NONE',  ( -4.903702542908602524, 213.8346818373418898, 66.95113791807857240 ) ) ;
#24637=CARTESIAN_POINT ( 'NONE',  ( -4.903702542908436435, 200.1653181626580249, 47.04886208192144892 ) ) ;
#24638=CARTESIAN_POINT ( 'NONE',  ( 0.05014649552810505201, 217.5146222423826714, 94.25113791807855534 ) ) ;
#24639=CARTESIAN_POINT ( 'NONE',  ( 10.01549611932653860, 210.2015048109876716, 73.85113791807857808 ) ) ;
#24645=CARTESIAN_POINT ( 'NONE',  ( 12.01549611932652972, 210.8513442034534933, 52.85113791807857098 ) ) ;
#24648=CARTESIAN_POINT ( 'NONE',  ( 7.456977232089302632, 217.1783343296989131, 4.551137918078565825 ) ) ;
#24649=CARTESIAN_POINT ( 'NONE',  ( -8.062137200540920645, 212.9164362838581894, 63.80113791807858092 ) ) ;
#24650=CARTESIAN_POINT ( 'NONE',  ( -12.01549611932659722, 210.8513442034533227, 32.64886208192143613 ) ) ;
#24651=CARTESIAN_POINT ( 'NONE',  ( 9.984503880673420539, 210.2968891136705736, 48.84886208192143187 ) ) ;
#24654=CARTESIAN_POINT ( 'NONE',  ( 12.01549611932652972, 210.8513442034534933, 79.85113791807857808 ) ) ;
#24655=CARTESIAN_POINT ( 'NONE',  ( 4.984841277089725686, 213.7757310962907411, 97.55113791807858092 ) ) ;
#24656=CIRCLE ( 'NONE', #11044, 5.999999999999995559 ) ;
#24657=CARTESIAN_POINT ( 'NONE',  ( 6.220909254589681581, 198.5229672870052582, 64.44886208192143329 ) ) ;
#24661=CARTESIAN_POINT ( 'NONE',  ( 9.736236675708031640, 199.9851607334238963, 61.29886208192144892 ) ) ;
#24664=CARTESIAN_POINT ( 'NONE',  ( 8.000000000000008882, 207.0476921513415220, 45.99886208192144466 ) ) ;
#24670=CARTESIAN_POINT ( 'NONE',  ( 8.015496119326531499, 209.5516654185219636, 49.85113791807857808 ) ) ;
#24671=CARTESIAN_POINT ( 'NONE',  ( 6.139770520408223575, 215.5359834540460611, 30.54886208192142760 ) ) ;
#24678=CARTESIAN_POINT ( 'NONE',  ( -6.500168698208244500, 211.6636982574061676, 11.79886208192143648 ) ) ;
#24680=CARTESIAN_POINT ( 'NONE',  ( -10.01549611932653860, 203.7984951890123284, 57.35113791807856387 ) ) ;
#24682=CARTESIAN_POINT ( 'NONE',  ( -6.139770520408369237, 215.5359834540460042, 42.95113791807856529 ) ) ;
#24686=CARTESIAN_POINT ( 'NONE',  ( 8.000000000000008882, 207.0476921513415220, 102.9988620819214304 ) ) ;
#24690=CARTESIAN_POINT ( 'NONE',  ( -3.753561863808691168, 195.6020594897209435, 17.90113791807856458 ) ) ;
#24692=CARTESIAN_POINT ( 'NONE',  ( 10.00000000000000711, 206.9523078486586201, 65.00113791807856956 ) ) ;
#24693=CARTESIAN_POINT ( 'NONE',  ( -6.139770520408368348, 215.5359834540460042, 39.95113791807857950 ) ) ;
#24697=CARTESIAN_POINT ( 'NONE',  ( -11.98450388067341876, 203.0532714938636047, 8.348862081921435419 ) ) ;
#24698=CARTESIAN_POINT ( 'NONE',  ( 10.00000000000000711, 207.0476921513415220, 12.99886208192143400 ) ) ;
#24701=CARTESIAN_POINT ( 'NONE',  ( -9.736236675707914401, 199.9851607334237542, 51.20113791807856529 ) ) ;
#24702=CARTESIAN_POINT ( 'NONE',  ( -4.903702542908602524, 213.8346818373418898, 72.95113791807857240 ) ) ;
#24703=CARTESIAN_POINT ( 'NONE',  ( 8.062137200540822946, 212.9164362838583315, 27.69886208192143684 ) ) ;
#24707=CARTESIAN_POINT ( 'NONE',  ( 10.00000000000000711, 206.9523078486586201, 86.00113791807858377 ) ) ;
#24713=CARTESIAN_POINT ( 'NONE',  ( 0.05014649552807626948, 215.4116977939061144, 19.25113791807856245 ) ) ;
#24716=CARTESIAN_POINT ( 'NONE',  ( 10.01549611932659545, 203.7984951890123853, 1.148862081921433909 ) ) ;
#24719=CARTESIAN_POINT ( 'NONE',  ( -6.500168698208129925, 202.3363017425936050, 45.20113791807857240 ) ) ;
#24722=CARTESIAN_POINT ( 'NONE',  ( -10.01549611932659722, 210.2015048109875011, 92.64886208192143613 ) ) ;
#24724=CARTESIAN_POINT ( 'NONE',  ( 6.220909254589536808, 215.4770327129947702, 34.55113791807855250 ) ) ;
#24727=CARTESIAN_POINT ( 'NONE',  ( 9.680171189290716072, 214.0920067884432854, 78.69886208192143329 ) ) ;
#24734=CARTESIAN_POINT ( 'NONE',  ( 10.00000000000000711, 206.9523078486586201, 95.00113791807856956 ) ) ;
#24737=CARTESIAN_POINT ( 'NONE',  ( -8.062137200540920645, 212.9164362838581894, 33.80113791807857382 ) ) ;
#24744=CARTESIAN_POINT ( 'NONE',  ( 0.05014649552807549926, 219.6175466908591716, 19.25113791807856245 ) ) ;
#24748=CARTESIAN_POINT ( 'NONE',  ( -7.456977232089471386, 217.1783343296987709, 41.94886208192144039 ) ) ;
#24749=CARTESIAN_POINT ( 'NONE',  ( -6.220909254589537696, 198.5229672870051161, 6.051137918078566713 ) ) ;
#24750=CARTESIAN_POINT ( 'NONE',  ( 6.220909254589536808, 215.4770327129947702, 64.55113791807858092 ) ) ;
#24752=CARTESIAN_POINT ( 'NONE',  ( 6.444103211790928043, 211.7408657792734061, 9.698862081921433287 ) ) ;
#24753=PRODUCT_DEFINITION_CONTEXT ( 'detailed design', #31172, 'design' ) ;
#24756=CARTESIAN_POINT ( 'NONE',  ( -8.101690028313589309, 224.0100459381558267, 105.4832055762867782 ) ) ;
#24759=CARTESIAN_POINT ( 'NONE',  ( 2.517493886308900919, 214.5937144450984420, 43.40113791807856813 ) ) ;
#24760=DIRECTION ( 'NONE',  ( 0.5526942671207023539, 0.1536855300543050473, 0.8190908404712123891 ) ) ;
#24764=CARTESIAN_POINT ( 'NONE',  ( -6.220909254589682469, 215.4770327129946850, 65.94886208192144750 ) ) ;
#24767=CARTESIAN_POINT ( 'NONE',  ( -0.05014649552810635652, 196.4853777576173002, -0.2488620819214343305 ) ) ;
#24770=CARTESIAN_POINT ( 'NONE',  ( -2.517493886309087880, 214.5937144450984135, 84.09886208192143897 ) ) ;
#24774=CARTESIAN_POINT ( 'NONE',  ( 3.135527875058820690, 216.4958274776887492, 16.40113791807856813 ) ) ;
#24778=CARTESIAN_POINT ( 'NONE',  ( -9.680171189290831535, 214.0920067884431148, 87.80113791807858092 ) ) ;
#24781=CARTESIAN_POINT ( 'NONE',  ( -10.01549611932653860, 203.7984951890123000, 102.3511379180785781 ) ) ;
#24784=CARTESIAN_POINT ( 'NONE',  ( 11.98450388067341876, 210.9467285061363953, 69.84886208192143897 ) ) ;
#24785=CARTESIAN_POINT ( 'NONE',  ( 3.044812012439969795, 216.5253028482143520, 81.39886208192145034 ) ) ;
#24786=CARTESIAN_POINT ( 'NONE',  ( -3.662846001189865142, 195.5725841191952838, 10.89886208192143613 ) ) ;
#24788=CARTESIAN_POINT ( 'NONE',  ( -8.062137200540920645, 212.9164362838581894, 24.80113791807857027 ) ) ;
#24790=CARTESIAN_POINT ( 'NONE',  ( -0.05014649552828403384, 217.5146222423826714, 87.24886208192143044 ) ) ;
#24795=CARTESIAN_POINT ( 'NONE',  ( -4.903702542908436435, 200.1653181626580249, 68.04886208192144181 ) ) ;
#24803=CARTESIAN_POINT ( 'NONE',  ( -7.984503880673488041, 209.6470497212046098, 72.65113791807856103 ) ) ;
#24806=CARTESIAN_POINT ( 'NONE',  ( 6.444103211790928043, 211.7408657792734061, 51.69886208192144039 ) ) ;
#24811=CARTESIAN_POINT ( 'NONE',  ( -0.05014649552807705357, 194.3824533091408000, 56.75113791807857666 ) ) ;
#24813=CARTESIAN_POINT ( 'NONE',  ( 7.456977232089302632, 217.1783343296989131, 1.551137918078565603 ) ) ;
#24814=CARTESIAN_POINT ( 'NONE',  ( -8.062137200540920645, 212.9164362838581894, 78.80113791807858092 ) ) ;
#24815=CARTESIAN_POINT ( 'NONE',  ( -0.05014649552828442242, 219.6175466908591716, 39.24886208192143755 ) ) ;
#24816=CARTESIAN_POINT ( 'NONE',  ( 6.220909254589680693, 198.5229672870052582, 52.44886208192143329 ) ) ;
#24818=CARTESIAN_POINT ( 'NONE',  ( -11.98450388067348804, 210.9467285061362247, 90.65113791807857524 ) ) ;
#24819=CARTESIAN_POINT ( 'NONE',  ( 2.517493886308900919, 214.5937144450984420, 94.40113791807857524 ) ) ;
#24821=CARTESIAN_POINT ( 'NONE',  ( -10.01549611932659722, 210.2015048109875011, 62.64886208192143613 ) ) ;
#24824=CARTESIAN_POINT ( 'NONE',  ( 9.680171189290716072, 214.0920067884432854, 72.69886208192143329 ) ) ;
#24827=CARTESIAN_POINT ( 'NONE',  ( 4.984841277089891776, 200.2242689037093726, 43.44886208192144039 ) ) ;
#24833=CARTESIAN_POINT ( 'NONE',  ( 0.05014649552807626948, 215.4116977939061144, 61.25113791807857666 ) ) ;
#24835=CARTESIAN_POINT ( 'NONE',  ( 8.118202686958138514, 201.1607312380088501, 43.29886208192143471 ) ) ;
#24841=CARTESIAN_POINT ( 'NONE',  ( -4.903702542908436435, 200.1653181626580249, 26.04886208192144181 ) ) ;
#24842=CARTESIAN_POINT ( 'NONE',  ( -10.01549611932653860, 203.7984951890123284, 60.35113791807857808 ) ) ;
#24843=CARTESIAN_POINT ( 'NONE',  ( -8.118202686958039038, 201.1607312380087080, 42.20113791807857240 ) ) ;
#24846=CARTESIAN_POINT ( 'NONE',  ( -0.05014649552810635652, 196.4853777576173002, 17.75113791807856245 ) ) ;
#24847=CARTESIAN_POINT ( 'NONE',  ( 0.05014649552828262524, 198.5883022060938572, 97.74886208192141623 ) ) ;
#24851=CARTESIAN_POINT ( 'NONE',  ( -7.375838497908182134, 217.2372850707499765, 27.95113791807857240 ) ) ;
#24853=CARTESIAN_POINT ( 'NONE',  ( -8.062137200540920645, 212.9164362838581894, 78.80113791807858092 ) ) ;
#24854=CARTESIAN_POINT ( 'NONE',  ( -0.05014649552810635652, 196.4853777576173002, 47.75113791807856245 ) ) ;
#24857=DIRECTION ( 'NONE',  ( -6.106226635438360972E-16, 0.04769215134144213358, -0.9988620819214358848 ) ) ;
#24858=CARTESIAN_POINT ( 'NONE',  ( 12.01549611932659367, 203.1486557965466773, 1.148862081921433909 ) ) ;
#24859=CARTESIAN_POINT ( 'NONE',  ( -10.01549611932659545, 210.2015048109875011, 23.64886208192143613 ) ) ;
#24862=CARTESIAN_POINT ( 'NONE',  ( -12.01549611932652972, 203.1486557965464499, 60.35113791807857098 ) ) ;
#24863=CARTESIAN_POINT ( 'NONE',  ( 4.984841277089725686, 213.7757310962907411, 67.55113791807856671 ) ) ;
#24864=CARTESIAN_POINT ( 'NONE',  ( -10.00000000000000711, 206.9523078486584495, 35.49886208192143044 ) ) ;
#24867=CARTESIAN_POINT ( 'NONE',  ( 8.118202686958039038, 212.8392687619912635, 85.70113791807858661 ) ) ;
#24873=CARTESIAN_POINT ( 'NONE',  ( 4.903702542908601636, 200.1653181626581102, 29.45113791807856529 ) ) ;
#24876=CARTESIAN_POINT ( 'NONE',  ( 3.135527875058981895, 197.5041725223112792, 13.59886208192143719 ) ) ;
#24879=CARTESIAN_POINT ( 'NONE',  ( -7.984503880673488041, 209.6470497212046098, 51.65113791807857524 ) ) ;
#24885=CARTESIAN_POINT ( 'NONE',  ( 8.062137200540822946, 212.9164362838583315, 87.69886208192144750 ) ) ;
#24887=CARTESIAN_POINT ( 'NONE',  ( -8.062137200540920645, 212.9164362838581894, 30.80113791807856671 ) ) ;
#24889=CARTESIAN_POINT ( 'NONE',  ( -8.062137200540920645, 212.9164362838581894, 21.80113791807856671 ) ) ;
#24895=CARTESIAN_POINT ( 'NONE',  ( 6.139770520408368348, 198.4640165459539674, 92.45113791807857240 ) ) ;
#24898=CARTESIAN_POINT ( 'NONE',  ( -9.984503880673473830, 210.2968891136704315, 42.65113791807856813 ) ) ;
#24904=CARTESIAN_POINT ( 'NONE',  ( 7.375838497908181246, 196.7627149292499666, 17.45113791807856174 ) ) ;
#24911=CARTESIAN_POINT ( 'NONE',  ( 3.753561863808876797, 195.6020594897209719, 43.59886208192143897 ) ) ;
#24912=CARTESIAN_POINT ( 'NONE',  ( -3.135527875058821579, 197.5041725223112223, -0.09886208192143428053 ) ) ;
#24913=CARTESIAN_POINT ( 'NONE',  ( -6.220909254589537696, 198.5229672870051161, 63.05113791807858092 ) ) ;
#24914=CARTESIAN_POINT ( 'NONE',  ( -8.000000000000008882, 206.9523078486584780, 26.49886208192143400 ) ) ;
#24919=CARTESIAN_POINT ( 'NONE',  ( -6.500168698208244500, 211.6636982574061676, 98.79886208192142760 ) ) ;
#24922=CARTESIAN_POINT ( 'NONE',  ( 2.426778023690261410, 199.3768101843759837, 38.60113791807857098 ) ) ;
#24923=CARTESIAN_POINT ( 'NONE',  ( 9.379977934355910207, 208.8253170565643870, -1.014254689207407356 ) ) ;
#24928=CARTESIAN_POINT ( 'NONE',  ( -10.01549611932653860, 203.7984951890123284, 3.351137918078566091 ) ) ;
#24929=CARTESIAN_POINT ( 'NONE',  ( -9.984503880673420539, 203.7031108863293980, 62.34886208192143897 ) ) ;
#24932=CARTESIAN_POINT ( 'NONE',  ( 9.984503880673470277, 203.7031108863295401, -0.8488620819214341973 ) ) ;
#24938=CARTESIAN_POINT ( 'NONE',  ( -8.015496119326597224, 209.5516654185217362, 80.64886208192145034 ) ) ;
#24943=CARTESIAN_POINT ( 'NONE',  ( 6.220909254589536808, 215.4770327129947987, 16.55113791807857027 ) ) ;
#24947=CARTESIAN_POINT ( 'NONE',  ( 0.05014649552807549926, 219.6175466908591716, 91.25113791807856956 ) ) ;
#24949=CARTESIAN_POINT ( 'NONE',  ( -9.998182820724316855, 207.4287148614901071, 102.5187279279133037 ) ) ;
#24951=CARTESIAN_POINT ( 'NONE',  ( 0.05014649552828288198, 194.3824533091408000, 73.74886208192144466 ) ) ;
#24952=CARTESIAN_POINT ( 'NONE',  ( -6.139770520408224463, 198.4640165459539105, 80.04886208192142760 ) ) ;
#24953=CARTESIAN_POINT ( 'NONE',  ( -3.662846001189865142, 195.5725841191952838, 16.89886208192143613 ) ) ;
#24956=CARTESIAN_POINT ( 'NONE',  ( 0.05014649552810505201, 217.5146222423826714, 34.25113791807856956 ) ) ;
#24959=CARTESIAN_POINT ( 'NONE',  ( -8.062137200540822946, 201.0835637161416400, 89.19886208192144750 ) ) ;
#24965=CARTESIAN_POINT ( 'NONE',  ( 6.444103211790928043, 211.7408657792734061, 72.69886208192143329 ) ) ;
#24973=CARTESIAN_POINT ( 'NONE',  ( 6.500168698208129925, 211.6636982574063381, 79.70113791807857240 ) ) ;
#24977=CARTESIAN_POINT ( 'NONE',  ( 6.444103211790928043, 211.7408657792734061, 54.69886208192144039 ) ) ;
#24978=CIRCLE ( 'NONE', #29331, 10.62447292484156947 ) ;
#24986=CARTESIAN_POINT ( 'NONE',  ( 12.01549611932652972, 210.8513442034534933, 58.85113791807857098 ) ) ;
#24989=CARTESIAN_POINT ( 'NONE',  ( 0.05014649552807549926, 219.6175466908591716, 1.251137918078565558 ) ) ;
#24990=CARTESIAN_POINT ( 'NONE',  ( 8.062137200540920645, 201.0835637161417822, 77.30113791807858092 ) ) ;
#24991=CARTESIAN_POINT ( 'NONE',  ( 0.05014649552828288198, 194.3824533091408000, 43.74886208192143755 ) ) ;
#24992=CARTESIAN_POINT ( 'NONE',  ( 3.044812012439969795, 216.5253028482143520, 45.39886208192143613 ) ) ;
#24994=CARTESIAN_POINT ( 'NONE',  ( 3.753561863808689836, 218.3979405102790565, 91.40113791807857524 ) ) ;
#24995=CARTESIAN_POINT ( 'NONE',  ( 10.01549611932653860, 210.2015048109876716, 1.851137918078565203 ) ) ;
#24996=CARTESIAN_POINT ( 'NONE',  ( 0.05014649552828275708, 196.4853777576173002, 55.74886208192143755 ) ) ;
#24998=CARTESIAN_POINT ( 'NONE',  ( -9.680171189290716072, 199.9079932115567146, 71.19886208192144750 ) ) ;
#25001=CARTESIAN_POINT ( 'NONE',  ( 8.000000000000008882, 207.0476921513415220, 42.99886208192143755 ) ) ;
#25007=CARTESIAN_POINT ( 'NONE',  ( 2.426778023690261410, 199.3768101843759837, 62.60113791807857808 ) ) ;
#25010=CARTESIAN_POINT ( 'NONE',  ( -6.139770520408224463, 198.4640165459539389, 44.04886208192143471 ) ) ;
#25015=CARTESIAN_POINT ( 'NONE',  ( 8.015496119326595448, 204.4483345814782638, 25.14886208192143258 ) ) ;
#25016=CARTESIAN_POINT ( 'NONE',  ( 8.118202686958039038, 212.8392687619912635, 61.70113791807857240 ) ) ;
#25018=CARTESIAN_POINT ( 'NONE',  ( -9.984503880673473830, 210.2968891136704315, 42.65113791807856813 ) ) ;
#25021=CARTESIAN_POINT ( 'NONE',  ( 6.139770520408368348, 198.4640165459539674, 20.45113791807855819 ) ) ;
#25022=CARTESIAN_POINT ( 'NONE',  ( -2.426778023690262742, 214.6231898156240163, 10.10113791807856742 ) ) ;
#25026=CARTESIAN_POINT ( 'NONE',  ( 7.456977232089302632, 217.1783343296989131, 25.55113791807857027 ) ) ;
#25029=CARTESIAN_POINT ( 'NONE',  ( -10.00000000000000711, 207.0476921513413515, 75.50113791807858377 ) ) ;
#25030=CARTESIAN_POINT ( 'NONE',  ( -3.135527875058821579, 197.5041725223112223, 47.90113791807857524 ) ) ;
#25033=CARTESIAN_POINT ( 'NONE',  ( -3.662846001189865142, 195.5725841191952838, 13.89886208192143613 ) ) ;
#25034=CARTESIAN_POINT ( 'NONE',  ( 3.135527875058981895, 197.5041725223112792, 16.59886208192143542 ) ) ;
#25037=CARTESIAN_POINT ( 'NONE',  ( 7.456977232089302632, 217.1783343296989131, 61.55113791807858092 ) ) ;
#25038=CARTESIAN_POINT ( 'NONE',  ( 0.05014649552807626948, 215.4116977939061144, 70.25113791807856956 ) ) ;
#25039=CARTESIAN_POINT ( 'NONE',  ( -0.05014649552828403384, 217.5146222423826714, 27.24886208192142689 ) ) ;
#25042=ORIENTED_EDGE ( 'NONE', *, *, #8713, .F. ) ;
#25043=CARTESIAN_POINT ( 'NONE',  ( 9.984503880673470277, 203.7031108863295401, 92.15113791807856103 ) ) ;
#25048=CARTESIAN_POINT ( 'NONE',  ( 6.500168698208129925, 211.6636982574063381, 31.70113791807857240 ) ) ;
#25050=CARTESIAN_POINT ( 'NONE',  ( 6.220909254589681581, 198.5229672870052582, 16.44886208192143329 ) ) ;
#25053=CARTESIAN_POINT ( 'NONE',  ( -4.984841277089726574, 200.2242689037092305, 51.05113791807858092 ) ) ;
#25055=CARTESIAN_POINT ( 'NONE',  ( -6.139770520408224463, 198.4640165459539389, 104.0488620819214276 ) ) ;
#25057=CARTESIAN_POINT ( 'NONE',  ( 0.05014649552810505201, 217.5146222423826714, 34.25113791807856956 ) ) ;
#25059=CARTESIAN_POINT ( 'NONE',  ( 8.062137200540920645, 201.0835637161417822, 20.30113791807856671 ) ) ;
#25063=DIRECTION ( 'NONE',  ( 0.01265860800194867734, -0.08535984102820122488, -0.9962697712884263090 ) ) ;
#25064=CARTESIAN_POINT ( 'NONE',  ( 3.135527875058820690, 216.4958274776887492, 100.4011379180785752 ) ) ;
#25067=CARTESIAN_POINT ( 'NONE',  ( -6.220909254589537696, 198.5229672870051161, 48.05113791807858092 ) ) ;
#25073=CARTESIAN_POINT ( 'NONE',  ( 9.736236675707914401, 214.0148392665762458, 28.70113791807857240 ) ) ;
#25077=CARTESIAN_POINT ( 'NONE',  ( -6.220909254589537696, 198.5229672870051161, 0.05113791807856577637 ) ) ;
#25078=CARTESIAN_POINT ( 'NONE',  ( 3.044812012440130555, 197.4746971517856764, 62.60113791807857098 ) ) ;
#25079=CARTESIAN_POINT ( 'NONE',  ( 7.984503880673422316, 209.6470497212048372, 21.84886208192143542 ) ) ;
#25082=CARTESIAN_POINT ( 'NONE',  ( -0.05014649552807731031, 198.5883022060938572, 2.751137918078566003 ) ) ;
#25084=CARTESIAN_POINT ( 'NONE',  ( 12.01549611932659367, 203.1486557965466773, 85.14886208192143613 ) ) ;
#25089=CARTESIAN_POINT ( 'NONE',  ( 10.00000000000000711, 206.9523078486586201, -0.9988620819214343305 ) ) ;
#25090=CARTESIAN_POINT ( 'NONE',  ( 10.01549611932659545, 203.7984951890123853, 76.14886208192143613 ) ) ;
#25093=CARTESIAN_POINT ( 'NONE',  ( -3.044812012440131443, 216.5253028482142952, 7.101137918078566535 ) ) ;
#25097=CARTESIAN_POINT ( 'NONE',  ( 0.05014649552828262524, 198.5883022060938572, 79.74886208192143044 ) ) ;
#25100=CARTESIAN_POINT ( 'NONE',  ( 7.375838497908012492, 217.2372850707501186, 90.54886208192144181 ) ) ;
#25103=CARTESIAN_POINT ( 'NONE',  ( -9.984503880673475606, 210.2968891136704315, 18.65113791807856458 ) ) ;
#25107=CARTESIAN_POINT ( 'NONE',  ( 9.680171189290831535, 199.9079932115568852, 83.30113791807858092 ) ) ;
#25110=CARTESIAN_POINT ( 'NONE',  ( 12.00000000000000711, 207.0476921513415220, 69.99886208192144466 ) ) ;
#25111=CARTESIAN_POINT ( 'NONE',  ( 9.984503880673420539, 210.2968891136705736, 78.84886208192142476 ) ) ;
#25112=CARTESIAN_POINT ( 'NONE',  ( 12.00000000000000711, 207.0476921513415220, 12.99886208192143400 ) ) ;
#25114=CARTESIAN_POINT ( 'NONE',  ( -3.135527875058821579, 197.5041725223112223, 32.90113791807857524 ) ) ;
#25116=CARTESIAN_POINT ( 'NONE',  ( -8.118202686958138514, 212.8392687619910930, 101.7988620819214418 ) ) ;
#25118=VERTEX_POINT ( 'NONE', #14649 ) ;
#25120=CARTESIAN_POINT ( 'NONE',  ( 7.984503880673422316, 209.6470497212048372, 78.84886208192143897 ) ) ;
#25128=CARTESIAN_POINT ( 'NONE',  ( -7.984503880673488041, 209.6470497212046098, 75.65113791807856103 ) ) ;
#25133=CARTESIAN_POINT ( 'NONE',  ( -2.517493886309087880, 214.5937144450984135, 57.09886208192145318 ) ) ;
#25141=CARTESIAN_POINT ( 'NONE',  ( 9.680171189290831535, 199.9079932115568852, 53.30113791807857382 ) ) ;
#25142=CARTESIAN_POINT ( 'NONE',  ( -10.00000000000000711, 207.0476921513413515, 102.5011379180785838 ) ) ;
#25143=CARTESIAN_POINT ( 'NONE',  ( 6.220909254589536808, 215.4770327129947987, 79.55113791807856671 ) ) ;
#25145=CARTESIAN_POINT ( 'NONE',  ( 12.01549611932659367, 203.1486557965466773, 40.14886208192143613 ) ) ;
#25146=CARTESIAN_POINT ( 'NONE',  ( 10.00000000000000711, 207.0476921513415220, 45.99886208192143755 ) ) ;
#25148=CARTESIAN_POINT ( 'NONE',  ( -11.98450388067348804, 210.9467285061362247, 84.65113791807856103 ) ) ;
#25150=CARTESIAN_POINT ( 'NONE',  ( -8.118202686958039038, 201.1607312380087080, 6.201137918078566180 ) ) ;
#25151=CARTESIAN_POINT ( 'NONE',  ( -10.00000000000000711, 206.9523078486584495, 71.49886208192144466 ) ) ;
#25154=CARTESIAN_POINT ( 'NONE',  ( -12.01549611932659722, 210.8513442034533227, 74.64886208192143613 ) ) ;
#25158=CARTESIAN_POINT ( 'NONE',  ( -8.000000000000008882, 206.9523078486584780, 41.49886208192143755 ) ) ;
#25168=CARTESIAN_POINT ( 'NONE',  ( -6.220909254589682469, 215.4770327129946850, 38.94886208192144039 ) ) ;
#25174=CARTESIAN_POINT ( 'NONE',  ( -6.500168698208244500, 211.6636982574061676, 20.79886208192143826 ) ) ;
#25175=CARTESIAN_POINT ( 'NONE',  ( 6.139770520408368348, 198.4640165459539674, 56.45113791807857950 ) ) ;
#25176=CARTESIAN_POINT ( 'NONE',  ( 3.044812012440130555, 197.4746971517856764, 47.60113791807857098 ) ) ;
#25178=CARTESIAN_POINT ( 'NONE',  ( 10.01549611932653860, 210.2015048109876716, 16.85113791807856032 ) ) ;
#25179=CARTESIAN_POINT ( 'NONE',  ( 6.444103211791042618, 202.2591342207267644, 2.301137918078565825 ) ) ;
#25183=CARTESIAN_POINT ( 'NONE',  ( 11.98450388067348271, 203.0532714938637753, 29.15113791807857169 ) ) ;
#25186=CARTESIAN_POINT ( 'NONE',  ( 9.984503880673470277, 203.7031108863295401, 71.15113791807857524 ) ) ;
#25187=CARTESIAN_POINT ( 'NONE',  ( -8.118202686958039038, 201.1607312380087080, 45.20113791807857240 ) ) ;
#25191=CARTESIAN_POINT ( 'NONE',  ( -12.01549611932659722, 210.8513442034533227, 14.64886208192143258 ) ) ;
#25192=CARTESIAN_POINT ( 'NONE',  ( -10.00000000000000711, 206.9523078486584495, 20.49886208192143755 ) ) ;
#25195=CARTESIAN_POINT ( 'NONE',  ( -0.05014649552807705357, 194.3824533091408000, 62.75113791807856245 ) ) ;
#25196=CARTESIAN_POINT ( 'NONE',  ( 6.500168698208129925, 211.6636982574063381, 82.70113791807858661 ) ) ;
#25198=CARTESIAN_POINT ( 'NONE',  ( 10.00000000000000711, 207.0476921513415220, 36.99886208192143755 ) ) ;
#25210=CARTESIAN_POINT ( 'NONE',  ( 8.015496119326531499, 209.5516654185219636, 31.85113791807857453 ) ) ;
#25214=CARTESIAN_POINT ( 'NONE',  ( 8.118202686958138514, 201.1607312380088501, 10.29886208192143471 ) ) ;
#25218=CARTESIAN_POINT ( 'NONE',  ( 4.984841277089725686, 213.7757310962907411, 52.55113791807858092 ) ) ;
#25222=CARTESIAN_POINT ( 'NONE',  ( 10.00000000000000711, 207.0476921513415220, 99.99886208192143044 ) ) ;
#25224=CARTESIAN_POINT ( 'NONE',  ( 10.00000000000000711, 206.9523078486586201, 32.00113791807856956 ) ) ;
#25227=CARTESIAN_POINT ( 'NONE',  ( -0.05014649552810635652, 196.4853777576173002, 14.75113791807856245 ) ) ;
#25233=CARTESIAN_POINT ( 'NONE',  ( -8.118202686958039038, 201.1607312380087080, 102.2011379180785866 ) ) ;
#25236=CARTESIAN_POINT ( 'NONE',  ( -0.05014649552810635652, 196.4853777576173002, 50.75113791807856956 ) ) ;
#25242=CARTESIAN_POINT ( 'NONE',  ( -3.662846001190052991, 218.4274158808045740, 31.10113791807856742 ) ) ;
#25246=CARTESIAN_POINT ( 'NONE',  ( 6.139770520408223575, 215.5359834540460611, 6.548862081921434708 ) ) ;
#25249=CARTESIAN_POINT ( 'NONE',  ( 3.135527875058820690, 216.4958274776887492, 58.40113791807857524 ) ) ;
#25251=CARTESIAN_POINT ( 'NONE',  ( -2.517493886309087880, 214.5937144450984135, 21.09886208192143897 ) ) ;
#25254=CARTESIAN_POINT ( 'NONE',  ( 8.015496119326531499, 209.5516654185219636, 1.851137918078566091 ) ) ;
#25256=CARTESIAN_POINT ( 'NONE',  ( 7.456977232089471386, 196.8216656703012006, 91.44886208192143329 ) ) ;
#25261=CARTESIAN_POINT ( 'NONE',  ( -3.135527875058821579, 197.5041725223112223, -0.09886208192143428053 ) ) ;
#25263=CARTESIAN_POINT ( 'NONE',  ( 3.044812012439969795, 216.5253028482143520, 72.39886208192143613 ) ) ;
#25266=CARTESIAN_POINT ( 'NONE',  ( -10.00000000000000711, 207.0476921513413515, 3.501137918078566003 ) ) ;
#25269=CARTESIAN_POINT ( 'NONE',  ( -6.220909254589537696, 198.5229672870051161, 93.05113791807853829 ) ) ;
#25271=CARTESIAN_POINT ( 'NONE',  ( -3.135527875058821579, 197.5041725223112223, 77.90113791807857524 ) ) ;
#25274=CARTESIAN_POINT ( 'NONE',  ( -12.01549611932659722, 210.8513442034533227, 86.64886208192143613 ) ) ;
#25277=CARTESIAN_POINT ( 'NONE',  ( 9.984503880673473830, 203.7031108863295401, 20.15113791807856813 ) ) ;
#25281=CARTESIAN_POINT ( 'NONE',  ( -12.01549611932652972, 203.1486557965464499, 87.35113791807857808 ) ) ;
#25284=CARTESIAN_POINT ( 'NONE',  ( 11.98450388067341876, 210.9467285061363953, 72.84886208192143897 ) ) ;
#25285=CARTESIAN_POINT ( 'NONE',  ( -10.01549611932659545, 210.2015048109875011, 77.64886208192143613 ) ) ;
#25286=CARTESIAN_POINT ( 'NONE',  ( 7.375838497908012492, 217.2372850707501186, 12.54886208192143826 ) ) ;
#25288=CARTESIAN_POINT ( 'NONE',  ( -3.044812012440131443, 216.5253028482142952, 37.10113791807857098 ) ) ;
#25290=CARTESIAN_POINT ( 'NONE',  ( -0.05014649552828403384, 217.5146222423826714, 99.24886208192143044 ) ) ;
#25292=EDGE_LOOP ( 'NONE', ( #25042, #32449, #30206, #14010, #29913 ) ) ;
#25294=CARTESIAN_POINT ( 'NONE',  ( -8.015496119326597224, 209.5516654185217362, 80.64886208192145034 ) ) ;
#25303=DIRECTION ( 'NONE',  ( 0.000000000000000000, -0.04769215134144196705, 0.9988620819214357738 ) ) ;
#25304=CARTESIAN_POINT ( 'NONE',  ( 6.500168698208129925, 211.6636982574063381, 82.70113791807858661 ) ) ;
#25308=CARTESIAN_POINT ( 'NONE',  ( -7.984503880673422316, 204.3529502787951628, 56.34886208192144608 ) ) ;
#25309=B_SPLINE_CURVE_WITH_KNOTS ( 'NONE', 3,
 ( #14045, #8274, #6034, #24441 ),
 .UNSPECIFIED., .F., .F.,
 ( 4, 4 ),
 ( 1.680513367352531873E-18, 0.0005135163888283047259 ),
 .UNSPECIFIED. ) ;
#25315=CARTESIAN_POINT ( 'NONE',  ( -12.00000000000000711, 207.0476921513413515, 60.50113791807856956 ) ) ;
#25317=CARTESIAN_POINT ( 'NONE',  ( 7.375838497908181246, 196.7627149292499666, 2.451137918078565736 ) ) ;
#25318=CARTESIAN_POINT ( 'NONE',  ( 6.220909254589536808, 215.4770327129947987, 73.55113791807858092 ) ) ;
#25319=CARTESIAN_POINT ( 'NONE',  ( 0.05014649552828288198, 194.3824533091408000, 46.74886208192143755 ) ) ;
#25320=CARTESIAN_POINT ( 'NONE',  ( -3.135527875058982783, 216.4958274776886924, 51.09886208192143897 ) ) ;
#25322=CARTESIAN_POINT ( 'NONE',  ( 3.753561863808689836, 218.3979405102790565, 85.40113791807856103 ) ) ;
#25324=CARTESIAN_POINT ( 'NONE',  ( -10.00000000000000711, 207.0476921513413515, 6.501137918078566003 ) ) ;
#25325=CARTESIAN_POINT ( 'NONE',  ( 6.220909254589681581, 198.5229672870052582, 70.44886208192144750 ) ) ;
#25328=CARTESIAN_POINT ( 'NONE',  ( 12.01549611932659367, 203.1486557965466773, 70.14886208192142192 ) ) ;
#25331=CARTESIAN_POINT ( 'NONE',  ( 2.426778023690075337, 214.6231898156240447, 54.39886208192144323 ) ) ;
#25339=CARTESIAN_POINT ( 'NONE',  ( -10.00000000000000711, 206.9523078486584495, 44.49886208192143755 ) ) ;
#25345=CARTESIAN_POINT ( 'NONE',  ( -6.444103211790928043, 202.2591342207265939, 29.19886208192143684 ) ) ;
#25346=CARTESIAN_POINT ( 'NONE',  ( -3.044812012440131443, 216.5253028482142952, 67.10113791807857808 ) ) ;
#25348=CARTESIAN_POINT ( 'NONE',  ( 10.00000000000000711, 206.9523078486586201, 44.00113791807857666 ) ) ;
#25350=CARTESIAN_POINT ( 'NONE',  ( -9.984503880673473830, 210.2968891136704315, 21.65113791807856458 ) ) ;
#25351=CARTESIAN_POINT ( 'NONE',  ( 4.903702542908601636, 200.1653181626581102, 5.451137918078566180 ) ) ;
#25354=CARTESIAN_POINT ( 'NONE',  ( -9.736236675707914401, 199.9851607334237542, 27.20113791807857240 ) ) ;
#25357=CARTESIAN_POINT ( 'NONE',  ( 0.05014649552810505201, 217.5146222423826714, 76.25113791807855534 ) ) ;
#25358=CARTESIAN_POINT ( 'NONE',  ( 9.984503880673473830, 203.7031108863295401, 53.15113791807857524 ) ) ;
#25361=CARTESIAN_POINT ( 'NONE',  ( -9.680171189290716072, 199.9079932115567146, 11.19886208192143506 ) ) ;
#25362=CARTESIAN_POINT ( 'NONE',  ( 0.05014649552828275014, 196.4853777576173002, 22.74886208192143400 ) ) ;
#25365=CARTESIAN_POINT ( 'NONE',  ( 3.662846001190051659, 195.5725841191953691, 56.60113791807857808 ) ) ;
#25366=CARTESIAN_POINT ( 'NONE',  ( -4.903702542908602524, 213.8346818373418898, 75.95113791807857240 ) ) ;
#25368=CARTESIAN_POINT ( 'NONE',  ( 10.01549611932659545, 203.7984951890123853, 37.14886208192142192 ) ) ;
#25379=CARTESIAN_POINT ( 'NONE',  ( -2.517493886308901807, 199.4062855549015012, 35.90113791807856813 ) ) ;
#25381=CARTESIAN_POINT ( 'NONE',  ( -10.01549611932659722, 210.2015048109875011, 14.64886208192143258 ) ) ;
#25384=CARTESIAN_POINT ( 'NONE',  ( -4.903702542908602524, 213.8346818373418898, 60.95113791807857240 ) ) ;
#25386=CARTESIAN_POINT ( 'NONE',  ( -10.00000000000000711, 206.9523078486584495, 98.49886208192143044 ) ) ;
#25388=CARTESIAN_POINT ( 'NONE',  ( -8.062137200540920645, 212.9164362838581894, 36.80113791807856671 ) ) ;
#25392=CARTESIAN_POINT ( 'NONE',  ( -10.01549611932653860, 203.7984951890123284, 18.35113791807856742 ) ) ;
#25396=CARTESIAN_POINT ( 'NONE',  ( -6.220909254589537696, 198.5229672870051161, 102.0511379180785383 ) ) ;
#25400=CARTESIAN_POINT ( 'NONE',  ( -6.139770520408369237, 215.5359834540460042, 42.95113791807856529 ) ) ;
#25407=CARTESIAN_POINT ( 'NONE',  ( -12.01549611932652972, 203.1486557965464499, 33.35113791807857098 ) ) ;
#25410=CARTESIAN_POINT ( 'NONE',  ( 9.984503880673420539, 210.2968891136705167, 12.84886208192143187 ) ) ;
#25413=CARTESIAN_POINT ( 'NONE',  ( -0.05014649552810635652, 196.4853777576173002, 2.751137918078565114 ) ) ;
#25414=CARTESIAN_POINT ( 'NONE',  ( -3.135527875058821579, 197.5041725223112223, 56.90113791807857524 ) ) ;
#25417=CARTESIAN_POINT ( 'NONE',  ( -4.984841277089891776, 213.7757310962905990, 23.94886208192143684 ) ) ;
#25421=CARTESIAN_POINT ( 'NONE',  ( -6.500168698208129925, 202.3363017425936050, 6.201137918078567068 ) ) ;
#25423=CARTESIAN_POINT ( 'NONE',  ( -12.01549611932659722, 210.8513442034533227, 92.64886208192143613 ) ) ;
#25428=CARTESIAN_POINT ( 'NONE',  ( -9.984503880673473830, 210.2968891136704315, 0.6511379180785656917 ) ) ;
#25429=CARTESIAN_POINT ( 'NONE',  ( 8.062137200540822946, 212.9164362838583315, 66.69886208192143329 ) ) ;
#25432=CARTESIAN_POINT ( 'NONE',  ( -8.062137200540920645, 212.9164362838581894, 3.801137918078565825 ) ) ;
#25436=CARTESIAN_POINT ( 'NONE',  ( -8.062137200540920645, 212.9164362838581894, 87.80113791807856671 ) ) ;
#25438=CARTESIAN_POINT ( 'NONE',  ( 8.062137200540920645, 201.0835637161417822, 77.30113791807858092 ) ) ;
#25439=AXIS2_PLACEMENT_3D ( 'NONE', #4945, #2890, #15832 ) ;
#25442=CARTESIAN_POINT ( 'NONE',  ( 7.456977232089471386, 196.8216656703012006, 82.44886208192144750 ) ) ;
#25446=CARTESIAN_POINT ( 'NONE',  ( 0.05014649552810506589, 217.5146222423826714, 34.25113791807856956 ) ) ;
#25450=CARTESIAN_POINT ( 'NONE',  ( -12.00000000000000711, 207.0476921513413515, 93.50113791807858377 ) ) ;
#25454=CARTESIAN_POINT ( 'NONE',  ( -8.118202686958138514, 212.8392687619910930, 89.79886208192144181 ) ) ;
#25455=CARTESIAN_POINT ( 'NONE',  ( -0.05014649552828442242, 219.6175466908591716, 27.24886208192143755 ) ) ;
#25457=CARTESIAN_POINT ( 'NONE',  ( 9.984503880673470277, 203.7031108863295401, 32.15113791807857524 ) ) ;
#25459=CARTESIAN_POINT ( 'NONE',  ( 3.135527875058981895, 197.5041725223112792, 100.5988620819214390 ) ) ;
#25463=CARTESIAN_POINT ( 'NONE',  ( -2.517493886309087880, 214.5937144450984135, 81.09886208192143897 ) ) ;
#25468=DIRECTION ( 'NONE',  ( 0.3362851123284906207, 0.04491457122451913281, 0.9406885799869860731 ) ) ;
#25473=CARTESIAN_POINT ( 'NONE',  ( 6.444103211791042618, 202.2591342207267644, 74.30113791807858092 ) ) ;
#25478=CARTESIAN_POINT ( 'NONE',  ( -4.984841277089891776, 213.7757310962905990, 50.94886208192143329 ) ) ;
#25479=CARTESIAN_POINT ( 'NONE',  ( -3.135527875058821579, 197.5041725223112223, 5.901137918078566358 ) ) ;
#25483=CARTESIAN_POINT ( 'NONE',  ( 7.456977232089302632, 217.1783343296989131, 55.55113791807858092 ) ) ;
#25486=CARTESIAN_POINT ( 'NONE',  ( 7.375838497908181246, 196.7627149292499666, 8.451137918078563516 ) ) ;
#25488=CARTESIAN_POINT ( 'NONE',  ( 3.044812012440130555, 197.4746971517856764, 77.60113791807857808 ) ) ;
#25490=CARTESIAN_POINT ( 'NONE',  ( -12.00000000000000711, 206.9523078486584780, 38.49886208192143044 ) ) ;
#25491=CARTESIAN_POINT ( 'NONE',  ( 6.139770520408223575, 215.5359834540460611, 60.54886208192142760 ) ) ;
#25493=CARTESIAN_POINT ( 'NONE',  ( 9.680171189290831535, 199.9079932115568852, 89.30113791807858092 ) ) ;
#25495=CARTESIAN_POINT ( 'NONE',  ( 10.00000000000000711, 206.9523078486586201, 5.001137918078565114 ) ) ;
#25496=CARTESIAN_POINT ( 'NONE',  ( 8.118202686958138514, 201.1607312380088501, 67.29886208192144181 ) ) ;
#25500=CARTESIAN_POINT ( 'NONE',  ( 12.01549611932659367, 203.1486557965466773, 73.14886208192142192 ) ) ;
#25503=CARTESIAN_POINT ( 'NONE',  ( -2.517493886309087880, 214.5937144450984135, 48.09886208192143897 ) ) ;
#25509=AXIS2_PLACEMENT_3D ( 'NONE', #15431, #15591, #28717 ) ;
#25512=CARTESIAN_POINT ( 'NONE',  ( 6.139770520408223575, 215.5359834540460611, 45.54886208192144181 ) ) ;
#25516=CARTESIAN_POINT ( 'NONE',  ( -3.135527875058821579, 197.5041725223112223, 56.90113791807857524 ) ) ;
#25519=CARTESIAN_POINT ( 'NONE',  ( -2.517493886309087880, 214.5937144450984135, 24.09886208192143897 ) ) ;
#25520=CARTESIAN_POINT ( 'NONE',  ( 3.044812012440130555, 197.4746971517856764, 71.60113791807857808 ) ) ;
#25522=CARTESIAN_POINT ( 'NONE',  ( -6.220909254589537696, 198.5229672870051161, 57.05113791807857382 ) ) ;
#25524=CARTESIAN_POINT ( 'NONE',  ( 0.05014649552810505201, 217.5146222423826714, 16.25113791807856600 ) ) ;
#25525=CARTESIAN_POINT ( 'NONE',  ( 7.984503880673485376, 204.3529502787953902, 2.151137918078566802 ) ) ;
#25528=CARTESIAN_POINT ( 'NONE',  ( 12.00000000000000711, 206.9523078486586485, 32.00113791807856956 ) ) ;
#25530=CARTESIAN_POINT ( 'NONE',  ( -10.00000000000000711, 207.0476921513413515, 72.50113791807858377 ) ) ;
#25532=CARTESIAN_POINT ( 'NONE',  ( 6.220909254589536808, 215.4770327129947987, 49.55113791807855961 ) ) ;
#25534=CARTESIAN_POINT ( 'NONE',  ( -3.753561863808878130, 218.3979405102790281, 15.09886208192143719 ) ) ;
#25535=CARTESIAN_POINT ( 'NONE',  ( -6.139770520408224463, 198.4640165459539105, 17.04886208192143471 ) ) ;
#25538=CARTESIAN_POINT ( 'NONE',  ( -9.736236675707914401, 199.9851607334237542, 60.20113791807857240 ) ) ;
#25541=CARTESIAN_POINT ( 'NONE',  ( -2.517493886308901807, 199.4062855549015012, 80.90113791807858945 ) ) ;
#25542=CARTESIAN_POINT ( 'NONE',  ( -8.062137200540822946, 201.0835637161416400, 38.19886208192143329 ) ) ;
#25546=CARTESIAN_POINT ( 'NONE',  ( -12.00000000000000711, 206.9523078486584780, 41.49886208192143044 ) ) ;
#25553=CARTESIAN_POINT ( 'NONE',  ( -4.984841277089726574, 200.2242689037092305, 36.05113791807856671 ) ) ;
#25555=CARTESIAN_POINT ( 'NONE',  ( 9.984503880673420539, 210.2968891136705167, 15.84886208192143719 ) ) ;
#25558=CARTESIAN_POINT ( 'NONE',  ( -2.517493886308901807, 199.4062855549015012, 59.90113791807856813 ) ) ;
#25561=CARTESIAN_POINT ( 'NONE',  ( -0.05014649552828403384, 217.5146222423826714, 96.24886208192144466 ) ) ;
#25564=CARTESIAN_POINT ( 'NONE',  ( -6.220909254589537696, 198.5229672870051161, 42.05113791807857382 ) ) ;
#25566=CARTESIAN_POINT ( 'NONE',  ( -3.135527875058821579, 197.5041725223112223, 20.90113791807856813 ) ) ;
#25572=CARTESIAN_POINT ( 'NONE',  ( -6.139770520408369237, 215.5359834540460042, 99.95113791807855819 ) ) ;
#25575=CARTESIAN_POINT ( 'NONE',  ( 10.00000000000000711, 206.9523078486586201, 47.00113791807856956 ) ) ;
#25582=CARTESIAN_POINT ( 'NONE',  ( -7.375838497908182134, 217.2372850707499765, 33.95113791807856529 ) ) ;
#25584=CARTESIAN_POINT ( 'NONE',  ( 10.01549611932659545, 203.7984951890123853, 16.14886208192143613 ) ) ;
#25588=CARTESIAN_POINT ( 'NONE',  ( -8.062137200540920645, 212.9164362838581894, 9.801137918078566713 ) ) ;
#25589=CARTESIAN_POINT ( 'NONE',  ( 9.984503880673470277, 203.7031108863295401, 74.15113791807854682 ) ) ;
#25591=CARTESIAN_POINT ( 'NONE',  ( 7.984503880673422316, 209.6470497212048372, 18.84886208192143187 ) ) ;
#25594=CARTESIAN_POINT ( 'NONE',  ( 2.426778023690261410, 199.3768101843759837, 5.601137918078567424 ) ) ;
#25596=CARTESIAN_POINT ( 'NONE',  ( -7.375838497908014268, 196.7627149292498530, 86.04886208192145602 ) ) ;
#25601=CARTESIAN_POINT ( 'NONE',  ( 0.05014649552810505201, 217.5146222423826714, 7.251137918078566003 ) ) ;
#25602=CARTESIAN_POINT ( 'NONE',  ( -3.135527875058982783, 216.4958274776886924, 72.09886208192143897 ) ) ;
#25606=CARTESIAN_POINT ( 'NONE',  ( 6.139770520408368348, 198.4640165459539674, 17.45113791807855819 ) ) ;
#25609=CARTESIAN_POINT ( 'NONE',  ( 6.220909254589536808, 215.4770327129947702, 94.55113791807858092 ) ) ;
#25610=CARTESIAN_POINT ( 'NONE',  ( -6.139770520408369237, 215.5359834540460042, 72.95113791807854398 ) ) ;
#25613=CARTESIAN_POINT ( 'NONE',  ( 12.01549611932659367, 203.1486557965466773, 88.14886208192143613 ) ) ;
#25615=CARTESIAN_POINT ( 'NONE',  ( -3.044812012440131443, 216.5253028482142952, 28.10113791807857098 ) ) ;
#25619=CARTESIAN_POINT ( 'NONE',  ( -3.753561863808691168, 195.6020594897209435, 92.90113791807857524 ) ) ;
#25620=CARTESIAN_POINT ( 'NONE',  ( -10.90161837886387808, 206.5319970171666455, 103.9075498093380645 ) ) ;
#25622=CARTESIAN_POINT ( 'NONE',  ( 6.220909254589680693, 198.5229672870052582, 85.44886208192143329 ) ) ;
#25624=CARTESIAN_POINT ( 'NONE',  ( 7.375838497908012492, 217.2372850707501186, 24.54886208192144181 ) ) ;
#25626=CARTESIAN_POINT ( 'NONE',  ( 8.062137200540920645, 201.0835637161417822, 32.30113791807857382 ) ) ;
#25628=CARTESIAN_POINT ( 'NONE',  ( 9.984503880673420539, 210.2968891136705167, 96.84886208192139634 ) ) ;
#25633=CARTESIAN_POINT ( 'NONE',  ( -9.963617232950836566, 205.9538967796982547, 104.4520962529709465 ) ) ;
#25634=CARTESIAN_POINT ( 'NONE',  ( -6.444103211790928043, 202.2591342207265939, 77.19886208192143329 ) ) ;
#25641=CARTESIAN_POINT ( 'NONE',  ( 2.426778023690261410, 199.3768101843759837, 59.60113791807857808 ) ) ;
#25644=CARTESIAN_POINT ( 'NONE',  ( -6.500168698208129925, 202.3363017425936050, 87.20113791807858661 ) ) ;
#25648=CARTESIAN_POINT ( 'NONE',  ( -2.517493886309087880, 214.5937144450984135, 63.09886208192143187 ) ) ;
#25655=CARTESIAN_POINT ( 'NONE',  ( -9.680171189290831535, 214.0920067884431148, 66.80113791807858092 ) ) ;
#25657=CARTESIAN_POINT ( 'NONE',  ( -9.680171189290831535, 214.0920067884431148, 12.80113791807856849 ) ) ;
#25658=CARTESIAN_POINT ( 'NONE',  ( -6.139770520408368348, 215.5359834540460042, 90.95113791807855819 ) ) ;
#25659=CARTESIAN_POINT ( 'NONE',  ( 11.98450388067341876, 210.9467285061363953, 54.84886208192143187 ) ) ;
#25660=CARTESIAN_POINT ( 'NONE',  ( 8.062137200540822946, 212.9164362838583315, 54.69886208192143329 ) ) ;
#25662=CARTESIAN_POINT ( 'NONE',  ( -9.736236675707914401, 199.9851607334237542, 93.20113791807858661 ) ) ;
#25665=CARTESIAN_POINT ( 'NONE',  ( 6.220909254589536808, 215.4770327129947702, 1.551137918078565825 ) ) ;
#25666=CARTESIAN_POINT ( 'NONE',  ( 6.220909254589681581, 198.5229672870052582, 73.44886208192139065 ) ) ;
#25669=CARTESIAN_POINT ( 'NONE',  ( -3.753561863808878130, 218.3979405102790281, 81.09886208192143897 ) ) ;
#25671=CARTESIAN_POINT ( 'NONE',  ( -8.118202686958039038, 201.1607312380087080, 90.20113791807857240 ) ) ;
#25674=CARTESIAN_POINT ( 'NONE',  ( -0.05014649552828365914, 215.4116977939061144, 48.24886208192144466 ) ) ;
#25682=CARTESIAN_POINT ( 'NONE',  ( -8.118202686958138514, 212.8392687619910930, 56.79886208192143471 ) ) ;
#25686=CARTESIAN_POINT ( 'NONE',  ( 6.444103211790928043, 211.7408657792734061, 30.69886208192143684 ) ) ;
#25687=CARTESIAN_POINT ( 'NONE',  ( 9.984503880673470277, 203.7031108863295401, 68.15113791807857524 ) ) ;
#25689=CARTESIAN_POINT ( 'NONE',  ( -8.118202686958039038, 201.1607312380087080, 54.20113791807857240 ) ) ;
#25690=CARTESIAN_POINT ( 'NONE',  ( 3.135527875058820690, 216.4958274776887492, 28.40113791807856813 ) ) ;
#25691=CARTESIAN_POINT ( 'NONE',  ( -6.500168698208129925, 202.3363017425936050, 9.201137918078563516 ) ) ;
#25695=CARTESIAN_POINT ( 'NONE',  ( -12.01549611932652972, 203.1486557965464499, 42.35113791807857098 ) ) ;
#25697=CARTESIAN_POINT ( 'NONE',  ( -10.00000000000000711, 207.0476921513413515, 81.50113791807856956 ) ) ;
#25698=CARTESIAN_POINT ( 'NONE',  ( 6.139770520408367460, 198.4640165459539389, 62.45113791807857950 ) ) ;
#25700=CARTESIAN_POINT ( 'NONE',  ( 12.01549611932659367, 203.1486557965466773, 16.14886208192143613 ) ) ;
#25701=CARTESIAN_POINT ( 'NONE',  ( -10.00000000000000711, 206.9523078486584495, 26.49886208192143755 ) ) ;
#25705=CARTESIAN_POINT ( 'NONE',  ( 3.662846001190051659, 195.5725841191953691, 71.60113791807857808 ) ) ;
#25706=CARTESIAN_POINT ( 'NONE',  ( 6.500168698208129925, 211.6636982574063381, 79.70113791807857240 ) ) ;
#25708=CARTESIAN_POINT ( 'NONE',  ( 8.118202686958138514, 201.1607312380088501, 37.29886208192143471 ) ) ;
#25711=CARTESIAN_POINT ( 'NONE',  ( 7.456977232089471386, 196.8216656703012006, 46.44886208192143329 ) ) ;
#25718=CARTESIAN_POINT ( 'NONE',  ( 0.05014649552807626948, 215.4116977939061144, 43.25113791807856956 ) ) ;
#25721=CARTESIAN_POINT ( 'NONE',  ( -3.044812012439970683, 197.4746971517856196, 19.89886208192143613 ) ) ;
#25728=CARTESIAN_POINT ( 'NONE',  ( -10.01549611932659722, 210.2015048109875011, 95.64886208192140771 ) ) ;
#25730=CARTESIAN_POINT ( 'NONE',  ( 6.139770520408368348, 198.4640165459539674, 41.45113791807857240 ) ) ;
#25732=CARTESIAN_POINT ( 'NONE',  ( -6.139770520408369237, 215.5359834540460042, 30.95113791807857240 ) ) ;
#25733=CARTESIAN_POINT ( 'NONE',  ( 9.984503880673420539, 210.2968891136705736, 99.84886208192142476 ) ) ;
#25734=CARTESIAN_POINT ( 'NONE',  ( -6.500168698208244500, 211.6636982574061676, 80.79886208192144181 ) ) ;
#25738=CARTESIAN_POINT ( 'NONE',  ( -9.680171189290831535, 214.0920067884431148, 9.801137918078564937 ) ) ;
#25741=CARTESIAN_POINT ( 'NONE',  ( 8.118202686958039038, 212.8392687619912635, 52.70113791807857240 ) ) ;
#25744=CARTESIAN_POINT ( 'NONE',  ( 6.139770520408223575, 215.5359834540460611, 3.548862081921434708 ) ) ;
#25747=CARTESIAN_POINT ( 'NONE',  ( -7.375838497908182134, 217.2372850707499765, 24.95113791807856884 ) ) ;
#25749=CARTESIAN_POINT ( 'NONE',  ( 9.984503880673420539, 210.2968891136705167, 15.84886208192143719 ) ) ;
#25754=CARTESIAN_POINT ( 'NONE',  ( 6.139770520408368348, 198.4640165459539674, 8.451137918078565292 ) ) ;
#25755=CARTESIAN_POINT ( 'NONE',  ( -8.118202686958039038, 201.1607312380087080, 69.20113791807858661 ) ) ;
#25758=CARTESIAN_POINT ( 'NONE',  ( -6.444103211790928043, 202.2591342207265939, 29.19886208192143684 ) ) ;
#25763=CARTESIAN_POINT ( 'NONE',  ( -8.000000000000008882, 207.0476921513413515, 6.501137918078566891 ) ) ;
#25765=CARTESIAN_POINT ( 'NONE',  ( -12.01549611932659722, 210.8513442034533227, 86.64886208192143613 ) ) ;
#25770=CARTESIAN_POINT ( 'NONE',  ( 8.118202686958039038, 212.8392687619912635, 7.701137918078566180 ) ) ;
#25773=CARTESIAN_POINT ( 'NONE',  ( -6.139770520408224463, 198.4640165459539389, 71.04886208192139918 ) ) ;
#25776=CARTESIAN_POINT ( 'NONE',  ( 3.044812012440130555, 197.4746971517856764, 8.601137918078565647 ) ) ;
#25783=CARTESIAN_POINT ( 'NONE',  ( 9.984503880673470277, 203.7031108863295401, 98.15113791807858945 ) ) ;
#25785=CARTESIAN_POINT ( 'NONE',  ( 10.01549611932653860, 210.2015048109876716, 79.85113791807853545 ) ) ;
#25789=CARTESIAN_POINT ( 'NONE',  ( 7.375838497908012492, 217.2372850707501186, 84.54886208192144181 ) ) ;
#25795=CARTESIAN_POINT ( 'NONE',  ( -3.662846001190052991, 218.4274158808045740, 100.1011379180785781 ) ) ;
#25800=CARTESIAN_POINT ( 'NONE',  ( 6.139770520408223575, 215.5359834540460611, 87.54886208192142760 ) ) ;
#25801=CARTESIAN_POINT ( 'NONE',  ( 9.680171189290716072, 214.0920067884432854, 21.69886208192144039 ) ) ;
#25803=CARTESIAN_POINT ( 'NONE',  ( -6.220909254589537696, 198.5229672870051161, 39.05113791807856671 ) ) ;
#25806=CARTESIAN_POINT ( 'NONE',  ( 0.05014649552828275708, 196.4853777576173002, 103.7488620819214589 ) ) ;
#25809=CARTESIAN_POINT ( 'NONE',  ( 8.015496119326595448, 204.4483345814782638, 85.14886208192143613 ) ) ;
#25814=VERTEX_POINT ( 'NONE', #29948 ) ;
#25816=CARTESIAN_POINT ( 'NONE',  ( 2.426778023690261410, 199.3768101843759837, 56.60113791807857808 ) ) ;
#25819=CARTESIAN_POINT ( 'NONE',  ( -2.517493886308901807, 199.4062855549015012, 86.90113791807857524 ) ) ;
#25822=CARTESIAN_POINT ( 'NONE',  ( -6.500168698208244500, 211.6636982574061676, 65.79886208192144181 ) ) ;
#25823=EDGE_CURVE ( 'NONE', #16872, #16076, #31481, .T. ) ;
#25830=CARTESIAN_POINT ( 'NONE',  ( -9.736236675707914401, 199.9851607334237542, 66.20113791807857240 ) ) ;
#25833=CARTESIAN_POINT ( 'NONE',  ( -11.98450388067348804, 210.9467285061362247, 6.651137918078566358 ) ) ;
#25835=CARTESIAN_POINT ( 'NONE',  ( -3.135527875058821579, 197.5041725223112223, 89.90113791807857524 ) ) ;
#25836=CARTESIAN_POINT ( 'NONE',  ( 11.98450388067341876, 210.9467285061363953, 51.84886208192144608 ) ) ;
#25837=CARTESIAN_POINT ( 'NONE',  ( -8.118202686958138514, 212.8392687619910930, 56.79886208192143471 ) ) ;
#25839=CARTESIAN_POINT ( 'NONE',  ( -12.00000000000000711, 207.0476921513413515, 99.50113791807856956 ) ) ;
#25841=CARTESIAN_POINT ( 'NONE',  ( -0.05014649552810635652, 196.4853777576173002, 17.75113791807856245 ) ) ;
#25843=CARTESIAN_POINT ( 'NONE',  ( -6.220909254589682469, 215.4770327129946850, 71.94886208192144750 ) ) ;
#25845=CARTESIAN_POINT ( 'NONE',  ( 3.662846001189864698, 218.4274158808046593, 81.39886208192143613 ) ) ;
#25846=CARTESIAN_POINT ( 'NONE',  ( 10.01549611932653860, 210.2015048109876716, 94.85113791807857808 ) ) ;
#25849=CARTESIAN_POINT ( 'NONE',  ( 8.015496119326595448, 204.4483345814782638, 49.14886208192145034 ) ) ;
#25856=CARTESIAN_POINT ( 'NONE',  ( 3.044812012439969795, 216.5253028482143520, 51.39886208192143613 ) ) ;
#25860=CARTESIAN_POINT ( 'NONE',  ( 6.500168698208244500, 202.3363017425938324, 31.29886208192143826 ) ) ;
#25861=CARTESIAN_POINT ( 'NONE',  ( 10.00000000000000711, 206.9523078486586201, 74.00113791807858377 ) ) ;
#25863=CARTESIAN_POINT ( 'NONE',  ( -8.062137200540920645, 212.9164362838581894, 54.80113791807857382 ) ) ;
#25865=CARTESIAN_POINT ( 'NONE',  ( 3.135527875058820690, 216.4958274776887492, 25.40113791807856813 ) ) ;
#25866=CARTESIAN_POINT ( 'NONE',  ( 2.426778023690261410, 199.3768101843759837, 11.60113791807856742 ) ) ;
#25870=CARTESIAN_POINT ( 'NONE',  ( 7.375838497908181246, 196.7627149292499666, 38.45113791807856529 ) ) ;
#25872=CARTESIAN_POINT ( 'NONE',  ( 6.220909254589536808, 215.4770327129947702, 88.55113791807853829 ) ) ;
#25873=CARTESIAN_POINT ( 'NONE',  ( -6.139770520408368348, 215.5359834540460042, 54.95113791807856529 ) ) ;
#25876=CARTESIAN_POINT ( 'NONE',  ( 7.375838497908012492, 217.2372850707501186, 21.54886208192143471 ) ) ;
#25877=CARTESIAN_POINT ( 'NONE',  ( -8.062137200540822946, 201.0835637161416400, 32.19886208192143329 ) ) ;
#25879=CARTESIAN_POINT ( 'NONE',  ( -7.456977232089304408, 196.8216656703010301, 69.05113791807856671 ) ) ;
#25880=CARTESIAN_POINT ( 'NONE',  ( -4.984841277089726574, 200.2242689037092305, 78.05113791807858092 ) ) ;
#25881=CARTESIAN_POINT ( 'NONE',  ( -10.01549611932659722, 210.2015048109875011, 38.64886208192142192 ) ) ;
#25884=CARTESIAN_POINT ( 'NONE',  ( 3.662846001189864698, 218.4274158808046593, 54.39886208192143613 ) ) ;
#25889=ORIENTED_EDGE ( 'NONE', *, *, #15102, .F. ) ;
#25890=CARTESIAN_POINT ( 'NONE',  ( -2.517493886308901807, 199.4062855549015012, 44.90113791807856813 ) ) ;
#25892=CARTESIAN_POINT ( 'NONE',  ( 3.135527875058981895, 197.5041725223112792, 22.59886208192143542 ) ) ;
#25897=CARTESIAN_POINT ( 'NONE',  ( -8.015496119326597224, 209.5516654185217362, 5.648862081921434353 ) ) ;
#25898=CARTESIAN_POINT ( 'NONE',  ( -8.062137200540920645, 212.9164362838581894, 45.80113791807856671 ) ) ;
#25900=CARTESIAN_POINT ( 'NONE',  ( 10.01549611932653860, 210.2015048109876716, 28.85113791807855677 ) ) ;
#25901=CARTESIAN_POINT ( 'NONE',  ( -3.135527875058982783, 216.4958274776886924, 102.0988620819214390 ) ) ;
#25903=CARTESIAN_POINT ( 'NONE',  ( -4.903702542908436435, 200.1653181626580249, 92.04886208192142760 ) ) ;
#25906=CARTESIAN_POINT ( 'NONE',  ( -7.375838497908182134, 217.2372850707499765, 9.951137918078567068 ) ) ;
#25909=CARTESIAN_POINT ( 'NONE',  ( -0.05014649552810635652, 196.4853777576173002, 53.75113791807857666 ) ) ;
#25916=CARTESIAN_POINT ( 'NONE',  ( 11.98450388067348271, 203.0532714938637753, 41.15113791807857524 ) ) ;
#25919=CARTESIAN_POINT ( 'NONE',  ( 3.044812012439969795, 216.5253028482143520, 9.398862081921436129 ) ) ;
#25922=CARTESIAN_POINT ( 'NONE',  ( -3.044812012440131443, 216.5253028482142952, 13.10113791807856742 ) ) ;
#25923=CARTESIAN_POINT ( 'NONE',  ( 8.062137200540920645, 201.0835637161417822, 71.30113791807856671 ) ) ;
#25925=CARTESIAN_POINT ( 'NONE',  ( 4.903702542908435547, 213.8346818373419751, 33.54886208192144181 ) ) ;
#25928=CARTESIAN_POINT ( 'NONE',  ( -7.984503880673488041, 209.6470497212046098, 9.651137918078566358 ) ) ;
#25930=CARTESIAN_POINT ( 'NONE',  ( 3.753561863808876797, 195.6020594897209719, 94.59886208192145318 ) ) ;
#25935=CARTESIAN_POINT ( 'NONE',  ( -3.135527875058821579, 197.5041725223112223, 5.901137918078566358 ) ) ;
#25936=CARTESIAN_POINT ( 'NONE',  ( 3.135527875058981895, 197.5041725223112792, 82.59886208192143897 ) ) ;
#25939=CARTESIAN_POINT ( 'NONE',  ( -9.984503880673473830, 210.2968891136704315, 9.651137918078568134 ) ) ;
#25943=CARTESIAN_POINT ( 'NONE',  ( 0.05014649552810505201, 217.5146222423826714, 100.2511379180785838 ) ) ;
#25945=CARTESIAN_POINT ( 'NONE',  ( -0.05014649552810635652, 196.4853777576173002, 86.75113791807858377 ) ) ;
#25948=CARTESIAN_POINT ( 'NONE',  ( 3.753561863808876797, 195.6020594897209719, 100.5988620819214532 ) ) ;
#25954=CARTESIAN_POINT ( 'NONE',  ( -7.375838497908182134, 217.2372850707499765, 96.95113791807857240 ) ) ;
#25956=CARTESIAN_POINT ( 'NONE',  ( -11.00000000000000355, 206.9999999999998863, 103.5000000000000142 ) ) ;
#25960=CARTESIAN_POINT ( 'NONE',  ( 9.984503880673420539, 210.2968891136705736, 90.84886208192143897 ) ) ;
#25961=CARTESIAN_POINT ( 'NONE',  ( 12.01549611932659367, 203.1486557965466773, 19.14886208192143968 ) ) ;
#25964=CARTESIAN_POINT ( 'NONE',  ( -6.220909254589537696, 198.5229672870051161, 45.05113791807855961 ) ) ;
#25966=CARTESIAN_POINT ( 'NONE',  ( -6.500168698208244500, 211.6636982574061676, 5.798862081921435596 ) ) ;
#25970=CARTESIAN_POINT ( 'NONE',  ( -6.500168698208244500, 211.6636982574061676, 89.79886208192142760 ) ) ;
#25972=CARTESIAN_POINT ( 'NONE',  ( -8.000000000000008882, 207.0476921513413515, 33.50113791807857666 ) ) ;
#25981=CARTESIAN_POINT ( 'NONE',  ( -2.426778023690262742, 214.6231898156240163, 85.10113791807857808 ) ) ;
#25984=AXIS2_PLACEMENT_3D ( 'NONE', #3640, #24433, #11821 ) ;
#25987=CARTESIAN_POINT ( 'NONE',  ( -6.444103211790928043, 202.2591342207265939, 62.19886208192144750 ) ) ;
#25996=CARTESIAN_POINT ( 'NONE',  ( 11.98450388067348271, 203.0532714938637753, 71.15113791807857524 ) ) ;
#25998=CARTESIAN_POINT ( 'NONE',  ( -12.00000000000000711, 207.0476921513413515, 9.501137918078566003 ) ) ;
#25999=CARTESIAN_POINT ( 'NONE',  ( -10.00000000000000711, 207.0476921513413515, 90.50113791807858377 ) ) ;
#26002=CARTESIAN_POINT ( 'NONE',  ( 12.01549611932659367, 203.1486557965466773, 55.14886208192143613 ) ) ;
#26003=CARTESIAN_POINT ( 'NONE',  ( -0.05014649552828402690, 217.5146222423826714, 60.24886208192143044 ) ) ;
#26004=CARTESIAN_POINT ( 'NONE',  ( -9.680171189290831535, 214.0920067884431148, 93.80113791807858092 ) ) ;
#26007=CARTESIAN_POINT ( 'NONE',  ( -3.044812012440131443, 216.5253028482142952, 16.10113791807856742 ) ) ;
#26008=CARTESIAN_POINT ( 'NONE',  ( 3.135527875058981895, 197.5041725223112792, 76.59886208192142476 ) ) ;
#26010=CARTESIAN_POINT ( 'NONE',  ( 9.680171189290716072, 214.0920067884432854, 78.69886208192143329 ) ) ;
#26012=CARTESIAN_POINT ( 'NONE',  ( -10.00000000000000711, 207.0476921513413515, 102.5011379180785838 ) ) ;
#26015=CARTESIAN_POINT ( 'NONE',  ( -4.984841277089891776, 213.7757310962905990, 50.94886208192143329 ) ) ;
#26025=CARTESIAN_POINT ( 'NONE',  ( -6.139770520408224463, 198.4640165459539389, 53.04886208192142050 ) ) ;
#26029=CARTESIAN_POINT ( 'NONE',  ( 4.903702542908435547, 213.8346818373419751, 36.54886208192144892 ) ) ;
#26032=CARTESIAN_POINT ( 'NONE',  ( 9.984503880673470277, 203.7031108863295401, 71.15113791807857524 ) ) ;
#26034=CARTESIAN_POINT ( 'NONE',  ( -0.05014649552810635652, 196.4853777576173002, 59.75113791807857666 ) ) ;
#26036=CARTESIAN_POINT ( 'NONE',  ( 3.044812012440130555, 197.4746971517856764, 29.60113791807856742 ) ) ;
#26037=CARTESIAN_POINT ( 'NONE',  ( 2.426778023690261410, 199.3768101843759837, 17.60113791807856742 ) ) ;
#26041=CARTESIAN_POINT ( 'NONE',  ( -12.01549611932652972, 203.1486557965464499, 36.35113791807856387 ) ) ;
#26043=CARTESIAN_POINT ( 'NONE',  ( 10.01549611932653860, 210.2015048109876716, 85.85113791807857808 ) ) ;
#26044=CARTESIAN_POINT ( 'NONE',  ( 9.984503880673473830, 203.7031108863295401, 59.15113791807857524 ) ) ;
#26045=AXIS2_PLACEMENT_3D ( 'NONE', #19031, #5739, #32137 ) ;
#26046=CARTESIAN_POINT ( 'NONE',  ( 11.98450388067341876, 210.9467285061363953, 27.84886208192143897 ) ) ;
#26047=CARTESIAN_POINT ( 'NONE',  ( 6.139770520408223575, 215.5359834540460611, 27.54886208192143471 ) ) ;
#26049=CARTESIAN_POINT ( 'NONE',  ( 12.00000000000000711, 206.9523078486586485, 68.00113791807856956 ) ) ;
#26050=CARTESIAN_POINT ( 'NONE',  ( -8.015496119326531499, 204.4483345814780364, 90.35113791807857808 ) ) ;
#26051=CARTESIAN_POINT ( 'NONE',  ( -8.118202686958138514, 212.8392687619910930, 50.79886208192143471 ) ) ;
#26054=CARTESIAN_POINT ( 'NONE',  ( -12.00000000000000711, 206.9523078486584780, 50.49886208192143044 ) ) ;
#26061=CARTESIAN_POINT ( 'NONE',  ( 6.139770520408368348, 198.4640165459539674, 68.45113791807858661 ) ) ;
#26064=CARTESIAN_POINT ( 'NONE',  ( -7.984503880673488041, 209.6470497212046098, 42.65113791807857524 ) ) ;
#26067=CARTESIAN_POINT ( 'NONE',  ( -3.135527875058982783, 216.4958274776886924, 24.09886208192143542 ) ) ;
#26073=CARTESIAN_POINT ( 'NONE',  ( -8.000000000000008882, 206.9523078486584780, 8.498862081921435774 ) ) ;
#26074=CARTESIAN_POINT ( 'NONE',  ( 8.118202686958039038, 212.8392687619912635, 37.70113791807857240 ) ) ;
#26076=CARTESIAN_POINT ( 'NONE',  ( -3.044812012440131443, 216.5253028482142952, 31.10113791807856742 ) ) ;
#26077=CARTESIAN_POINT ( 'NONE',  ( 3.044812012439969795, 216.5253028482143520, 99.39886208192145034 ) ) ;
#26079=CARTESIAN_POINT ( 'NONE',  ( -6.444103211790928043, 202.2591342207265939, 89.19886208192144750 ) ) ;
#26083=CARTESIAN_POINT ( 'NONE',  ( -0.05014649552807705357, 194.3824533091408000, 14.75113791807856600 ) ) ;
#26087=CARTESIAN_POINT ( 'NONE',  ( -9.984503880673473830, 210.2968891136704315, 54.65113791807858235 ) ) ;
#26093=CARTESIAN_POINT ( 'NONE',  ( -3.662846001190052991, 218.4274158808045740, 37.10113791807855677 ) ) ;
#26096=CARTESIAN_POINT ( 'NONE',  ( 3.044812012439969795, 216.5253028482143520, 12.39886208192143435 ) ) ;
#26099=CARTESIAN_POINT ( 'NONE',  ( -6.220909254589537696, 198.5229672870051161, 75.05113791807858092 ) ) ;
#26101=CARTESIAN_POINT ( 'NONE',  ( -8.015496119326597224, 209.5516654185217362, 32.64886208192144323 ) ) ;
#26104=CARTESIAN_POINT ( 'NONE',  ( 2.426778023690261410, 199.3768101843759837, 11.60113791807856742 ) ) ;
#26106=CARTESIAN_POINT ( 'NONE',  ( 3.662846001189864698, 218.4274158808046593, 96.39886208192146455 ) ) ;
#26111=CARTESIAN_POINT ( 'NONE',  ( -8.118202686958039038, 201.1607312380087080, 12.20113791807856707 ) ) ;
#26112=CARTESIAN_POINT ( 'NONE',  ( -9.984503880673420539, 203.7031108863293980, 77.34886208192142476 ) ) ;
#26115=CARTESIAN_POINT ( 'NONE',  ( 9.984503880673470277, 203.7031108863295401, 17.15113791807856103 ) ) ;
#26120=CARTESIAN_POINT ( 'NONE',  ( 8.062137200540920645, 201.0835637161417822, 83.30113791807858092 ) ) ;
#26123=CARTESIAN_POINT ( 'NONE',  ( 11.98450388067341876, 210.9467285061363953, 93.84886208192143897 ) ) ;
#26128=CARTESIAN_POINT ( 'NONE',  ( -12.00000000000000711, 207.0476921513413515, 96.50113791807856956 ) ) ;
#26132=CARTESIAN_POINT ( 'NONE',  ( 10.00000000000000711, 207.0476921513415220, 81.99886208192143044 ) ) ;
#26133=CARTESIAN_POINT ( 'NONE',  ( 12.01549611932659367, 203.1486557965466773, 25.14886208192143258 ) ) ;
#26135=CARTESIAN_POINT ( 'NONE',  ( -9.984503880673473830, 210.2968891136704315, 39.65113791807857524 ) ) ;
#26137=CARTESIAN_POINT ( 'NONE',  ( 0.05014649552828262524, 198.5883022060938572, 7.748862081921434886 ) ) ;
#26140=CARTESIAN_POINT ( 'NONE',  ( -2.426778023690076225, 199.3768101843759553, 91.89886208192143613 ) ) ;
#26141=CARTESIAN_POINT ( 'NONE',  ( -6.500168698208129925, 202.3363017425936050, 30.20113791807856529 ) ) ;
#26147=CARTESIAN_POINT ( 'NONE',  ( 8.015496119326531499, 209.5516654185219636, 91.85113791807857808 ) ) ;
#26151=CARTESIAN_POINT ( 'NONE',  ( 4.903702542908435547, 213.8346818373419751, 66.54886208192144181 ) ) ;
#26155=CARTESIAN_POINT ( 'NONE',  ( 6.139770520408367460, 198.4640165459539389, 5.451137918078566180 ) ) ;
#26159=CARTESIAN_POINT ( 'NONE',  ( -9.736236675707914401, 199.9851607334237542, 69.20113791807857240 ) ) ;
#26161=CARTESIAN_POINT ( 'NONE',  ( -8.118202686958039038, 201.1607312380087080, 87.20113791807858661 ) ) ;
#26162=CARTESIAN_POINT ( 'NONE',  ( 7.456977232089471386, 196.8216656703012006, 52.44886208192144039 ) ) ;
#26163=CARTESIAN_POINT ( 'NONE',  ( 9.984503880673420539, 210.2968891136705736, 57.84886208192143897 ) ) ;
#26164=CARTESIAN_POINT ( 'NONE',  ( 3.662846001190051659, 195.5725841191953691, 98.60113791807857808 ) ) ;
#26166=CARTESIAN_POINT ( 'NONE',  ( 10.00000000000000711, 206.9523078486586201, 17.00113791807856600 ) ) ;
#26167=CARTESIAN_POINT ( 'NONE',  ( 9.984503880673420539, 210.2968891136705167, 75.84886208192143897 ) ) ;
#26169=CARTESIAN_POINT ( 'NONE',  ( 7.456977232089471386, 196.8216656703012006, 76.44886208192143329 ) ) ;
#26170=CARTESIAN_POINT ( 'NONE',  ( -6.220909254589537696, 198.5229672870051161, 99.05113791807858092 ) ) ;
#26172=CARTESIAN_POINT ( 'NONE',  ( -2.517493886309087880, 214.5937144450984135, 66.09886208192142476 ) ) ;
#26180=CARTESIAN_POINT ( 'NONE',  ( 7.984503880673485376, 204.3529502787953902, 59.15113791807857524 ) ) ;
#26183=CARTESIAN_POINT ( 'NONE',  ( -10.01549611932659722, 210.2015048109875011, 47.64886208192142192 ) ) ;
#26186=CARTESIAN_POINT ( 'NONE',  ( -6.444103211790928043, 202.2591342207265939, 38.19886208192144750 ) ) ;
#26187=CARTESIAN_POINT ( 'NONE',  ( 6.220909254589536808, 215.4770327129947702, 79.55113791807855250 ) ) ;
#26189=CARTESIAN_POINT ( 'NONE',  ( 0.05014649552810505201, 217.5146222423826714, 55.25113791807858377 ) ) ;
#26192=CARTESIAN_POINT ( 'NONE',  ( -10.01549611932653860, 203.7984951890123284, 27.35113791807856742 ) ) ;
#26193=CARTESIAN_POINT ( 'NONE',  ( 6.444103211791042618, 202.2591342207267644, 14.30113791807856849 ) ) ;
#26197=CARTESIAN_POINT ( 'NONE',  ( 7.456977232089302632, 217.1783343296989131, 43.55113791807857382 ) ) ;
#26199=CARTESIAN_POINT ( 'NONE',  ( -3.135527875058821579, 197.5041725223112223, 83.90113791807857524 ) ) ;
#26200=CARTESIAN_POINT ( 'NONE',  ( 3.044812012440130555, 197.4746971517856764, 56.60113791807857098 ) ) ;
#26201=CARTESIAN_POINT ( 'NONE',  ( 11.98450388067341876, 210.9467285061363953, 24.84886208192143897 ) ) ;
#26202=CARTESIAN_POINT ( 'NONE',  ( 0.05014649552828275014, 196.4853777576173002, 28.74886208192144110 ) ) ;
#26205=CARTESIAN_POINT ( 'NONE',  ( -7.456977232089304408, 196.8216656703010301, 66.05113791807858092 ) ) ;
#26206=CARTESIAN_POINT ( 'NONE',  ( -8.000000000000008882, 207.0476921513413515, 84.50113791807856956 ) ) ;
#26208=CARTESIAN_POINT ( 'NONE',  ( 8.062137200540822946, 212.9164362838583315, 51.69886208192143329 ) ) ;
#26211=CARTESIAN_POINT ( 'NONE',  ( -3.662846001189865142, 195.5725841191952838, 49.89886208192143613 ) ) ;
#26217=CARTESIAN_POINT ( 'NONE',  ( 2.426778023690261410, 199.3768101843759837, 38.60113791807857098 ) ) ;
#26219=CARTESIAN_POINT ( 'NONE',  ( -6.139770520408224463, 198.4640165459539389, 26.04886208192143471 ) ) ;
#26224=CARTESIAN_POINT ( 'NONE',  ( 8.000000000000008882, 207.0476921513415220, 9.998862081921435774 ) ) ;
#26225=CARTESIAN_POINT ( 'NONE',  ( 6.220909254589536808, 215.4770327129947702, 55.55113791807855961 ) ) ;
#26227=CARTESIAN_POINT ( 'NONE',  ( 10.00000000000000711, 206.9523078486586201, 32.00113791807856956 ) ) ;
#26228=DIRECTION ( 'NONE',  ( 0.000000000000000000, -0.9988620819214357738, -0.04769215134144155765 ) ) ;
#26230=CARTESIAN_POINT ( 'NONE',  ( 4.984841277089891776, 200.2242689037093726, 88.44886208192144750 ) ) ;
#26235=CARTESIAN_POINT ( 'NONE',  ( 3.753561863808689836, 218.3979405102790565, 7.401137918078566358 ) ) ;
#26238=ADVANCED_FACE ( 'NONE', ( #787 ), #23336, .T. ) ;
#26239=CARTESIAN_POINT ( 'NONE',  ( -8.118202686958039038, 201.1607312380087080, 57.20113791807857950 ) ) ;
#26241=CARTESIAN_POINT ( 'NONE',  ( 10.01549611932653860, 210.2015048109876716, 31.85113791807857453 ) ) ;
#26247=CARTESIAN_POINT ( 'NONE',  ( -3.662846001190052991, 218.4274158808045740, 43.10113791807857098 ) ) ;
#26251=CARTESIAN_POINT ( 'NONE',  ( -9.984503880673420539, 203.7031108863293980, 17.34886208192143542 ) ) ;
#26256=CARTESIAN_POINT ( 'NONE',  ( 6.220909254589536808, 215.4770327129947702, 70.55113791807856671 ) ) ;
#26263=CARTESIAN_POINT ( 'NONE',  ( -2.426778023690262742, 214.6231898156240163, 13.10113791807856742 ) ) ;
#26265=CARTESIAN_POINT ( 'NONE',  ( -0.05014649552828442242, 219.6175466908591716, 96.24886208192144466 ) ) ;
#26270=CARTESIAN_POINT ( 'NONE',  ( 8.062137200540920645, 201.0835637161417822, 8.301137918078566713 ) ) ;
#26271=CARTESIAN_POINT ( 'NONE',  ( 8.118202686958138514, 201.1607312380088501, 79.29886208192144181 ) ) ;
#26274=CARTESIAN_POINT ( 'NONE',  ( 9.984503880673470277, 203.7031108863295401, 14.15113791807856458 ) ) ;
#26276=CIRCLE ( 'NONE', #18113, 1.000000000000000000 ) ;
#26278=CARTESIAN_POINT ( 'NONE',  ( -6.220909254589537696, 198.5229672870051161, 96.05113791807858092 ) ) ;
#26279=CARTESIAN_POINT ( 'NONE',  ( -6.139770520408369237, 215.5359834540460042, 87.95113791807858661 ) ) ;
#26282=CARTESIAN_POINT ( 'NONE',  ( -3.753561863808878130, 218.3979405102790281, 99.09886208192145318 ) ) ;
#26288=CARTESIAN_POINT ( 'NONE',  ( 9.680171189290831535, 199.9079932115568852, 101.3011379180785951 ) ) ;
#26293=CARTESIAN_POINT ( 'NONE',  ( 6.220909254589680693, 198.5229672870052582, 97.44886208192143329 ) ) ;
#26294=CARTESIAN_POINT ( 'NONE',  ( -12.00000000000000711, 206.9523078486584780, 29.49886208192143400 ) ) ;
#26296=CARTESIAN_POINT ( 'NONE',  ( 6.139770520408368348, 198.4640165459539674, 44.45113791807855819 ) ) ;
#26298=CARTESIAN_POINT ( 'NONE',  ( -9.984503880673420539, 203.7031108863293980, 104.3488620819214105 ) ) ;
#26303=CARTESIAN_POINT ( 'NONE',  ( 6.500168698208244500, 202.3363017425938324, 94.29886208192142760 ) ) ;
#26304=CARTESIAN_POINT ( 'NONE',  ( 7.984503880673485376, 204.3529502787953902, 26.15113791807857169 ) ) ;
#26312=CARTESIAN_POINT ( 'NONE',  ( -8.000000000000008882, 207.0476921513413515, 87.50113791807856956 ) ) ;
#26316=CARTESIAN_POINT ( 'NONE',  ( 2.517493886309087436, 199.4062855549015865, 61.59886208192145318 ) ) ;
#26320=CARTESIAN_POINT ( 'NONE',  ( -8.118202686958039038, 201.1607312380087080, 15.20113791807856884 ) ) ;
#26325=CARTESIAN_POINT ( 'NONE',  ( 9.736236675707914401, 214.0148392665762458, 73.70113791807857240 ) ) ;
#26327=CARTESIAN_POINT ( 'NONE',  ( 6.220909254589536808, 215.4770327129947987, 88.55113791807855250 ) ) ;
#26328=DIRECTION ( 'NONE',  ( -0.1461455375466716444, 0.9854922318508084755, -0.08629335326029916042 ) ) ;
#26330=CARTESIAN_POINT ( 'NONE',  ( 3.753561863808876797, 195.6020594897209719, 55.59886208192143897 ) ) ;
#26331=CARTESIAN_POINT ( 'NONE',  ( 3.135527875058981895, 197.5041725223112792, 70.59886208192143897 ) ) ;
#26332=CARTESIAN_POINT ( 'NONE',  ( 11.98450388067348271, 203.0532714938637753, 92.15113791807856103 ) ) ;
#26334=CARTESIAN_POINT ( 'NONE',  ( -8.062137200540920645, 212.9164362838581894, 15.80113791807856849 ) ) ;
#26336=CARTESIAN_POINT ( 'NONE',  ( -3.135527875058982783, 216.4958274776886924, 81.09886208192143897 ) ) ;
#26339=CARTESIAN_POINT ( 'NONE',  ( -3.044812012440131443, 216.5253028482142952, 100.1011379180785781 ) ) ;
#26343=CARTESIAN_POINT ( 'NONE',  ( 2.517493886309087436, 199.4062855549015865, 64.59886208192142476 ) ) ;
#26351=CARTESIAN_POINT ( 'NONE',  ( 6.500168698208129925, 211.6636982574063381, 61.70113791807857240 ) ) ;
#26354=CIRCLE ( 'NONE', #2443, 1.000000000000000222 ) ;
#26357=CARTESIAN_POINT ( 'NONE',  ( 6.444103211790928043, 211.7408657792734061, 36.69886208192144039 ) ) ;
#26358=CARTESIAN_POINT ( 'NONE',  ( -9.984503880673473830, 210.2968891136704315, 75.65113791807858945 ) ) ;
#26360=CARTESIAN_POINT ( 'NONE',  ( 0.05014649552810505201, 217.5146222423826714, 61.25113791807856245 ) ) ;
#26361=CARTESIAN_POINT ( 'NONE',  ( -8.062137200540920645, 212.9164362838581894, 24.80113791807857027 ) ) ;
#26362=CARTESIAN_POINT ( 'NONE',  ( 7.984503880673485376, 204.3529502787953902, 17.15113791807856458 ) ) ;
#26366=CARTESIAN_POINT ( 'NONE',  ( 9.736236675707914401, 214.0148392665762458, 34.70113791807856529 ) ) ;
#26368=CARTESIAN_POINT ( 'NONE',  ( 8.118202686958039038, 212.8392687619912635, 85.70113791807858661 ) ) ;
#26369=CARTESIAN_POINT ( 'NONE',  ( 3.135527875058820690, 216.4958274776887492, 61.40113791807857524 ) ) ;
#26370=CARTESIAN_POINT ( 'NONE',  ( -9.736236675708031640, 214.0148392665760753, 20.79886208192143826 ) ) ;
#26371=CARTESIAN_POINT ( 'NONE',  ( -8.118202686958138514, 212.8392687619910930, 38.79886208192143471 ) ) ;
#26373=CARTESIAN_POINT ( 'NONE',  ( 12.01549611932652972, 210.8513442034534933, 67.85113791807857808 ) ) ;
#26374=CARTESIAN_POINT ( 'NONE',  ( -4.984841277089726574, 200.2242689037092305, 90.05113791807858092 ) ) ;
#26375=CARTESIAN_POINT ( 'NONE',  ( 9.984503880673420539, 210.2968891136705167, 54.84886208192141765 ) ) ;
#26376=ADVANCED_FACE ( 'NONE', ( #5887 ), #3334, .T. ) ;
#26378=CARTESIAN_POINT ( 'NONE',  ( -3.753561863808878130, 218.3979405102790281, 54.09886208192143897 ) ) ;
#26386=CARTESIAN_POINT ( 'NONE',  ( -4.984841277089726574, 200.2242689037092305, 42.05113791807857382 ) ) ;
#26388=CARTESIAN_POINT ( 'NONE',  ( -9.984503880673420539, 203.7031108863293980, 23.34886208192142831 ) ) ;
#26394=CARTESIAN_POINT ( 'NONE',  ( -8.000000000000008882, 206.9523078486584780, 5.498862081921434886 ) ) ;
#26395=CARTESIAN_POINT ( 'NONE',  ( 10.01549611932653860, 210.2015048109876716, 46.85113791807856387 ) ) ;
#26398=CARTESIAN_POINT ( 'NONE',  ( -10.01549611932653860, 203.7984951890123284, 24.35113791807855677 ) ) ;
#26400=CARTESIAN_POINT ( 'NONE',  ( 4.984841277089891776, 200.2242689037093726, 94.44886208192143329 ) ) ;
#26403=CARTESIAN_POINT ( 'NONE',  ( 10.00000000000000711, 207.0000000000000853, 0.000000000000000000 ) ) ;
#26404=CARTESIAN_POINT ( 'NONE',  ( 7.375838497908181246, 196.7627149292499666, 11.45113791807856529 ) ) ;
#26408=CARTESIAN_POINT ( 'NONE',  ( -3.044812012440131443, 216.5253028482142952, 58.10113791807857808 ) ) ;
#26409=CARTESIAN_POINT ( 'NONE',  ( 3.135527875058820690, 216.4958274776887492, 25.40113791807856813 ) ) ;
#26415=CARTESIAN_POINT ( 'NONE',  ( 12.01549611932652972, 210.8513442034534933, 37.85113791807856387 ) ) ;
#26417=CARTESIAN_POINT ( 'NONE',  ( 8.118202686958138514, 201.1607312380088501, 25.29886208192143826 ) ) ;
#26420=CARTESIAN_POINT ( 'NONE',  ( -8.118202686958039038, 201.1607312380087080, 78.20113791807857240 ) ) ;
#26425=CARTESIAN_POINT ( 'NONE',  ( -8.000000000000008882, 207.0476921513413515, 9.501137918078566003 ) ) ;
#26427=CARTESIAN_POINT ( 'NONE',  ( 12.01549611932659367, 203.1486557965466773, 94.14886208192145034 ) ) ;
#26433=CARTESIAN_POINT ( 'NONE',  ( -0.05014649552828403384, 217.5146222423826714, 81.24886208192140202 ) ) ;
#26435=CARTESIAN_POINT ( 'NONE',  ( 6.139770520408368348, 198.4640165459539674, 20.45113791807855819 ) ) ;
#26439=CARTESIAN_POINT ( 'NONE',  ( -9.984503880673473830, 210.2968891136704315, 99.65113791807853261 ) ) ;
#26441=CARTESIAN_POINT ( 'NONE',  ( 3.044812012440130555, 197.4746971517856764, 83.60113791807857808 ) ) ;
#26445=CARTESIAN_POINT ( 'NONE',  ( 7.375838497908012492, 217.2372850707501186, 96.54886208192142760 ) ) ;
#26454=CARTESIAN_POINT ( 'NONE',  ( -3.135527875058982783, 216.4958274776886924, 93.09886208192145318 ) ) ;
#26455=CARTESIAN_POINT ( 'NONE',  ( -9.736236675708031640, 214.0148392665760753, 29.79886208192143826 ) ) ;
#26457=CARTESIAN_POINT ( 'NONE',  ( 10.00000000000000711, 206.9523078486586201, 41.00113791807856956 ) ) ;
#26459=CARTESIAN_POINT ( 'NONE',  ( 2.426778023690075337, 214.6231898156240447, 6.398862081921435241 ) ) ;
#26463=CARTESIAN_POINT ( 'NONE',  ( 4.903702542908435547, 213.8346818373419751, 90.54886208192144181 ) ) ;
#26465=CARTESIAN_POINT ( 'NONE',  ( -2.517493886308901807, 199.4062855549015012, 32.90113791807857524 ) ) ;
#26472=CARTESIAN_POINT ( 'NONE',  ( -0.05014649552807731031, 198.5883022060938572, 98.75113791807856956 ) ) ;
#26475=CARTESIAN_POINT ( 'NONE',  ( 6.444103211790928043, 211.7408657792734061, 69.69886208192143329 ) ) ;
#26479=CARTESIAN_POINT ( 'NONE',  ( 9.984503880673473830, 203.7031108863295401, 11.15113791807856458 ) ) ;
#26484=CARTESIAN_POINT ( 'NONE',  ( -12.00000000000000711, 207.0476921513413515, 72.50113791807856956 ) ) ;
#26486=CARTESIAN_POINT ( 'NONE',  ( -0.05014649552810635652, 196.4853777576173002, 98.75113791807855534 ) ) ;
#26490=CARTESIAN_POINT ( 'NONE',  ( -12.01549611932659722, 210.8513442034533227, 65.64886208192142192 ) ) ;
#26491=CARTESIAN_POINT ( 'NONE',  ( -6.139770520408224463, 198.4640165459539105, 68.04886208192144181 ) ) ;
#26492=CARTESIAN_POINT ( 'NONE',  ( -3.753561863808878130, 218.3979405102790281, 3.098862081921434530 ) ) ;
#26494=CARTESIAN_POINT ( 'NONE',  ( 10.01549611932653860, 210.2015048109876716, 13.85113791807856742 ) ) ;
#26495=CARTESIAN_POINT ( 'NONE',  ( -8.118202686958138514, 212.8392687619910930, 80.79886208192144181 ) ) ;
#26496=ORIENTED_EDGE ( 'NONE', *, *, #29362, .F. ) ;
#26497=CARTESIAN_POINT ( 'NONE',  ( 9.984503880673470277, 203.7031108863295401, 101.1511379180785752 ) ) ;
#26500=CARTESIAN_POINT ( 'NONE',  ( 7.984503880673422316, 209.6470497212048372, 63.84886208192143187 ) ) ;
#26503=CIRCLE ( 'NONE', #15103, 3.999999999999996003 ) ;
#26508=CARTESIAN_POINT ( 'NONE',  ( 6.444103211791042618, 202.2591342207267644, 62.30113791807858092 ) ) ;
#26509=CIRCLE ( 'NONE', #22733, 0.9999999999999968914 ) ;
#26512=CARTESIAN_POINT ( 'NONE',  ( -8.015496119326597224, 209.5516654185217362, 47.64886208192145034 ) ) ;
#26513=CARTESIAN_POINT ( 'NONE',  ( 10.00000000000000711, 206.9523078486586201, 80.00113791807856956 ) ) ;
#26516=CARTESIAN_POINT ( 'NONE',  ( 9.984503880673470277, 203.7031108863295401, 68.15113791807857524 ) ) ;
#26518=CARTESIAN_POINT ( 'NONE',  ( -6.444103211791042618, 211.7408657792732356, 12.80113791807856849 ) ) ;
#26521=CARTESIAN_POINT ( 'NONE',  ( 7.456977232089302632, 217.1783343296989131, 52.55113791807856671 ) ) ;
#26524=CARTESIAN_POINT ( 'NONE',  ( -10.00000000000000711, 207.0476921513413515, 99.50113791807856956 ) ) ;
#26525=CARTESIAN_POINT ( 'NONE',  ( 10.01549611932653860, 210.2015048109876716, 70.85113791807856387 ) ) ;
#26527=CARTESIAN_POINT ( 'NONE',  ( -3.753561863808878130, 218.3979405102790281, 27.09886208192143897 ) ) ;
#26528=CARTESIAN_POINT ( 'NONE',  ( 3.135527875058981895, 197.5041725223112792, 37.59886208192143187 ) ) ;
#26530=CARTESIAN_POINT ( 'NONE',  ( 7.456977232089302632, 217.1783343296989131, 73.55113791807856671 ) ) ;
#26531=CARTESIAN_POINT ( 'NONE',  ( 0.05014649552807626948, 215.4116977939061144, 85.25113791807856956 ) ) ;
#26532=CARTESIAN_POINT ( 'NONE',  ( -10.00000000000000711, 206.9523078486584495, 47.49886208192143755 ) ) ;
#26536=CARTESIAN_POINT ( 'NONE',  ( -9.736236675708031640, 214.0148392665760753, 47.79886208192143471 ) ) ;
#26537=EDGE_LOOP ( 'NONE', ( #21849, #6010, #28621, #20698 ) ) ;
#26542=CARTESIAN_POINT ( 'NONE',  ( -0.05014649552807731031, 198.5883022060938572, 47.75113791807856245 ) ) ;
#26544=CARTESIAN_POINT ( 'NONE',  ( 0.05014649552828275708, 196.4853777576173002, 34.74886208192143044 ) ) ;
#26549=CARTESIAN_POINT ( 'NONE',  ( 2.517493886309087436, 199.4062855549015865, 10.59886208192143542 ) ) ;
#26550=CARTESIAN_POINT ( 'NONE',  ( 0.05014649552810505201, 217.5146222423826714, 52.25113791807856245 ) ) ;
#26553=CARTESIAN_POINT ( 'NONE',  ( 10.00000000000000711, 206.9523078486586201, 38.00113791807857666 ) ) ;
#26556=CARTESIAN_POINT ( 'NONE',  ( 6.500168698208244500, 202.3363017425938324, 91.29886208192142760 ) ) ;
#26560=CARTESIAN_POINT ( 'NONE',  ( 12.00000000000000711, 206.9523078486586485, 17.00113791807856956 ) ) ;
#26563=CARTESIAN_POINT ( 'NONE',  ( -10.00000000000000711, 207.0476921513413515, 66.50113791807856956 ) ) ;
#26564=CARTESIAN_POINT ( 'NONE',  ( -8.118202686958039038, 201.1607312380087080, 33.20113791807857240 ) ) ;
#26568=CARTESIAN_POINT ( 'NONE',  ( 8.062137200540822946, 212.9164362838583315, 9.698862081921435063 ) ) ;
#26571=CARTESIAN_POINT ( 'NONE',  ( 7.456977232089302632, 217.1783343296989131, 37.55113791807855961 ) ) ;
#26574=CARTESIAN_POINT ( 'NONE',  ( -6.220909254589682469, 215.4770327129946850, 23.94886208192142618 ) ) ;
#26580=CARTESIAN_POINT ( 'NONE',  ( -10.00000000000000711, 207.0476921513413515, 78.50113791807856956 ) ) ;
#26585=CARTESIAN_POINT ( 'NONE',  ( -0.05014649552807731031, 198.5883022060938572, 14.75113791807856600 ) ) ;
#26588=CARTESIAN_POINT ( 'NONE',  ( 6.220909254589681581, 198.5229672870052582, 4.448862081921432399 ) ) ;
#26596=CARTESIAN_POINT ( 'NONE',  ( 10.01549611932659545, 203.7984951890123853, 82.14886208192140771 ) ) ;
#26598=CARTESIAN_POINT ( 'NONE',  ( 8.062137200540920645, 201.0835637161417822, 20.30113791807856671 ) ) ;
#26601=CARTESIAN_POINT ( 'NONE',  ( 12.00000000000000711, 207.0476921513415220, 81.99886208192144466 ) ) ;
#26602=CARTESIAN_POINT ( 'NONE',  ( -4.903702542908436435, 200.1653181626580249, 35.04886208192144181 ) ) ;
#26606=CARTESIAN_POINT ( 'NONE',  ( -8.118202686958039038, 201.1607312380087080, 84.20113791807858661 ) ) ;
#26609=CARTESIAN_POINT ( 'NONE',  ( 3.135527875058820690, 216.4958274776887492, 34.40113791807856813 ) ) ;
#26615=CARTESIAN_POINT ( 'NONE',  ( 9.736236675707914401, 214.0148392665762458, 10.70113791807856529 ) ) ;
#26619=CARTESIAN_POINT ( 'NONE',  ( 3.135527875058981895, 197.5041725223112792, 91.59886208192143897 ) ) ;
#26620=CARTESIAN_POINT ( 'NONE',  ( -12.00000000000000711, 206.9523078486584780, 35.49886208192143044 ) ) ;
#26623=CARTESIAN_POINT ( 'NONE',  ( -6.139770520408369237, 215.5359834540460042, 48.95113791807855108 ) ) ;
#26626=CARTESIAN_POINT ( 'NONE',  ( -4.984841277089891776, 213.7757310962905990, 17.94886208192143684 ) ) ;
#26629=CARTESIAN_POINT ( 'NONE',  ( 6.444103211790928043, 211.7408657792734061, 87.69886208192144750 ) ) ;
#26632=CARTESIAN_POINT ( 'NONE',  ( 2.517493886308900919, 214.5937144450984420, 34.40113791807856813 ) ) ;
#26638=CARTESIAN_POINT ( 'NONE',  ( 8.000000000000008882, 206.9523078486586485, 95.00113791807856956 ) ) ;
#26641=CARTESIAN_POINT ( 'NONE',  ( 2.426778023690075337, 214.6231898156240447, 75.39886208192143613 ) ) ;
#26644=CARTESIAN_POINT ( 'NONE',  ( -9.984503880673475606, 210.2968891136704315, 12.65113791807856458 ) ) ;
#26648=CARTESIAN_POINT ( 'NONE',  ( -12.00000000000000711, 207.0476921513413515, 78.50113791807856956 ) ) ;
#26652=CARTESIAN_POINT ( 'NONE',  ( 6.139770520408367460, 198.4640165459539389, 98.45113791807857240 ) ) ;
#26655=CARTESIAN_POINT ( 'NONE',  ( -11.98450388067341876, 203.0532714938636047, 104.3488620819214532 ) ) ;
#26656=CARTESIAN_POINT ( 'NONE',  ( -3.662846001189865142, 195.5725841191952838, 58.89886208192143613 ) ) ;
#26657=CARTESIAN_POINT ( 'NONE',  ( -9.984503880673420539, 203.7031108863293980, 68.34886208192143897 ) ) ;
#26658=CARTESIAN_POINT ( 'NONE',  ( -3.662846001189865142, 195.5725841191952838, 1.898862081921434131 ) ) ;
#26660=CARTESIAN_POINT ( 'NONE',  ( 8.118202686958039038, 212.8392687619912635, 25.70113791807856529 ) ) ;
#26663=CARTESIAN_POINT ( 'NONE',  ( -6.220909254589682469, 215.4770327129946850, 74.94886208192143329 ) ) ;
#26665=CARTESIAN_POINT ( 'NONE',  ( -8.118202686958039038, 201.1607312380087080, 96.20113791807857240 ) ) ;
#26668=CARTESIAN_POINT ( 'NONE',  ( -8.000000000000008882, 206.9523078486584780, 59.49886208192144466 ) ) ;
#26676=CARTESIAN_POINT ( 'NONE',  ( 4.984841277089725686, 213.7757310962907411, 73.55113791807856671 ) ) ;
#26681=CARTESIAN_POINT ( 'NONE',  ( -7.984503880673422316, 204.3529502787951628, 41.34886208192143897 ) ) ;
#26682=CARTESIAN_POINT ( 'NONE',  ( -3.135527875058821579, 197.5041725223112223, 80.90113791807858945 ) ) ;
#26684=CARTESIAN_POINT ( 'NONE',  ( 9.984503880673470277, 203.7031108863295401, 62.15113791807856813 ) ) ;
#26686=CARTESIAN_POINT ( 'NONE',  ( -0.05014649552807731031, 198.5883022060938572, 20.75113791807856600 ) ) ;
#26690=CARTESIAN_POINT ( 'NONE',  ( 9.736236675707914401, 214.0148392665762458, 46.70113791807857240 ) ) ;
#26692=CARTESIAN_POINT ( 'NONE',  ( 3.135527875058820690, 216.4958274776887492, 91.40113791807857524 ) ) ;
#26693=CARTESIAN_POINT ( 'NONE',  ( -8.118202686958039038, 201.1607312380087080, 69.20113791807858661 ) ) ;
#26694=CARTESIAN_POINT ( 'NONE',  ( 11.98450388067341876, 210.9467285061363953, 33.84886208192142476 ) ) ;
#26695=CARTESIAN_POINT ( 'NONE',  ( -3.135527875058982783, 216.4958274776886924, 39.09886208192143187 ) ) ;
#26697=CARTESIAN_POINT ( 'NONE',  ( -0.05014649552807705357, 194.3824533091408000, 77.75113791807856956 ) ) ;
#26698=CARTESIAN_POINT ( 'NONE',  ( -4.903702542908602524, 213.8346818373418898, 84.95113791807858661 ) ) ;
#26699=CARTESIAN_POINT ( 'NONE',  ( -3.135527875058982783, 216.4958274776886924, 51.09886208192143897 ) ) ;
#26703=CARTESIAN_POINT ( 'NONE',  ( 7.375838497908012492, 217.2372850707501186, 57.54886208192142760 ) ) ;
#26706=CARTESIAN_POINT ( 'NONE',  ( 8.015496119326595448, 204.4483345814782638, 37.14886208192143613 ) ) ;
#26711=CARTESIAN_POINT ( 'NONE',  ( -6.444103211791042618, 211.7408657792732356, 48.80113791807858092 ) ) ;
#26713=CARTESIAN_POINT ( 'NONE',  ( -3.135527875058982783, 216.4958274776886924, 33.09886208192143187 ) ) ;
#26715=ORIENTED_EDGE ( 'NONE', *, *, #29583, .F. ) ;
#26719=CARTESIAN_POINT ( 'NONE',  ( -7.984503880673422316, 204.3529502787951628, 14.34886208192143364 ) ) ;
#26720=CARTESIAN_POINT ( 'NONE',  ( 0.05014649552810505201, 217.5146222423826714, 49.25113791807857666 ) ) ;
#26722=CARTESIAN_POINT ( 'NONE',  ( -6.220909254589537696, 198.5229672870051161, 36.05113791807857382 ) ) ;
#26727=CARTESIAN_POINT ( 'NONE',  ( 4.984841277089891776, 200.2242689037093726, 100.4488620819214475 ) ) ;
#26730=DIRECTION ( 'NONE',  ( -0.1461455375466716444, 0.9854922318508084755, -0.08629335326029916042 ) ) ;
#26731=CARTESIAN_POINT ( 'NONE',  ( 7.375838497908181246, 196.7627149292499666, 20.45113791807856529 ) ) ;
#26732=CARTESIAN_POINT ( 'NONE',  ( -9.996365641501871124, 207.8097375604742467, 102.5363179372327096 ) ) ;
#26734=CARTESIAN_POINT ( 'NONE',  ( -3.044812012440131443, 216.5253028482142952, 64.10113791807857808 ) ) ;
#26735=CARTESIAN_POINT ( 'NONE',  ( -8.062137200540920645, 212.9164362838581894, 36.80113791807856671 ) ) ;
#26738=CARTESIAN_POINT ( 'NONE',  ( -8.118202686958138514, 212.8392687619910930, 8.798862081921434708 ) ) ;
#26741=CARTESIAN_POINT ( 'NONE',  ( 12.00000000000000711, 206.9523078486586485, 50.00113791807856956 ) ) ;
#26743=CARTESIAN_POINT ( 'NONE',  ( -10.01549611932659722, 210.2015048109875011, 17.64886208192143613 ) ) ;
#26746=CARTESIAN_POINT ( 'NONE',  ( -8.118202686958039038, 201.1607312380087080, 84.20113791807858661 ) ) ;
#26752=CARTESIAN_POINT ( 'NONE',  ( 2.517493886308900919, 214.5937144450984420, 25.40113791807857169 ) ) ;
#26754=CARTESIAN_POINT ( 'NONE',  ( -0.05014649552828403384, 217.5146222423826714, 3.248862081921433997 ) ) ;
#26762=CARTESIAN_POINT ( 'NONE',  ( -3.135527875058982783, 216.4958274776886924, 87.09886208192143897 ) ) ;
#26764=CARTESIAN_POINT ( 'NONE',  ( -8.062137200540920645, 212.9164362838581894, 18.80113791807856671 ) ) ;
#26765=CARTESIAN_POINT ( 'NONE',  ( -0.05014649552828442242, 219.6175466908591716, 81.24886208192143044 ) ) ;
#26769=CARTESIAN_POINT ( 'NONE',  ( -0.05014649552810635652, 196.4853777576173002, 98.75113791807854113 ) ) ;
#26772=CARTESIAN_POINT ( 'NONE',  ( 8.118202686958039038, 212.8392687619912635, 40.70113791807857240 ) ) ;
#26778=CARTESIAN_POINT ( 'NONE',  ( 3.662846001190051659, 195.5725841191953691, 20.60113791807856742 ) ) ;
#26782=CARTESIAN_POINT ( 'NONE',  ( -6.139770520408224463, 198.4640165459539105, 92.04886208192142760 ) ) ;
#26784=CARTESIAN_POINT ( 'NONE',  ( 3.753561863808876797, 195.6020594897209719, 37.59886208192143187 ) ) ;
#26786=CARTESIAN_POINT ( 'NONE',  ( 0.05014649552810505201, 217.5146222423826714, 52.25113791807856245 ) ) ;
#26789=CARTESIAN_POINT ( 'NONE',  ( -2.517493886309087880, 214.5937144450984135, 15.09886208192143719 ) ) ;
#26794=CARTESIAN_POINT ( 'NONE',  ( -0.05014649552828365914, 215.4116977939061144, 99.24886208192143044 ) ) ;
#26796=CARTESIAN_POINT ( 'NONE',  ( 8.000000000000008882, 206.9523078486586485, 41.00113791807857666 ) ) ;
#26801=CARTESIAN_POINT ( 'NONE',  ( -8.062137200540822946, 201.0835637161416400, 56.19886208192144039 ) ) ;
#26804=CARTESIAN_POINT ( 'NONE',  ( -6.444103211791042618, 211.7408657792732356, 93.80113791807858092 ) ) ;
#26808=CARTESIAN_POINT ( 'NONE',  ( -0.05014649552828365914, 215.4116977939061144, 69.24886208192143044 ) ) ;
#26814=CARTESIAN_POINT ( 'NONE',  ( -6.139770520408368348, 215.5359834540460042, 9.951137918078567068 ) ) ;
#26818=CARTESIAN_POINT ( 'NONE',  ( -0.05014649552807705357, 194.3824533091408000, 80.75113791807856956 ) ) ;
#26820=CARTESIAN_POINT ( 'NONE',  ( 8.118202686958039038, 212.8392687619912635, 100.7011379180785866 ) ) ;
#26823=CARTESIAN_POINT ( 'NONE',  ( -12.10169002831357510, 232.5389149829038331, 105.4832055762867782 ) ) ;
#26824=CARTESIAN_POINT ( 'NONE',  ( -7.375838497908014268, 196.7627149292498530, 65.04886208192144181 ) ) ;
#26826=CARTESIAN_POINT ( 'NONE',  ( 10.00000000000000711, 207.0476921513415220, 63.99886208192143044 ) ) ;
#26827=CARTESIAN_POINT ( 'NONE',  ( -7.375838497908014268, 196.7627149292498530, 5.048862081921433820 ) ) ;
#26829=CARTESIAN_POINT ( 'NONE',  ( -0.05014649552810635652, 196.4853777576173002, 26.75113791807856956 ) ) ;
#26830=CARTESIAN_POINT ( 'NONE',  ( 0.05014649552828275708, 196.4853777576173002, 91.74886208192144466 ) ) ;
#26836=CARTESIAN_POINT ( 'NONE',  ( 6.444103211790928043, 211.7408657792734061, 66.69886208192143329 ) ) ;
#26844=CARTESIAN_POINT ( 'NONE',  ( 4.903702542908601636, 200.1653181626581102, 68.45113791807857240 ) ) ;
#26850=CARTESIAN_POINT ( 'NONE',  ( 2.517493886309087436, 199.4062855549015865, 46.59886208192143897 ) ) ;
#26851=CARTESIAN_POINT ( 'NONE',  ( 10.01549611932653860, 210.2015048109876716, 82.85113791807854966 ) ) ;
#26853=CARTESIAN_POINT ( 'NONE',  ( 3.044812012440130555, 197.4746971517856764, 62.60113791807857098 ) ) ;
#26855=CARTESIAN_POINT ( 'NONE',  ( 2.426778023690261410, 199.3768101843759837, 23.60113791807857098 ) ) ;
#26861=CARTESIAN_POINT ( 'NONE',  ( 9.680171189290831535, 199.9079932115568852, 50.30113791807857382 ) ) ;
#26865=CARTESIAN_POINT ( 'NONE',  ( 3.135527875058820690, 216.4958274776887492, 97.40113791807858945 ) ) ;
#26866=CARTESIAN_POINT ( 'NONE',  ( -6.139770520408368348, 215.5359834540460042, 66.95113791807857240 ) ) ;
#26867=CARTESIAN_POINT ( 'NONE',  ( -7.456977232089471386, 217.1783343296987709, 35.94886208192142618 ) ) ;
#26868=CARTESIAN_POINT ( 'NONE',  ( -6.139770520408224463, 198.4640165459539105, 35.04886208192143471 ) ) ;
#26870=CARTESIAN_POINT ( 'NONE',  ( -12.00000000000000711, 207.0476921513413515, 81.50113791807856956 ) ) ;
#26871=CARTESIAN_POINT ( 'NONE',  ( -4.903702542908602524, 213.8346818373418898, 99.95113791807860082 ) ) ;
#26872=CARTESIAN_POINT ( 'NONE',  ( 8.118202686958138514, 201.1607312380088501, 58.29886208192143471 ) ) ;
#26875=CARTESIAN_POINT ( 'NONE',  ( -12.01549611932659722, 210.8513442034533227, 59.64886208192143613 ) ) ;
#26877=CARTESIAN_POINT ( 'NONE',  ( -2.426778023690076225, 199.3768101843759553, 31.89886208192144323 ) ) ;
#26884=CARTESIAN_POINT ( 'NONE',  ( 6.500168698208129925, 211.6636982574063381, 49.70113791807857240 ) ) ;
#26887=CARTESIAN_POINT ( 'NONE',  ( 9.984503880673420539, 210.2968891136705167, 36.84886208192143187 ) ) ;
#26894=CARTESIAN_POINT ( 'NONE',  ( 8.015496119326595448, 204.4483345814782638, 19.14886208192143968 ) ) ;
#26895=CARTESIAN_POINT ( 'NONE',  ( 6.139770520408368348, 198.4640165459539674, 53.45113791807855108 ) ) ;
#26897=CARTESIAN_POINT ( 'NONE',  ( 6.220909254589536808, 215.4770327129947702, 34.55113791807855250 ) ) ;
#26901=CARTESIAN_POINT ( 'NONE',  ( 2.426778023690075337, 214.6231898156240447, 99.39886208192146455 ) ) ;
#26905=CARTESIAN_POINT ( 'NONE',  ( -3.662846001190052991, 218.4274158808045740, 16.10113791807856742 ) ) ;
#26908=CARTESIAN_POINT ( 'NONE',  ( -10.01549611932653860, 203.7984951890123284, 66.35113791807853545 ) ) ;
#26909=CARTESIAN_POINT ( 'NONE',  ( 8.118202686958039038, 212.8392687619912635, 40.70113791807857240 ) ) ;
#26912=CARTESIAN_POINT ( 'NONE',  ( -12.01549611932652972, 203.1486557965464499, 102.3511379180785639 ) ) ;
#26913=CARTESIAN_POINT ( 'NONE',  ( 3.135527875058981895, 197.5041725223112792, 10.59886208192143542 ) ) ;
#26916=CARTESIAN_POINT ( 'NONE',  ( 7.375838497908181246, 196.7627149292499666, 44.45113791807857240 ) ) ;
#26917=CARTESIAN_POINT ( 'NONE',  ( 8.015496119326531499, 209.5516654185219636, 64.85113791807857808 ) ) ;
#26919=CARTESIAN_POINT ( 'NONE',  ( 6.139770520408223575, 215.5359834540460611, 21.54886208192143826 ) ) ;
#26922=CARTESIAN_POINT ( 'NONE',  ( 3.135527875058820690, 216.4958274776887492, 76.40113791807857524 ) ) ;
#26927=CARTESIAN_POINT ( 'NONE',  ( -7.984503880673488041, 209.6470497212046098, 21.65113791807856813 ) ) ;
#26929=CARTESIAN_POINT ( 'NONE',  ( 8.118202686958138514, 201.1607312380088501, 7.298862081921435596 ) ) ;
#26936=CARTESIAN_POINT ( 'NONE',  ( -6.220909254589682469, 215.4770327129946850, 89.94886208192140487 ) ) ;
#26938=CARTESIAN_POINT ( 'NONE',  ( -8.118202686958039038, 201.1607312380087080, 21.20113791807856529 ) ) ;
#26940=CARTESIAN_POINT ( 'NONE',  ( -3.753561863808878130, 218.3979405102790281, 78.09886208192142476 ) ) ;
#26944=CARTESIAN_POINT ( 'NONE',  ( 6.139770520408368348, 198.4640165459539674, 95.45113791807855819 ) ) ;
#26947=CARTESIAN_POINT ( 'NONE',  ( 10.00000000000000711, 206.9523078486586201, 38.00113791807857666 ) ) ;
#26953=CARTESIAN_POINT ( 'NONE',  ( 3.753561863808689836, 218.3979405102790565, 19.40113791807856813 ) ) ;
#26957=CARTESIAN_POINT ( 'NONE',  ( -11.98450388067341876, 203.0532714938636047, 32.34886208192142476 ) ) ;
#26959=CARTESIAN_POINT ( 'NONE',  ( -6.220909254589537696, 198.5229672870051161, 54.05113791807856671 ) ) ;
#26961=CARTESIAN_POINT ( 'NONE',  ( -0.05014649552828365914, 215.4116977939061144, 15.24886208192143577 ) ) ;
#26964=CARTESIAN_POINT ( 'NONE',  ( 8.015496119326595448, 204.4483345814782638, 100.1488620819214646 ) ) ;
#26965=CARTESIAN_POINT ( 'NONE',  ( -2.517493886308901807, 199.4062855549015012, 35.90113791807856813 ) ) ;
#26969=CARTESIAN_POINT ( 'NONE',  ( 3.044812012439969795, 216.5253028482143520, 60.39886208192143613 ) ) ;
#26972=CARTESIAN_POINT ( 'NONE',  ( -0.05014649552807731031, 198.5883022060938572, 101.7511379180785696 ) ) ;
#26974=CARTESIAN_POINT ( 'NONE',  ( 4.903702542908435547, 213.8346818373419751, 75.54886208192142760 ) ) ;
#26979=CARTESIAN_POINT ( 'NONE',  ( -6.220909254589537696, 198.5229672870051445, 15.05113791807856494 ) ) ;
#26984=CARTESIAN_POINT ( 'NONE',  ( -3.662846001190052991, 218.4274158808045740, 79.10113791807857808 ) ) ;
#26986=CARTESIAN_POINT ( 'NONE',  ( -10.00000000000000711, 207.0476921513413515, 96.50113791807856956 ) ) ;
#26991=CARTESIAN_POINT ( 'NONE',  ( 8.062137200540822946, 212.9164362838583315, 6.698862081921435063 ) ) ;
#26992=CARTESIAN_POINT ( 'NONE',  ( 3.662846001189864698, 218.4274158808046593, 57.39886208192143613 ) ) ;
#26994=CARTESIAN_POINT ( 'NONE',  ( 9.984503880673420539, 210.2968891136705736, 66.84886208192142476 ) ) ;
#26995=CARTESIAN_POINT ( 'NONE',  ( 12.01549611932659367, 203.1486557965466773, 1.148862081921433909 ) ) ;
#26997=CARTESIAN_POINT ( 'NONE',  ( 10.00000000000000711, 206.9523078486586201, 23.00113791807856600 ) ) ;
#26998=CARTESIAN_POINT ( 'NONE',  ( 3.044812012439969795, 216.5253028482143520, 87.39886208192143613 ) ) ;
#27004=CARTESIAN_POINT ( 'NONE',  ( -7.984503880673422316, 204.3529502787951628, 68.34886208192142476 ) ) ;
#27012=CARTESIAN_POINT ( 'NONE',  ( -2.426778023690262742, 214.6231898156240163, 70.10113791807857808 ) ) ;
#27013=DIRECTION ( 'NONE',  ( 0.000000000000000000, 0.04769215134145521340, 0.9988620819214352187 ) ) ;
#27017=CARTESIAN_POINT ( 'NONE',  ( -0.05014649552828365914, 215.4116977939061144, 45.24886208192144466 ) ) ;
#27018=CARTESIAN_POINT ( 'NONE',  ( 8.062137200540920645, 201.0835637161417822, 89.30113791807858092 ) ) ;
#27019=CARTESIAN_POINT ( 'NONE',  ( -6.220909254589537696, 198.5229672870051161, 69.05113791807858092 ) ) ;
#27023=CARTESIAN_POINT ( 'NONE',  ( -7.984503880673488041, 209.6470497212046098, 21.65113791807856813 ) ) ;
#27027=CARTESIAN_POINT ( 'NONE',  ( -7.375838497908182134, 217.2372850707499765, 48.95113791807855108 ) ) ;
#27029=CARTESIAN_POINT ( 'NONE',  ( -6.139770520408369237, 215.5359834540460042, 90.95113791807854398 ) ) ;
#27030=CARTESIAN_POINT ( 'NONE',  ( 6.139770520408367460, 198.4640165459539389, 71.45113791807857240 ) ) ;
#27031=CARTESIAN_POINT ( 'NONE',  ( 11.98450388067341876, 210.9467285061363953, 36.84886208192142476 ) ) ;
#27032=CARTESIAN_POINT ( 'NONE',  ( -9.984503880673420539, 203.7031108863293980, 41.34886208192143187 ) ) ;
#27034=CARTESIAN_POINT ( 'NONE',  ( 3.662846001190051659, 195.5725841191953691, 80.60113791807857808 ) ) ;
#27036=CARTESIAN_POINT ( 'NONE',  ( -8.000000000000008882, 207.0476921513413515, 93.50113791807858377 ) ) ;
#27038=CARTESIAN_POINT ( 'NONE',  ( -10.00000000000000711, 206.9523078486584495, 59.49886208192143755 ) ) ;
#27040=ORIENTED_EDGE ( 'NONE', *, *, #5398, .F. ) ;
#27041=CARTESIAN_POINT ( 'NONE',  ( 3.662846001189864698, 218.4274158808046593, 60.39886208192143613 ) ) ;
#27045=CARTESIAN_POINT ( 'NONE',  ( -6.444103211790928043, 202.2591342207265939, 41.19886208192144750 ) ) ;
#27052=CARTESIAN_POINT ( 'NONE',  ( 0.05014649552807626948, 215.4116977939061144, 52.25113791807857666 ) ) ;
#27054=CARTESIAN_POINT ( 'NONE',  ( 10.00000000000000711, 207.0476921513415220, 36.99886208192143755 ) ) ;
#27060=CARTESIAN_POINT ( 'NONE',  ( -2.426778023690076225, 199.3768101843759553, 16.89886208192143613 ) ) ;
#27062=CARTESIAN_POINT ( 'NONE',  ( 10.01549611932653860, 210.2015048109876716, 61.85113791807857098 ) ) ;
#27063=CARTESIAN_POINT ( 'NONE',  ( -10.01549611932653860, 203.7984951890123284, 33.35113791807855677 ) ) ;
#27067=CARTESIAN_POINT ( 'NONE',  ( 6.444103211791042618, 202.2591342207267644, -0.6988620819214341751 ) ) ;
#27071=CARTESIAN_POINT ( 'NONE',  ( 9.680171189290831535, 199.9079932115568852, 23.30113791807857027 ) ) ;
#27073=CARTESIAN_POINT ( 'NONE',  ( -8.062137200540920645, 212.9164362838581894, 63.80113791807858092 ) ) ;
#27074=CARTESIAN_POINT ( 'NONE',  ( 10.01549611932653860, 210.2015048109876716, 43.85113791807856387 ) ) ;
#27076=DIRECTION ( 'NONE',  ( -0.3500148194780949296, -0.04467534437043436946, 0.9356782244720136532 ) ) ;
#27078=CARTESIAN_POINT ( 'NONE',  ( 12.00000000000000711, 207.0476921513415220, 6.998862081921433997 ) ) ;
#27079=CARTESIAN_POINT ( 'NONE',  ( -0.05014649552828402690, 217.5146222423826714, 9.248862081921433997 ) ) ;
#27081=ORIENTED_EDGE ( 'NONE', *, *, #32237, .T. ) ;
#27082=CARTESIAN_POINT ( 'NONE',  ( 7.375838497908181246, 196.7627149292499666, 47.45113791807857950 ) ) ;
#27083=CARTESIAN_POINT ( 'NONE',  ( -6.444103211791042618, 211.7408657792732356, 69.80113791807856671 ) ) ;
#27086=CARTESIAN_POINT ( 'NONE',  ( -3.044812012439970683, 197.4746971517856196, 34.89886208192143613 ) ) ;
#27090=CARTESIAN_POINT ( 'NONE',  ( -6.220909254589537696, 198.5229672870051161, 81.05113791807856671 ) ) ;
#27099=CARTESIAN_POINT ( 'NONE',  ( 8.015496119326531499, 209.5516654185219636, 25.85113791807856742 ) ) ;
#27101=CARTESIAN_POINT ( 'NONE',  ( -8.118202686958138514, 212.8392687619910930, 8.798862081921434708 ) ) ;
#27106=CARTESIAN_POINT ( 'NONE',  ( -2.426778023690262742, 214.6231898156240163, 52.10113791807857808 ) ) ;
#27110=CARTESIAN_POINT ( 'NONE',  ( -8.062137200540822946, 201.0835637161416400, 92.19886208192143329 ) ) ;
#27112=CARTESIAN_POINT ( 'NONE',  ( -6.220909254589537696, 198.5229672870051161, 21.05113791807855961 ) ) ;
#27114=CARTESIAN_POINT ( 'NONE',  ( -7.375838497908014268, 196.7627149292498530, 77.04886208192142760 ) ) ;
#27118=CARTESIAN_POINT ( 'NONE',  ( 6.220909254589536808, 215.4770327129947702, 97.55113791807855250 ) ) ;
#27122=CARTESIAN_POINT ( 'NONE',  ( -0.05014649552810635652, 196.4853777576173002, 41.75113791807855534 ) ) ;
#27128=CARTESIAN_POINT ( 'NONE',  ( -11.98450388067348804, 210.9467285061362247, 18.65113791807856458 ) ) ;
#27132=CARTESIAN_POINT ( 'NONE',  ( -12.00000000000000711, 206.9523078486584780, 38.49886208192143044 ) ) ;
#27134=CARTESIAN_POINT ( 'NONE',  ( -8.062137200540920645, 212.9164362838581894, 51.80113791807857382 ) ) ;
#27136=CARTESIAN_POINT ( 'NONE',  ( 2.426778023690075337, 214.6231898156240447, 9.398862081921436129 ) ) ;
#27140=CARTESIAN_POINT ( 'NONE',  ( -6.444103211790928043, 202.2591342207265939, 104.1988620819214475 ) ) ;
#27143=CARTESIAN_POINT ( 'NONE',  ( 4.984841277089725686, 213.7757310962907411, 40.55113791807856671 ) ) ;
#27149=CARTESIAN_POINT ( 'NONE',  ( 6.220909254589681581, 198.5229672870052582, 64.44886208192143329 ) ) ;
#27152=CARTESIAN_POINT ( 'NONE',  ( 6.500168698208129925, 211.6636982574063381, 97.70113791807858661 ) ) ;
#27156=CARTESIAN_POINT ( 'NONE',  ( -8.000000000000008882, 206.9523078486584780, 77.49886208192144466 ) ) ;
#27160=CARTESIAN_POINT ( 'NONE',  ( -6.139770520408368348, 215.5359834540460042, 21.95113791807856529 ) ) ;
#27164=CARTESIAN_POINT ( 'NONE',  ( 7.456977232089302632, 217.1783343296989131, 91.55113791807858092 ) ) ;
#27166=CARTESIAN_POINT ( 'NONE',  ( 3.044812012440130555, 197.4746971517856764, 92.60113791807857808 ) ) ;
#27169=CARTESIAN_POINT ( 'NONE',  ( 3.044812012439969795, 216.5253028482143520, 6.398862081921435241 ) ) ;
#27170=CARTESIAN_POINT ( 'NONE',  ( 7.456977232089471386, 196.8216656703012006, 61.44886208192143329 ) ) ;
#27171=CARTESIAN_POINT ( 'NONE',  ( -0.05014649552828402690, 217.5146222423826714, 78.24886208192144466 ) ) ;
#27172=CARTESIAN_POINT ( 'NONE',  ( -11.98450388067341876, 203.0532714938636047, 5.348862081921434530 ) ) ;
#27174=CARTESIAN_POINT ( 'NONE',  ( 8.062137200540920645, 201.0835637161417822, 23.30113791807856671 ) ) ;
#27175=CARTESIAN_POINT ( 'NONE',  ( -8.118202686958138514, 212.8392687619910930, 86.79886208192142760 ) ) ;
#27180=CARTESIAN_POINT ( 'NONE',  ( 6.500168698208244500, 202.3363017425938324, 70.29886208192142760 ) ) ;
#27188=CARTESIAN_POINT ( 'NONE',  ( 6.444103211791042618, 202.2591342207267644, 71.30113791807856671 ) ) ;
#27191=CARTESIAN_POINT ( 'NONE',  ( -4.984841277089891776, 213.7757310962905990, 47.94886208192144039 ) ) ;
#27192=CARTESIAN_POINT ( 'NONE',  ( 10.01549611932653860, 210.2015048109876716, 91.85113791807853545 ) ) ;
#27193=CARTESIAN_POINT ( 'NONE',  ( 8.062137200540920645, 201.0835637161417822, 80.30113791807858092 ) ) ;
#27198=CARTESIAN_POINT ( 'NONE',  ( -9.736236675707914401, 199.9851607334237542, 51.20113791807856529 ) ) ;
#27200=CARTESIAN_POINT ( 'NONE',  ( -3.135527875058821579, 197.5041725223112223, 101.9011379180785752 ) ) ;
#27201=CARTESIAN_POINT ( 'NONE',  ( 0.05014649552810506589, 217.5146222423826714, 70.25113791807856956 ) ) ;
#27202=CARTESIAN_POINT ( 'NONE',  ( 9.736236675708031640, 199.9851607334238963, 31.29886208192143826 ) ) ;
#27203=CARTESIAN_POINT ( 'NONE',  ( 9.984503880673420539, 210.2968891136705736, 45.84886208192142476 ) ) ;
#27205=CARTESIAN_POINT ( 'NONE',  ( -11.98450388067348804, 210.9467285061362247, 78.65113791807858945 ) ) ;
#27206=CARTESIAN_POINT ( 'NONE',  ( 4.903702542908601636, 200.1653181626581102, 101.4511379180785866 ) ) ;
#27209=CARTESIAN_POINT ( 'NONE',  ( 10.01549611932659545, 203.7984951890123853, 64.14886208192145034 ) ) ;
#27212=CARTESIAN_POINT ( 'NONE',  ( 9.680171189290716072, 214.0920067884432854, 63.69886208192144039 ) ) ;
#27215=CARTESIAN_POINT ( 'NONE',  ( -2.517493886309087880, 214.5937144450984135, 42.09886208192144608 ) ) ;
#27221=CARTESIAN_POINT ( 'NONE',  ( -2.426778023690262742, 214.6231898156240163, 55.10113791807857808 ) ) ;
#27223=CARTESIAN_POINT ( 'NONE',  ( -3.044812012439970683, 197.4746971517856196, 34.89886208192143613 ) ) ;
#27230=CARTESIAN_POINT ( 'NONE',  ( -6.444103211790928043, 202.2591342207265939, 11.19886208192143506 ) ) ;
#27231=CARTESIAN_POINT ( 'NONE',  ( -8.062137200540920645, 212.9164362838581894, 60.80113791807857382 ) ) ;
#27232=CARTESIAN_POINT ( 'NONE',  ( 8.062137200540920645, 201.0835637161417822, 38.30113791807857382 ) ) ;
#27234=CARTESIAN_POINT ( 'NONE',  ( -7.984503880673488041, 209.6470497212046098, 0.6511379180785660248 ) ) ;
#27238=CARTESIAN_POINT ( 'NONE',  ( -9.680171189290831535, 214.0920067884431148, 15.80113791807856849 ) ) ;
#27241=CARTESIAN_POINT ( 'NONE',  ( 6.139770520408368348, 198.4640165459539674, 62.45113791807857950 ) ) ;
#27242=CARTESIAN_POINT ( 'NONE',  ( 6.220909254589536808, 215.4770327129947987, 43.55113791807857382 ) ) ;
#27245=CARTESIAN_POINT ( 'NONE',  ( -9.736236675708031640, 214.0148392665760753, 2.798862081921433820 ) ) ;
#27246=CARTESIAN_POINT ( 'NONE',  ( -3.135527875058982783, 216.4958274776886924, 9.098862081921435419 ) ) ;
#27249=CARTESIAN_POINT ( 'NONE',  ( -12.00000000000000711, 207.0476921513413515, 45.50113791807856956 ) ) ;
#27250=CARTESIAN_POINT ( 'NONE',  ( 8.000000000000008882, 206.9523078486586485, 65.00113791807856956 ) ) ;
#27252=CARTESIAN_POINT ( 'NONE',  ( 9.984503880673420539, 210.2968891136705167, 33.84886208192143187 ) ) ;
#27255=CARTESIAN_POINT ( 'NONE',  ( -8.118202686958039038, 201.1607312380087080, 87.20113791807858661 ) ) ;
#27261=CARTESIAN_POINT ( 'NONE',  ( -0.05014649552807731031, 198.5883022060938572, 23.75113791807855890 ) ) ;
#27263=CARTESIAN_POINT ( 'NONE',  ( -11.98450388067341876, 203.0532714938636047, 104.3488620819214532 ) ) ;
#27266=CARTESIAN_POINT ( 'NONE',  ( -6.444103211791042618, 211.7408657792732356, 51.80113791807858092 ) ) ;
#27271=CARTESIAN_POINT ( 'NONE',  ( -3.044812012439970683, 197.4746971517856196, 94.89886208192143613 ) ) ;
#27273=CARTESIAN_POINT ( 'NONE',  ( -6.220909254589537696, 198.5229672870051161, 33.05113791807857382 ) ) ;
#27276=ADVANCED_FACE ( 'NONE', ( #18812 ), #12364, .T. ) ;
#27277=CARTESIAN_POINT ( 'NONE',  ( -12.01549611932659722, 210.8513442034533227, 74.64886208192143613 ) ) ;
#27281=CARTESIAN_POINT ( 'NONE',  ( -8.118202686958039038, 201.1607312380087080, 99.20113791807858661 ) ) ;
#27286=CARTESIAN_POINT ( 'NONE',  ( -9.984503880673473830, 210.2968891136704315, 36.65113791807855392 ) ) ;
#27291=CARTESIAN_POINT ( 'NONE',  ( -0.05014649552807705357, 194.3824533091408000, 23.75113791807855890 ) ) ;
#27294=CARTESIAN_POINT ( 'NONE',  ( -9.521242624480144912, 207.9188892840786878, 102.6634595774070533 ) ) ;
#27297=CARTESIAN_POINT ( 'NONE',  ( 0.05014649552828288198, 194.3824533091408000, 40.74886208192143044 ) ) ;
#27298=CARTESIAN_POINT ( 'NONE',  ( -3.135527875058821579, 197.5041725223112223, 5.901137918078566358 ) ) ;
#27299=CARTESIAN_POINT ( 'NONE',  ( 3.044812012440130555, 197.4746971517856764, 53.60113791807857098 ) ) ;
#27300=CARTESIAN_POINT ( 'NONE',  ( 4.984841277089891776, 200.2242689037093726, 16.44886208192143684 ) ) ;
#27303=CARTESIAN_POINT ( 'NONE',  ( -8.000000000000008882, 206.9523078486584780, 104.4988620819214304 ) ) ;
#27305=CARTESIAN_POINT ( 'NONE',  ( -6.500168698208129925, 202.3363017425936050, 36.20113791807857240 ) ) ;
#27309=DIRECTION ( 'NONE',  ( 0.000000000000000000, -0.04769215134144196705, 0.9988620819214357738 ) ) ;
#27310=CARTESIAN_POINT ( 'NONE',  ( -10.01549611932659722, 210.2015048109875011, 65.64886208192143613 ) ) ;
#27313=CARTESIAN_POINT ( 'NONE',  ( -3.135527875058821579, 197.5041725223112223, 5.901137918078566358 ) ) ;
#27317=CARTESIAN_POINT ( 'NONE',  ( 4.903702542908435547, 213.8346818373419751, 81.54886208192144181 ) ) ;
#27321=CARTESIAN_POINT ( 'NONE',  ( -3.044812012440131443, 216.5253028482142952, 22.10113791807856742 ) ) ;
#27326=CARTESIAN_POINT ( 'NONE',  ( 3.662846001190051659, 195.5725841191953691, 83.60113791807857808 ) ) ;
#27331=CARTESIAN_POINT ( 'NONE',  ( -0.05014649552828442242, 219.6175466908591716, 69.24886208192143044 ) ) ;
#27332=CARTESIAN_POINT ( 'NONE',  ( -10.00000000000000711, 206.9523078486584495, 77.49886208192144466 ) ) ;
#27333=CARTESIAN_POINT ( 'NONE',  ( -11.98450388067341876, 203.0532714938636047, 17.34886208192143187 ) ) ;
#27335=CARTESIAN_POINT ( 'NONE',  ( -6.220909254589537696, 198.5229672870051161, 24.05113791807855961 ) ) ;
#27336=CARTESIAN_POINT ( 'NONE',  ( 3.044812012439969795, 216.5253028482143520, 93.39886208192143613 ) ) ;
#27341=CARTESIAN_POINT ( 'NONE',  ( 7.984503880673422316, 209.6470497212048372, 75.84886208192143897 ) ) ;
#27350=CARTESIAN_POINT ( 'NONE',  ( -6.500168698208129925, 202.3363017425936050, 66.20113791807857240 ) ) ;
#27354=CARTESIAN_POINT ( 'NONE',  ( 2.517493886309087436, 199.4062855549015865, 52.59886208192143897 ) ) ;
#27355=CARTESIAN_POINT ( 'NONE',  ( 8.118202686958039038, 212.8392687619912635, 76.70113791807857240 ) ) ;
#27361=CARTESIAN_POINT ( 'NONE',  ( -9.680171189290831535, 214.0920067884431148, 57.80113791807857382 ) ) ;
#27363=CARTESIAN_POINT ( 'NONE',  ( 9.984503880673470277, 203.7031108863295401, 101.1511379180785752 ) ) ;
#27365=CARTESIAN_POINT ( 'NONE',  ( -6.220909254589537696, 198.5229672870051445, 78.05113791807858092 ) ) ;
#27366=CARTESIAN_POINT ( 'NONE',  ( 9.736236675708031640, 199.9851607334238963, 43.29886208192143471 ) ) ;
#27367=CARTESIAN_POINT ( 'NONE',  ( 8.118202686958138514, 201.1607312380088501, 52.29886208192143471 ) ) ;
#27369=CARTESIAN_POINT ( 'NONE',  ( 11.98450388067348271, 203.0532714938637753, 89.15113791807856103 ) ) ;
#27370=CARTESIAN_POINT ( 'NONE',  ( 8.000000000000008882, 206.9523078486586485, 101.0011379180785696 ) ) ;
#27371=CARTESIAN_POINT ( 'NONE',  ( 3.135527875058981895, 197.5041725223112792, 61.59886208192143897 ) ) ;
#27375=CARTESIAN_POINT ( 'NONE',  ( 7.375838497908012492, 217.2372850707501186, 60.54886208192144181 ) ) ;
#27378=CARTESIAN_POINT ( 'NONE',  ( 0.05014649552828262524, 198.5883022060938572, 37.74886208192143755 ) ) ;
#27384=CARTESIAN_POINT ( 'NONE',  ( -2.517493886308901807, 199.4062855549015012, 59.90113791807856813 ) ) ;
#27387=CARTESIAN_POINT ( 'NONE',  ( 0.05014649552828275708, 196.4853777576173002, 46.74886208192143755 ) ) ;
#27393=CARTESIAN_POINT ( 'NONE',  ( 6.500168698208244500, 202.3363017425938324, 19.29886208192143471 ) ) ;
#27395=CARTESIAN_POINT ( 'NONE',  ( -3.044812012440131443, 216.5253028482142952, 64.10113791807857808 ) ) ;
#27396=CARTESIAN_POINT ( 'NONE',  ( 10.01549611932653860, 210.2015048109876716, 43.85113791807854966 ) ) ;
#27400=CARTESIAN_POINT ( 'NONE',  ( 6.220909254589536808, 215.4770327129947702, 22.55113791807856671 ) ) ;
#27401=CARTESIAN_POINT ( 'NONE',  ( 4.903702542908435547, 213.8346818373419751, 99.54886208192144181 ) ) ;
#27405=CARTESIAN_POINT ( 'NONE',  ( 0.05014649552807549926, 219.6175466908591716, 25.25113791807856956 ) ) ;
#27408=CARTESIAN_POINT ( 'NONE',  ( -3.135527875058821579, 197.5041725223112223, 77.90113791807857524 ) ) ;
#27410=CARTESIAN_POINT ( 'NONE',  ( 10.00000000000000711, 206.9523078486586201, 35.00113791807856956 ) ) ;
#27413=CARTESIAN_POINT ( 'NONE',  ( -11.98450388067341876, 203.0532714938636047, 2.348862081921434530 ) ) ;
#27414=CARTESIAN_POINT ( 'NONE',  ( 8.118202686958138514, 201.1607312380088501, 16.29886208192143471 ) ) ;
#27417=CARTESIAN_POINT ( 'NONE',  ( 0.05014649552807549926, 219.6175466908591716, 52.25113791807857666 ) ) ;
#27418=CARTESIAN_POINT ( 'NONE',  ( -2.517493886308901807, 199.4062855549015012, 71.90113791807856103 ) ) ;
#27419=CARTESIAN_POINT ( 'NONE',  ( -6.139770520408224463, 198.4640165459539389, 35.04886208192144181 ) ) ;
#27424=CARTESIAN_POINT ( 'NONE',  ( 6.139770520408368348, 198.4640165459539674, 89.45113791807857240 ) ) ;
#27430=CARTESIAN_POINT ( 'NONE',  ( -7.984503880673488041, 209.6470497212046098, 36.65113791807856103 ) ) ;
#27433=CARTESIAN_POINT ( 'NONE',  ( -6.220909254589682469, 215.4770327129946850, 17.94886208192143684 ) ) ;
#27436=CARTESIAN_POINT ( 'NONE',  ( -6.500168698208129925, 202.3363017425936050, 48.20113791807858661 ) ) ;
#27441=CARTESIAN_POINT ( 'NONE',  ( 3.044812012439969795, 216.5253028482143520, 87.39886208192143613 ) ) ;
#27444=CARTESIAN_POINT ( 'NONE',  ( 6.220909254589536808, 215.4770327129947702, 28.55113791807855961 ) ) ;
#27446=CARTESIAN_POINT ( 'NONE',  ( 3.044812012440130555, 197.4746971517856764, 17.60113791807856742 ) ) ;
#27450=CARTESIAN_POINT ( 'NONE',  ( -6.139770520408369237, 215.5359834540460042, 90.95113791807854398 ) ) ;
#27453=CARTESIAN_POINT ( 'NONE',  ( -9.984503880673473830, 210.2968891136704315, 45.65113791807855392 ) ) ;
#27459=CARTESIAN_POINT ( 'NONE',  ( 3.753561863808689836, 218.3979405102790565, 16.40113791807856458 ) ) ;
#27463=CARTESIAN_POINT ( 'NONE',  ( 9.736236675708031640, 199.9851607334238963, 40.29886208192143471 ) ) ;
#27464=CARTESIAN_POINT ( 'NONE',  ( 0.05014649552810505201, 217.5146222423826714, 1.251137918078566003 ) ) ;
#27465=CARTESIAN_POINT ( 'NONE',  ( -9.984503880673473830, 210.2968891136704315, 57.65113791807858235 ) ) ;
#27466=CARTESIAN_POINT ( 'NONE',  ( -6.444103211790928043, 202.2591342207265939, 26.19886208192144039 ) ) ;
#27467=EDGE_CURVE ( 'NONE', #29176, #860, #26509, .T. ) ;
#27470=CARTESIAN_POINT ( 'NONE',  ( 8.000000000000008882, 207.0476921513415220, 99.99886208192143044 ) ) ;
#27473=CARTESIAN_POINT ( 'NONE',  ( -6.444103211791042618, 211.7408657792732356, 36.80113791807856671 ) ) ;
#27479=CARTESIAN_POINT ( 'NONE',  ( -9.984503880673420539, 203.7031108863293980, 59.34886208192141765 ) ) ;
#27483=CARTESIAN_POINT ( 'NONE',  ( -6.139770520408369237, 215.5359834540460042, 6.951137918078566180 ) ) ;
#27488=CARTESIAN_POINT ( 'NONE',  ( 0.05014649552828262524, 198.5883022060938572, 85.74886208192143044 ) ) ;
#27492=CARTESIAN_POINT ( 'NONE',  ( 3.135527875058820690, 216.4958274776887492, 19.40113791807856813 ) ) ;
#27496=CARTESIAN_POINT ( 'NONE',  ( -12.00000000000000711, 207.0476921513413515, 90.50113791807858377 ) ) ;
#27499=CARTESIAN_POINT ( 'NONE',  ( 9.680171189290716072, 214.0920067884432854, 72.69886208192143329 ) ) ;
#27500=CARTESIAN_POINT ( 'NONE',  ( -3.044812012439970683, 197.4746971517856196, 73.89886208192143613 ) ) ;
#27501=CARTESIAN_POINT ( 'NONE',  ( 3.753561863808876797, 195.6020594897209719, 13.59886208192143719 ) ) ;
#27503=CARTESIAN_POINT ( 'NONE',  ( -6.220909254589537696, 198.5229672870051161, 30.05113791807856671 ) ) ;
#27505=CARTESIAN_POINT ( 'NONE',  ( 8.062137200540822946, 212.9164362838583315, 84.69886208192144750 ) ) ;
#27510=CARTESIAN_POINT ( 'NONE',  ( -4.984841277089891776, 213.7757310962905990, 68.94886208192144750 ) ) ;
#27519=CARTESIAN_POINT ( 'NONE',  ( 8.000000000000008882, 206.9523078486586485, 80.00113791807856956 ) ) ;
#27522=CARTESIAN_POINT ( 'NONE',  ( 4.984841277089891776, 200.2242689037093726, 55.44886208192143329 ) ) ;
#27528=CARTESIAN_POINT ( 'NONE',  ( 0.05014649552807549926, 219.6175466908591716, 61.25113791807856245 ) ) ;
#27529=CARTESIAN_POINT ( 'NONE',  ( 4.102348501002488490, 207.3577873115561943, -8.835681806194324750 ) ) ;
#27530=CARTESIAN_POINT ( 'NONE',  ( 12.01549611932652972, 210.8513442034534933, 1.851137918078565647 ) ) ;
#27531=CARTESIAN_POINT ( 'NONE',  ( 6.139770520408367460, 198.4640165459539389, 80.45113791807857240 ) ) ;
#27532=CARTESIAN_POINT ( 'NONE',  ( 7.375838497908012492, 217.2372850707501186, 39.54886208192143471 ) ) ;
#27533=CARTESIAN_POINT ( 'NONE',  ( -3.044812012439970683, 197.4746971517856196, 46.89886208192143613 ) ) ;
#27535=CARTESIAN_POINT ( 'NONE',  ( -7.456977232089304408, 196.8216656703010301, 84.05113791807858092 ) ) ;
#27536=CARTESIAN_POINT ( 'NONE',  ( 0.05014649552807626948, 215.4116977939061144, 94.25113791807859798 ) ) ;
#27537=CARTESIAN_POINT ( 'NONE',  ( 8.062137200540822946, 212.9164362838583315, 60.69886208192143329 ) ) ;
#27540=CARTESIAN_POINT ( 'NONE',  ( -12.00000000000000711, 206.9523078486584780, 71.49886208192144466 ) ) ;
#27543=CARTESIAN_POINT ( 'NONE',  ( 6.500168698208244500, 202.3363017425938324, 46.29886208192144892 ) ) ;
#27549=CARTESIAN_POINT ( 'NONE',  ( -8.015496119326531499, 204.4483345814780364, 63.35113791807857098 ) ) ;
#27551=CARTESIAN_POINT ( 'NONE',  ( 8.118202686958138514, 201.1607312380088501, 40.29886208192143471 ) ) ;
#27557=CARTESIAN_POINT ( 'NONE',  ( -6.500168698208244500, 211.6636982574061676, 23.79886208192143826 ) ) ;
#27558=CARTESIAN_POINT ( 'NONE',  ( -6.139770520408369237, 215.5359834540460042, 60.95113791807857950 ) ) ;
#27559=CARTESIAN_POINT ( 'NONE',  ( 6.220909254589536808, 215.4770327129947702, 49.55113791807855250 ) ) ;
#27561=CARTESIAN_POINT ( 'NONE',  ( 9.984503880673470277, 203.7031108863295401, 17.15113791807856103 ) ) ;
#27562=CARTESIAN_POINT ( 'NONE',  ( 6.444103211791042618, 202.2591342207267644, 8.301137918078564937 ) ) ;
#27565=CARTESIAN_POINT ( 'NONE',  ( -0.05014649552807705357, 194.3824533091408000, 26.75113791807856956 ) ) ;
#27566=DIRECTION ( 'NONE',  ( 0.000000000000000000, 0.9988620819214357738, 0.04769215134144196705 ) ) ;
#27567=CARTESIAN_POINT ( 'NONE',  ( 0.05014649552810505201, 217.5146222423826714, 73.25113791807855534 ) ) ;
#27568=CARTESIAN_POINT ( 'NONE',  ( 8.118202686958039038, 212.8392687619912635, 49.70113791807857240 ) ) ;
#27573=CARTESIAN_POINT ( 'NONE',  ( -12.00000000000000711, 206.9523078486584780, 17.49886208192143400 ) ) ;
#27574=CARTESIAN_POINT ( 'NONE',  ( 10.00000000000000711, 207.0476921513415220, 18.99886208192143755 ) ) ;
#27577=CARTESIAN_POINT ( 'NONE',  ( -9.680171189290831535, 214.0920067884431148, 60.80113791807858092 ) ) ;
#27578=CARTESIAN_POINT ( 'NONE',  ( -6.500168698208129925, 202.3363017425936050, 66.20113791807857240 ) ) ;
#27579=CARTESIAN_POINT ( 'NONE',  ( 10.00000000000000711, 207.0476921513415220, 27.99886208192143755 ) ) ;
#27583=CARTESIAN_POINT ( 'NONE',  ( -6.139770520408369237, 215.5359834540460042, 90.95113791807854398 ) ) ;
#27588=CARTESIAN_POINT ( 'NONE',  ( 6.444103211791042618, 202.2591342207267644, 32.30113791807856671 ) ) ;
#27593=CARTESIAN_POINT ( 'NONE',  ( -6.220909254589682469, 215.4770327129946850, 11.94886208192143684 ) ) ;
#27596=CARTESIAN_POINT ( 'NONE',  ( -8.015496119326531499, 204.4483345814780364, 54.35113791807857098 ) ) ;
#27600=CARTESIAN_POINT ( 'NONE',  ( 6.220909254589681581, 198.5229672870052582, 97.44886208192143329 ) ) ;
#27602=CARTESIAN_POINT ( 'NONE',  ( -8.118202686958039038, 201.1607312380087080, 30.20113791807856884 ) ) ;
#27604=CARTESIAN_POINT ( 'NONE',  ( 10.00000000000000711, 206.9523078486586201, 14.00113791807856600 ) ) ;
#27610=CARTESIAN_POINT ( 'NONE',  ( 11.98450388067348271, 203.0532714938637753, 2.151137918078565914 ) ) ;
#27613=CARTESIAN_POINT ( 'NONE',  ( -3.044812012440131443, 216.5253028482142952, 46.10113791807857098 ) ) ;
#27619=CARTESIAN_POINT ( 'NONE',  ( -0.05014649552807705357, 194.3824533091408000, 26.75113791807856956 ) ) ;
#27620=AXIS2_PLACEMENT_3D ( 'NONE', #12783, #8012, #31176 ) ;
#27626=CARTESIAN_POINT ( 'NONE',  ( -3.753561863808878130, 218.3979405102790281, 45.09886208192143897 ) ) ;
#27628=CARTESIAN_POINT ( 'NONE',  ( -8.062137200540920645, 212.9164362838581894, 60.80113791807857382 ) ) ;
#27630=CARTESIAN_POINT ( 'NONE',  ( -6.444103211790928043, 202.2591342207265939, 20.19886208192143684 ) ) ;
#27634=CARTESIAN_POINT ( 'NONE',  ( 6.500168698208129925, 211.6636982574063381, 1.701137918078565958 ) ) ;
#27637=CARTESIAN_POINT ( 'NONE',  ( 11.98450388067341876, 210.9467285061363953, 87.84886208192142476 ) ) ;
#27641=CARTESIAN_POINT ( 'NONE',  ( 9.576885917778305668, 206.5919175358980624, 112.0468591418754869 ) ) ;
#27644=CARTESIAN_POINT ( 'NONE',  ( 6.220909254589681581, 198.5229672870052582, 73.44886208192139065 ) ) ;
#27647=CARTESIAN_POINT ( 'NONE',  ( -3.044812012440131443, 216.5253028482142952, 4.101137918078565647 ) ) ;
#27653=CARTESIAN_POINT ( 'NONE',  ( -8.000000000000008882, 206.9523078486584780, 86.49886208192144466 ) ) ;
#27656=CARTESIAN_POINT ( 'NONE',  ( -11.98450388067341876, 203.0532714938636047, 86.34886208192143897 ) ) ;
#27659=CARTESIAN_POINT ( 'NONE',  ( 3.044812012440130555, 197.4746971517856764, 17.60113791807856742 ) ) ;
#27663=CARTESIAN_POINT ( 'NONE',  ( 9.736236675707914401, 214.0148392665762458, 88.70113791807857240 ) ) ;
#27665=CARTESIAN_POINT ( 'NONE',  ( -10.00000000000000711, 207.0476921513413515, 102.5011379180785838 ) ) ;
#27667=CARTESIAN_POINT ( 'NONE',  ( -3.662846001189865142, 195.5725841191952838, 67.89886208192143613 ) ) ;
#27668=CARTESIAN_POINT ( 'NONE',  ( -8.118202686958138514, 212.8392687619910930, 77.79886208192144181 ) ) ;
#27669=CARTESIAN_POINT ( 'NONE',  ( -0.05014649552828442242, 219.6175466908591716, 9.248862081921435774 ) ) ;
#27672=CARTESIAN_POINT ( 'NONE',  ( 8.118202686958039038, 212.8392687619912635, 28.70113791807856884 ) ) ;
#27675=CARTESIAN_POINT ( 'NONE',  ( -8.118202686958138514, 212.8392687619910930, 98.79886208192144181 ) ) ;
#27681=CARTESIAN_POINT ( 'NONE',  ( -4.984841277089891776, 213.7757310962905990, 83.94886208192144750 ) ) ;
#27690=CARTESIAN_POINT ( 'NONE',  ( 2.426778023690261410, 199.3768101843759837, 74.60113791807854966 ) ) ;
#27693=CARTESIAN_POINT ( 'NONE',  ( -2.426778023690076225, 199.3768101843759553, 55.89886208192144323 ) ) ;
#27703=CARTESIAN_POINT ( 'NONE',  ( -9.736236675707914401, 199.9851607334237542, 54.20113791807856529 ) ) ;
#27706=CARTESIAN_POINT ( 'NONE',  ( 8.062137200540920645, 201.0835637161417822, 101.3011379180785809 ) ) ;
#27708=CARTESIAN_POINT ( 'NONE',  ( -10.00000000000000711, 207.0476921513413515, 75.50113791807858377 ) ) ;
#27709=CARTESIAN_POINT ( 'NONE',  ( -7.456977232089471386, 217.1783343296987709, 41.94886208192144039 ) ) ;
#27710=CARTESIAN_POINT ( 'NONE',  ( 3.135527875058981895, 197.5041725223112792, 46.59886208192143187 ) ) ;
#27712=CARTESIAN_POINT ( 'NONE',  ( 3.753561863808689836, 218.3979405102790565, 88.40113791807857524 ) ) ;
#27714=CARTESIAN_POINT ( 'NONE',  ( 10.00000000000000711, 206.9523078486586201, 2.001137918078565558 ) ) ;
#27716=CARTESIAN_POINT ( 'NONE',  ( -8.062137200540822946, 201.0835637161416400, 74.19886208192143329 ) ) ;
#27719=CARTESIAN_POINT ( 'NONE',  ( -11.98450388067341876, 203.0532714938636047, 74.34886208192142476 ) ) ;
#27722=CARTESIAN_POINT ( 'NONE',  ( -6.444103211790928043, 202.2591342207265939, 47.19886208192144750 ) ) ;
#27729=CARTESIAN_POINT ( 'NONE',  ( -3.135527875058982783, 216.4958274776886924, 45.09886208192143897 ) ) ;
#27734=CARTESIAN_POINT ( 'NONE',  ( 6.500168698208244500, 202.3363017425938324, 28.29886208192143826 ) ) ;
#27735=CARTESIAN_POINT ( 'NONE',  ( -6.220909254589537696, 198.5229672870051161, 63.05113791807858092 ) ) ;
#27736=CARTESIAN_POINT ( 'NONE',  ( 9.984503880673470277, 203.7031108863295401, 44.15113791807856813 ) ) ;
#27738=CARTESIAN_POINT ( 'NONE',  ( -6.139770520408369237, 215.5359834540460042, 18.95113791807856884 ) ) ;
#27739=CARTESIAN_POINT ( 'NONE',  ( -7.984503880673488041, 209.6470497212046098, 3.651137918078566802 ) ) ;
#27743=CARTESIAN_POINT ( 'NONE',  ( 7.375838497908181246, 196.7627149292499666, 32.45113791807856529 ) ) ;
#27745=CARTESIAN_POINT ( 'NONE',  ( 10.01549611932653860, 210.2015048109876716, 79.85113791807853545 ) ) ;
#27746=CARTESIAN_POINT ( 'NONE',  ( -8.062137200540920645, 212.9164362838581894, 51.80113791807857382 ) ) ;
#27749=CARTESIAN_POINT ( 'NONE',  ( -3.662846001189865142, 195.5725841191952838, 10.89886208192143613 ) ) ;
#27750=CARTESIAN_POINT ( 'NONE',  ( -3.135527875058982783, 216.4958274776886924, 15.09886208192143542 ) ) ;
#27753=CARTESIAN_POINT ( 'NONE',  ( 9.680171189290831535, 199.9079932115568852, 62.30113791807858092 ) ) ;
#27754=CARTESIAN_POINT ( 'NONE',  ( -8.000000000000008882, 207.0476921513413515, 75.50113791807856956 ) ) ;
#27755=CARTESIAN_POINT ( 'NONE',  ( -10.01549611932659722, 210.2015048109875011, 26.64886208192142902 ) ) ;
#27763=CARTESIAN_POINT ( 'NONE',  ( -6.500168698208129925, 202.3363017425936050, 33.20113791807857240 ) ) ;
#27765=CARTESIAN_POINT ( 'NONE',  ( 3.044812012439969795, 216.5253028482143520, 18.39886208192143613 ) ) ;
#27768=CARTESIAN_POINT ( 'NONE',  ( -8.015496119326531499, 204.4483345814780364, 45.35113791807857098 ) ) ;
#27771=CARTESIAN_POINT ( 'NONE',  ( 3.044812012439969795, 216.5253028482143520, 96.39886208192145034 ) ) ;
#27773=CARTESIAN_POINT ( 'NONE',  ( 3.135527875058820690, 216.4958274776887492, 31.40113791807857524 ) ) ;
#27775=CARTESIAN_POINT ( 'NONE',  ( 8.062137200540920645, 201.0835637161417822, 14.30113791807856671 ) ) ;
#27782=CARTESIAN_POINT ( 'NONE',  ( -12.00000000000000711, 207.0476921513413515, 0.5011379180785653364 ) ) ;
#27785=CARTESIAN_POINT ( 'NONE',  ( 10.00000000000000711, 206.9523078486586201, 50.00113791807856956 ) ) ;
#27791=CARTESIAN_POINT ( 'NONE',  ( -12.00000000000000711, 207.0476921513413515, 27.50113791807856956 ) ) ;
#27794=CARTESIAN_POINT ( 'NONE',  ( 7.456977232089471386, 196.8216656703012006, 103.4488620819214475 ) ) ;
#27797=CARTESIAN_POINT ( 'NONE',  ( 3.044812012440130555, 197.4746971517856764, 5.601137918078566535 ) ) ;
#27798=CARTESIAN_POINT ( 'NONE',  ( -0.05014649552810635652, 196.4853777576173002, 65.75113791807856956 ) ) ;
#27799=CARTESIAN_POINT ( 'NONE',  ( 7.984503880673422316, 209.6470497212048372, 27.84886208192143897 ) ) ;
#27802=CARTESIAN_POINT ( 'NONE',  ( -6.444103211791042618, 211.7408657792732356, 0.8011379180785661580 ) ) ;
#27804=CARTESIAN_POINT ( 'NONE',  ( 11.98450388067341876, 210.9467285061363953, 90.84886208192142476 ) ) ;
#27808=DIRECTION ( 'NONE',  ( -6.106226635438360972E-16, 0.04769215134144213358, -0.9988620819214358848 ) ) ;
#27810=CARTESIAN_POINT ( 'NONE',  ( 3.135527875058981895, 197.5041725223112792, 67.59886208192143897 ) ) ;
#27813=CARTESIAN_POINT ( 'NONE',  ( 10.00000000000000711, 206.9523078486586201, 8.001137918078566003 ) ) ;
#27816=CARTESIAN_POINT ( 'NONE',  ( 8.118202686958039038, 212.8392687619912635, 88.70113791807857240 ) ) ;
#27820=CARTESIAN_POINT ( 'NONE',  ( -9.680171189290716072, 199.9079932115567146, 89.19886208192144750 ) ) ;
#27822=CARTESIAN_POINT ( 'NONE',  ( -8.062137200540920645, 212.9164362838581894, 18.80113791807856671 ) ) ;
#27827=CARTESIAN_POINT ( 'NONE',  ( 0.05014649552807549926, 219.6175466908591716, 85.25113791807856956 ) ) ;
#27831=CARTESIAN_POINT ( 'NONE',  ( 12.01549611932659367, 203.1486557965466773, 67.14886208192143613 ) ) ;
#27832=CARTESIAN_POINT ( 'NONE',  ( 3.044812012439969795, 216.5253028482143520, 75.39886208192143613 ) ) ;
#27833=CARTESIAN_POINT ( 'NONE',  ( -3.753561863808878130, 218.3979405102790281, 15.09886208192143719 ) ) ;
#27835=CARTESIAN_POINT ( 'NONE',  ( -8.118202686958039038, 201.1607312380087080, 36.20113791807857240 ) ) ;
#27837=CARTESIAN_POINT ( 'NONE',  ( -3.135527875058982783, 216.4958274776886924, 102.0988620819214390 ) ) ;
#27842=CARTESIAN_POINT ( 'NONE',  ( 6.500168698208244500, 202.3363017425938324, 82.29886208192144181 ) ) ;
#27844=CARTESIAN_POINT ( 'NONE',  ( 10.00000000000000888, 207.8771832641648984, -0.04188241574673567946 ) ) ;
#27851=CARTESIAN_POINT ( 'NONE',  ( -6.444103211791042618, 211.7408657792732356, 75.80113791807858092 ) ) ;
#27855=CARTESIAN_POINT ( 'NONE',  ( -6.444103211790928043, 202.2591342207265939, 50.19886208192144750 ) ) ;
#27862=CARTESIAN_POINT ( 'NONE',  ( -7.456977232089304408, 196.8216656703010301, 57.05113791807856671 ) ) ;
#27864=CARTESIAN_POINT ( 'NONE',  ( 12.00000000000000711, 206.9523078486586485, -0.9988620819214344415 ) ) ;
#27865=CARTESIAN_POINT ( 'NONE',  ( -3.044812012440131443, 216.5253028482142952, 79.10113791807857808 ) ) ;
#27866=CARTESIAN_POINT ( 'NONE',  ( 7.456977232089471386, 196.8216656703012006, 46.44886208192143329 ) ) ;
#27868=CARTESIAN_POINT ( 'NONE',  ( -6.220909254589682469, 215.4770327129947134, 50.94886208192142618 ) ) ;
#27870=CARTESIAN_POINT ( 'NONE',  ( 3.662846001190051659, 195.5725841191953691, 86.60113791807857808 ) ) ;
#27872=CARTESIAN_POINT ( 'NONE',  ( -3.135527875058821579, 197.5041725223112223, 5.901137918078566358 ) ) ;
#27873=CARTESIAN_POINT ( 'NONE',  ( -10.00000000000000711, 206.9523078486584495, 68.49886208192143044 ) ) ;
#27876=CARTESIAN_POINT ( 'NONE',  ( -0.05014649552828442242, 219.6175466908591716, 75.24886208192143044 ) ) ;
#27880=CARTESIAN_POINT ( 'NONE',  ( -8.000000000000008882, 206.9523078486584780, 56.49886208192145176 ) ) ;
#27891=CARTESIAN_POINT ( 'NONE',  ( 10.01549611932659545, 203.7984951890123853, 40.14886208192143613 ) ) ;
#27898=CARTESIAN_POINT ( 'NONE',  ( 0.05014649552828262524, 198.5883022060938572, 28.74886208192144110 ) ) ;
#27900=CARTESIAN_POINT ( 'NONE',  ( -8.118202686958039038, 201.1607312380087080, 66.20113791807857240 ) ) ;
#27902=CARTESIAN_POINT ( 'NONE',  ( -6.220909254589537696, 198.5229672870051161, 42.05113791807857382 ) ) ;
#27904=CARTESIAN_POINT ( 'NONE',  ( 3.135527875058820690, 216.4958274776887492, 19.40113791807856813 ) ) ;
#27905=CARTESIAN_POINT ( 'NONE',  ( 8.000000000000008882, 206.9523078486586485, 5.001137918078565114 ) ) ;
#27909=CARTESIAN_POINT ( 'NONE',  ( -12.01549611932652972, 203.1486557965464499, 33.35113791807857098 ) ) ;
#27912=CARTESIAN_POINT ( 'NONE',  ( 6.220909254589536808, 215.4770327129947702, 73.55113791807858092 ) ) ;
#27913=CARTESIAN_POINT ( 'NONE',  ( -6.220909254589537696, 198.5229672870051445, 48.05113791807857382 ) ) ;
#27916=CARTESIAN_POINT ( 'NONE',  ( 9.680171189290716072, 214.0920067884432854, 15.69886208192143684 ) ) ;
#27917=CARTESIAN_POINT ( 'NONE',  ( 10.01549611932659367, 203.7984951890124421, 22.14886208192143613 ) ) ;
#27920=CARTESIAN_POINT ( 'NONE',  ( 7.375838497908181246, 196.7627149292499666, 59.45113791807857240 ) ) ;
#27921=CARTESIAN_POINT ( 'NONE',  ( 8.000000000000008882, 206.9523078486586485, 77.00113791807858377 ) ) ;
#27922=CARTESIAN_POINT ( 'NONE',  ( 9.984503880673420539, 210.2968891136705167, 36.84886208192143187 ) ) ;
#27935=CARTESIAN_POINT ( 'NONE',  ( 8.015496119326531499, 209.5516654185219636, 34.85113791807857098 ) ) ;
#27938=CARTESIAN_POINT ( 'NONE',  ( 6.220909254589681581, 198.5229672870052582, 13.44886208192143151 ) ) ;
#27942=CARTESIAN_POINT ( 'NONE',  ( -2.426778023690262742, 214.6231898156240163, 64.10113791807857808 ) ) ;
#27946=CARTESIAN_POINT ( 'NONE',  ( 3.135527875058981895, 197.5041725223112792, 97.59886208192143897 ) ) ;
#27948=CARTESIAN_POINT ( 'NONE',  ( -8.118202686958039038, 201.1607312380087080, 36.20113791807857240 ) ) ;
#27950=CARTESIAN_POINT ( 'NONE',  ( 0.05014649552810505201, 217.5146222423826714, 16.25113791807856600 ) ) ;
#27956=CARTESIAN_POINT ( 'NONE',  ( 0.05014649552807549926, 219.6175466908591716, 4.251137918078565114 ) ) ;
#27959=CARTESIAN_POINT ( 'NONE',  ( 9.984503880673470277, 203.7031108863295401, 44.15113791807856813 ) ) ;
#27966=CARTESIAN_POINT ( 'NONE',  ( -0.05014649552807705357, 194.3824533091408000, 32.75113791807856956 ) ) ;
#27969=CARTESIAN_POINT ( 'NONE',  ( -10.00000000000000711, 206.9523078486584495, 11.49886208192143577 ) ) ;
#27972=CARTESIAN_POINT ( 'NONE',  ( -10.00000000000000711, 207.0476921513413515, 3.501137918078566003 ) ) ;
#27973=CARTESIAN_POINT ( 'NONE',  ( -3.044812012440131443, 216.5253028482142952, 58.10113791807857808 ) ) ;
#27975=CARTESIAN_POINT ( 'NONE',  ( 4.903702542908435547, 213.8346818373419751, 24.54886208192144181 ) ) ;
#27978=CARTESIAN_POINT ( 'NONE',  ( 6.444103211791042618, 202.2591342207267644, 5.301137918078567601 ) ) ;
#27980=CARTESIAN_POINT ( 'NONE',  ( -7.375838497908014268, 196.7627149292498530, 92.04886208192142760 ) ) ;
#27987=CARTESIAN_POINT ( 'NONE',  ( 6.220909254589681581, 198.5229672870052582, 67.44886208192143329 ) ) ;
#27990=CARTESIAN_POINT ( 'NONE',  ( -6.139770520408369237, 215.5359834540460042, 3.951137918078566180 ) ) ;
#27994=CARTESIAN_POINT ( 'NONE',  ( 3.135527875058820690, 216.4958274776887492, 94.40113791807857524 ) ) ;
#27996=CARTESIAN_POINT ( 'NONE',  ( -10.01549611932653860, 203.7984951890123284, 72.35113791807859229 ) ) ;
#27999=CARTESIAN_POINT ( 'NONE',  ( 7.456977232089471386, 196.8216656703012006, 91.44886208192143329 ) ) ;
#28001=CARTESIAN_POINT ( 'NONE',  ( 6.220909254589536808, 215.4770327129947987, 28.55113791807856671 ) ) ;
#28005=CARTESIAN_POINT ( 'NONE',  ( 0.05014649552807549926, 219.6175466908591716, 97.25113791807856956 ) ) ;
#28008=CARTESIAN_POINT ( 'NONE',  ( -0.05014649552828402690, 217.5146222423826714, 87.24886208192144466 ) ) ;
#28009=CARTESIAN_POINT ( 'NONE',  ( -12.00000000000000711, 206.9523078486584780, 11.49886208192143577 ) ) ;
#28011=CARTESIAN_POINT ( 'NONE',  ( -9.984503880673473830, 210.2968891136704315, 36.65113791807855392 ) ) ;
#28013=CARTESIAN_POINT ( 'NONE',  ( 8.062137200540822946, 212.9164362838583315, 99.69886208192144750 ) ) ;
#28018=CARTESIAN_POINT ( 'NONE',  ( 4.903702542908435547, 213.8346818373419751, 78.54886208192142760 ) ) ;
#28026=CARTESIAN_POINT ( 'NONE',  ( 6.444103211791042618, 202.2591342207267644, 80.30113791807858092 ) ) ;
#28031=CARTESIAN_POINT ( 'NONE',  ( -2.426778023690076225, 199.3768101843759553, 52.89886208192144323 ) ) ;
#28034=CARTESIAN_POINT ( 'NONE',  ( 10.01549611932653860, 210.2015048109876716, 1.851137918078565425 ) ) ;
#28039=CARTESIAN_POINT ( 'NONE',  ( 7.456977232089302632, 217.1783343296989131, 61.55113791807858092 ) ) ;
#28041=CARTESIAN_POINT ( 'NONE',  ( -12.01549611932652972, 203.1486557965464499, 9.351137918078563871 ) ) ;
#28042=CARTESIAN_POINT ( 'NONE',  ( -3.135527875058821579, 197.5041725223112223, 74.90113791807857524 ) ) ;
#28043=CARTESIAN_POINT ( 'NONE',  ( -11.98450388067341876, 203.0532714938636047, 44.34886208192143897 ) ) ;
#28044=CARTESIAN_POINT ( 'NONE',  ( 0.05014649552828275014, 196.4853777576173002, 52.74886208192143755 ) ) ;
#28047=CARTESIAN_POINT ( 'NONE',  ( -9.680171189290831535, 214.0920067884431148, 87.80113791807858092 ) ) ;
#28049=CARTESIAN_POINT ( 'NONE',  ( 8.062137200540920645, 201.0835637161417822, 8.301137918078566713 ) ) ;
#28050=CARTESIAN_POINT ( 'NONE',  ( -8.062137200540822946, 201.0835637161416400, 68.19886208192144750 ) ) ;
#28053=CARTESIAN_POINT ( 'NONE',  ( 12.00000000000000711, 207.0476921513415220, 72.99886208192144466 ) ) ;
#28057=CARTESIAN_POINT ( 'NONE',  ( 4.984841277089891776, 200.2242689037093726, 49.44886208192144750 ) ) ;
#28062=CARTESIAN_POINT ( 'NONE',  ( 10.00000000000000888, 207.0000000000002842, 5.551115123125782702E-14 ) ) ;
#28066=CARTESIAN_POINT ( 'NONE',  ( -6.139770520408224463, 198.4640165459539389, 38.04886208192144181 ) ) ;
#28071=CARTESIAN_POINT ( 'NONE',  ( -2.517493886309087880, 214.5937144450984135, 21.09886208192143897 ) ) ;
#28072=CARTESIAN_POINT ( 'NONE',  ( 0.05014649552810505201, 217.5146222423826714, 67.25113791807856956 ) ) ;
#28074=CARTESIAN_POINT ( 'NONE',  ( -10.01549611932653860, 203.7984951890123284, 51.35113791807858519 ) ) ;
#28076=CARTESIAN_POINT ( 'NONE',  ( 8.062137200540920645, 201.0835637161417822, 20.30113791807856671 ) ) ;
#28077=CARTESIAN_POINT ( 'NONE',  ( -8.000000000000008882, 207.0476921513413515, 9.501137918078566003 ) ) ;
#28080=CARTESIAN_POINT ( 'NONE',  ( 0.05014649552807549926, 219.6175466908591716, 31.25113791807856956 ) ) ;
#28083=CARTESIAN_POINT ( 'NONE',  ( 9.984503880673470277, 203.7031108863295401, 77.15113791807857524 ) ) ;
#28084=CARTESIAN_POINT ( 'NONE',  ( 3.135527875058820690, 216.4958274776887492, 52.40113791807857524 ) ) ;
#28087=CARTESIAN_POINT ( 'NONE',  ( 0.05014649552828288198, 194.3824533091408000, 10.74886208192143577 ) ) ;
#28088=CARTESIAN_POINT ( 'NONE',  ( 3.135527875058981895, 197.5041725223112792, 22.59886208192143542 ) ) ;
#28091=CARTESIAN_POINT ( 'NONE',  ( -12.01549611932652972, 203.1486557965464499, 54.35113791807857098 ) ) ;
#28092=CARTESIAN_POINT ( 'NONE',  ( -8.015496119326531499, 204.4483345814780364, 78.35113791807857808 ) ) ;
#28094=CARTESIAN_POINT ( 'NONE',  ( -0.05014649552828403384, 217.5146222423826714, 45.24886208192143755 ) ) ;
#28105=CARTESIAN_POINT ( 'NONE',  ( 7.984503880673485376, 204.3529502787953902, 32.15113791807857524 ) ) ;
#28107=CARTESIAN_POINT ( 'NONE',  ( 3.135527875058981895, 197.5041725223112792, 16.59886208192143542 ) ) ;
#28110=CARTESIAN_POINT ( 'NONE',  ( 2.426778023690261410, 199.3768101843759837, 56.60113791807857808 ) ) ;
#28113=CARTESIAN_POINT ( 'NONE',  ( 9.984503880673420539, 210.2968891136705167, 96.84886208192139634 ) ) ;
#28115=CARTESIAN_POINT ( 'NONE',  ( -9.984503880673473830, 210.2968891136704315, 39.65113791807857524 ) ) ;
#28117=CARTESIAN_POINT ( 'NONE',  ( -0.05014649552810635652, 196.4853777576173002, 17.75113791807856245 ) ) ;
#28121=CIRCLE ( 'NONE', #8021, 10.62447292484156947 ) ;
#28125=CARTESIAN_POINT ( 'NONE',  ( 0.05014649552807549926, 219.6175466908591716, 1.251137918078565558 ) ) ;
#28129=CARTESIAN_POINT ( 'NONE',  ( -0.05014649552810635652, 196.4853777576173002, 47.75113791807855534 ) ) ;
#28136=CARTESIAN_POINT ( 'NONE',  ( 9.680171189290831535, 199.9079932115568852, 32.30113791807855961 ) ) ;
#28140=CARTESIAN_POINT ( 'NONE',  ( 6.139770520408223575, 215.5359834540460611, 15.54886208192143293 ) ) ;
#28144=CARTESIAN_POINT ( 'NONE',  ( 8.118202686958039038, 212.8392687619912635, 10.70113791807856529 ) ) ;
#28145=CARTESIAN_POINT ( 'NONE',  ( 10.01549611932653860, 210.2015048109876716, 58.85113791807856387 ) ) ;
#28147=ORIENTED_EDGE ( 'NONE', *, *, #164, .T. ) ;
#28148=CARTESIAN_POINT ( 'NONE',  ( 4.903702542908435547, 213.8346818373419751, 21.54886208192143471 ) ) ;
#28153=CARTESIAN_POINT ( 'NONE',  ( -2.517493886308901807, 199.4062855549015012, 5.901137918078568134 ) ) ;
#28154=CARTESIAN_POINT ( 'NONE',  ( 3.662846001189864698, 218.4274158808046593, 93.39886208192143613 ) ) ;
#28161=CARTESIAN_POINT ( 'NONE',  ( 10.00000000000000711, 207.0476921513415220, 69.99886208192143044 ) ) ;
#28164=CARTESIAN_POINT ( 'NONE',  ( -3.044812012440131443, 216.5253028482142952, 16.10113791807856742 ) ) ;
#28168=CARTESIAN_POINT ( 'NONE',  ( -3.044812012440131443, 216.5253028482142952, 94.10113791807857808 ) ) ;
#28170=CARTESIAN_POINT ( 'NONE',  ( -10.00000000000000711, 207.0476921513413515, 75.50113791807858377 ) ) ;
#28174=CARTESIAN_POINT ( 'NONE',  ( -3.662846001189865142, 195.5725841191952838, 91.89886208192143613 ) ) ;
#28178=CARTESIAN_POINT ( 'NONE',  ( 6.139770520408367460, 198.4640165459539389, 29.45113791807856884 ) ) ;
#28182=CARTESIAN_POINT ( 'NONE',  ( -9.736236675707914401, 199.9851607334237542, 99.20113791807858661 ) ) ;
#28186=CARTESIAN_POINT ( 'NONE',  ( -10.01549611932659545, 210.2015048109875011, 86.64886208192142192 ) ) ;
#28187=CARTESIAN_POINT ( 'NONE',  ( 3.753561863808876797, 195.6020594897209719, 25.59886208192143897 ) ) ;
#28189=CARTESIAN_POINT ( 'NONE',  ( 6.220909254589536808, 215.4770327129947702, 34.55113791807855250 ) ) ;
#28191=CARTESIAN_POINT ( 'NONE',  ( 6.139770520408223575, 215.5359834540460611, 102.5488620819214134 ) ) ;
#28195=CARTESIAN_POINT ( 'NONE',  ( 4.984841277089891776, 200.2242689037093726, 76.44886208192143329 ) ) ;
#28201=CARTESIAN_POINT ( 'NONE',  ( 6.500168698208129925, 211.6636982574063381, 58.70113791807857240 ) ) ;
#28204=CARTESIAN_POINT ( 'NONE',  ( 8.015496119326531499, 209.5516654185219636, 76.85113791807856387 ) ) ;
#28209=CARTESIAN_POINT ( 'NONE',  ( -4.903702542908436435, 200.1653181626580249, 68.04886208192144181 ) ) ;
#28215=CARTESIAN_POINT ( 'NONE',  ( 3.753561863808689836, 218.3979405102790565, 64.40113791807856103 ) ) ;
#28219=CARTESIAN_POINT ( 'NONE',  ( -9.680171189290831535, 214.0920067884431148, 9.801137918078564937 ) ) ;
#28220=CARTESIAN_POINT ( 'NONE',  ( 10.01549611932653860, 210.2015048109876716, 85.85113791807857808 ) ) ;
#28222=CARTESIAN_POINT ( 'NONE',  ( -7.375838497908014268, 196.7627149292498530, 56.04886208192144181 ) ) ;
#28223=CARTESIAN_POINT ( 'NONE',  ( -9.984503880673420539, 203.7031108863293980, 53.34886208192144608 ) ) ;
#28225=CARTESIAN_POINT ( 'NONE',  ( -7.375838497908182134, 217.2372850707499765, 96.95113791807857240 ) ) ;
#28227=CARTESIAN_POINT ( 'NONE',  ( -10.01549611932653860, 203.7984951890123284, 0.3511379180785655363 ) ) ;
#28228=CARTESIAN_POINT ( 'NONE',  ( 6.139770520408223575, 215.5359834540460611, 66.54886208192144181 ) ) ;
#28233=CARTESIAN_POINT ( 'NONE',  ( 12.00000000000000711, 207.0476921513415220, 66.99886208192144466 ) ) ;
#28234=CARTESIAN_POINT ( 'NONE',  ( 6.220909254589536808, 215.4770327129947702, 85.55113791807858092 ) ) ;
#28237=CARTESIAN_POINT ( 'NONE',  ( -6.500168698208244500, 211.6636982574061676, 53.79886208192144892 ) ) ;
#28245=CARTESIAN_POINT ( 'NONE',  ( 9.984503880673420539, 210.2968891136705167, 54.84886208192141765 ) ) ;
#28251=CARTESIAN_POINT ( 'NONE',  ( 4.984841277089891776, 200.2242689037093726, 34.44886208192144039 ) ) ;
#28252=CARTESIAN_POINT ( 'NONE',  ( 6.220909254589536808, 215.4770327129947702, 73.55113791807858092 ) ) ;
#28254=CARTESIAN_POINT ( 'NONE',  ( -6.139770520408369237, 215.5359834540460042, 57.95113791807856529 ) ) ;
#28257=CARTESIAN_POINT ( 'NONE',  ( -9.984503880673473830, 210.2968891136704315, 30.65113791807856813 ) ) ;
#28258=CARTESIAN_POINT ( 'NONE',  ( -8.015496119326531499, 204.4483345814780364, 6.351137918078565647 ) ) ;
#28262=CARTESIAN_POINT ( 'NONE',  ( 9.680171189290831535, 199.9079932115568852, 41.30113791807857382 ) ) ;
#28264=CARTESIAN_POINT ( 'NONE',  ( 9.984503880673470277, 203.7031108863295401, 86.15113791807857524 ) ) ;
#28265=CARTESIAN_POINT ( 'NONE',  ( -9.984503880673475606, 210.2968891136704315, 51.65113791807855392 ) ) ;
#28267=CARTESIAN_POINT ( 'NONE',  ( -11.98450388067341876, 203.0532714938636047, 17.34886208192143187 ) ) ;
#28268=CARTESIAN_POINT ( 'NONE',  ( 8.118202686958138514, 201.1607312380088501, 25.29886208192143826 ) ) ;
#28270=VERTEX_POINT ( 'NONE', #21326 ) ;
#28271=CARTESIAN_POINT ( 'NONE',  ( 7.375838497908181246, 196.7627149292499666, 65.45113791807858661 ) ) ;
#28273=CARTESIAN_POINT ( 'NONE',  ( 0.05014649552807626948, 215.4116977939061144, 79.25113791807856956 ) ) ;
#28274=CARTESIAN_POINT ( 'NONE',  ( -6.139770520408224463, 198.4640165459539389, 38.04886208192144181 ) ) ;
#28278=CARTESIAN_POINT ( 'NONE',  ( 9.736236675708031640, 199.9851607334238963, 46.29886208192144181 ) ) ;
#28285=CARTESIAN_POINT ( 'NONE',  ( -7.984503880673488041, 209.6470497212046098, 39.65113791807857524 ) ) ;
#28287=CARTESIAN_POINT ( 'NONE',  ( 9.984503880673420539, 210.2968891136705167, 21.84886208192143542 ) ) ;
#28290=CARTESIAN_POINT ( 'NONE',  ( 8.015496119326531499, 209.5516654185219636, 61.85113791807857098 ) ) ;
#28294=CARTESIAN_POINT ( 'NONE',  ( -10.01549611932659722, 210.2015048109875011, 98.64886208192143613 ) ) ;
#28296=CARTESIAN_POINT ( 'NONE',  ( -10.01549611932653860, 203.7984951890123284, 42.35113791807855677 ) ) ;
#28299=CARTESIAN_POINT ( 'NONE',  ( 9.984503880673470277, 203.7031108863295401, 23.15113791807856813 ) ) ;
#28300=CARTESIAN_POINT ( 'NONE',  ( 0.05014649552828275014, 196.4853777576173002, 100.7488620819214304 ) ) ;
#28301=CARTESIAN_POINT ( 'NONE',  ( 4.984841277089891776, 200.2242689037093726, 82.44886208192144750 ) ) ;
#28304=CARTESIAN_POINT ( 'NONE',  ( 9.736236675707914401, 214.0148392665762458, 4.701137918078565292 ) ) ;
#28308=CARTESIAN_POINT ( 'NONE',  ( -8.118202686958039038, 201.1607312380087080, 60.20113791807857240 ) ) ;
#28314=CARTESIAN_POINT ( 'NONE',  ( -9.736236675707914401, 199.9851607334237542, 33.20113791807856529 ) ) ;
#28316=CARTESIAN_POINT ( 'NONE',  ( -3.044812012439970683, 197.4746971517856196, 10.89886208192143613 ) ) ;
#28319=CARTESIAN_POINT ( 'NONE',  ( -10.01549611932653860, 203.7984951890123284, 6.351137918078566535 ) ) ;
#28320=CARTESIAN_POINT ( 'NONE',  ( -8.062137200540920645, 212.9164362838581894, 75.80113791807858092 ) ) ;
#28322=CARTESIAN_POINT ( 'NONE',  ( 6.444103211790928043, 211.7408657792734061, 30.69886208192143684 ) ) ;
#28324=EDGE_LOOP ( 'NONE', ( #4460, #10930, #9798, #489, #5236, #5027 ) ) ;
#28325=CARTESIAN_POINT ( 'NONE',  ( -4.984841277089726574, 200.2242689037092305, 0.05113791807856601229 ) ) ;
#28328=CARTESIAN_POINT ( 'NONE',  ( -3.753561863808878130, 218.3979405102790281, 87.09886208192143897 ) ) ;
#28333=CARTESIAN_POINT ( 'NONE',  ( -6.220909254589537696, 198.5229672870051161, 6.051137918078566713 ) ) ;
#28335=CARTESIAN_POINT ( 'NONE',  ( 6.139770520408223575, 215.5359834540460611, 72.54886208192144181 ) ) ;
#28339=CARTESIAN_POINT ( 'NONE',  ( 3.044812012440130555, 197.4746971517856764, 11.60113791807856742 ) ) ;
#28343=CARTESIAN_POINT ( 'NONE',  ( 10.00000000000000711, 206.9523078486586201, 95.00113791807856956 ) ) ;
#28345=CARTESIAN_POINT ( 'NONE',  ( 6.139770520408368348, 198.4640165459539674, 74.45113791807857240 ) ) ;
#28349=CARTESIAN_POINT ( 'NONE',  ( -3.753561863808878130, 218.3979405102790281, 90.09886208192143897 ) ) ;
#28354=CARTESIAN_POINT ( 'NONE',  ( 12.01549611932652972, 210.8513442034534933, 97.85113791807857808 ) ) ;
#28357=CARTESIAN_POINT ( 'NONE',  ( 8.062137200540822946, 212.9164362838583315, 81.69886208192143329 ) ) ;
#28359=CARTESIAN_POINT ( 'NONE',  ( -9.736236675708031640, 214.0148392665760753, 20.79886208192143826 ) ) ;
#28361=CARTESIAN_POINT ( 'NONE',  ( -8.062137200540920645, 212.9164362838581894, 42.80113791807857382 ) ) ;
#28363=CARTESIAN_POINT ( 'NONE',  ( 8.118202686958138514, 201.1607312380088501, 97.29886208192144181 ) ) ;
#28366=CARTESIAN_POINT ( 'NONE',  ( 8.000000000000008882, 207.0476921513415220, 84.99886208192144466 ) ) ;
#28371=CARTESIAN_POINT ( 'NONE',  ( 4.903702542908601636, 200.1653181626581102, 62.45113791807857240 ) ) ;
#28375=CARTESIAN_POINT ( 'NONE',  ( 6.444103211791042618, 202.2591342207267644, 92.30113791807858092 ) ) ;
#28379=CARTESIAN_POINT ( 'NONE',  ( -8.000000000000008882, 206.9523078486584780, 62.49886208192144466 ) ) ;
#28382=CARTESIAN_POINT ( 'NONE',  ( -0.05014649552810635652, 196.4853777576173002, -0.2488620819214343305 ) ) ;
#28387=CARTESIAN_POINT ( 'NONE',  ( -3.662846001190052991, 218.4274158808045740, 67.10113791807857808 ) ) ;
#28389=CARTESIAN_POINT ( 'NONE',  ( 9.680171189290831535, 199.9079932115568852, 14.30113791807856849 ) ) ;
#28390=CARTESIAN_POINT ( 'NONE',  ( 9.984503880673473830, 203.7031108863295401, 89.15113791807857524 ) ) ;
#28391=CARTESIAN_POINT ( 'NONE',  ( -12.01549611932659722, 210.8513442034533227, 47.64886208192143613 ) ) ;
#28392=CARTESIAN_POINT ( 'NONE',  ( 10.01549611932659367, 203.7984951890124421, 55.14886208192143613 ) ) ;
#28394=CARTESIAN_POINT ( 'NONE',  ( 9.736236675707914401, 214.0148392665762458, 97.70113791807858661 ) ) ;
#28396=CARTESIAN_POINT ( 'NONE',  ( 6.139770520408368348, 198.4640165459539674, 14.45113791807856352 ) ) ;
#28397=CARTESIAN_POINT ( 'NONE',  ( 3.044812012439969795, 216.5253028482143520, 69.39886208192143613 ) ) ;
#28399=CARTESIAN_POINT ( 'NONE',  ( -3.662846001189865142, 195.5725841191952838, 76.89886208192143613 ) ) ;
#28400=CARTESIAN_POINT ( 'NONE',  ( 8.118202686958039038, 212.8392687619912635, 94.70113791807857240 ) ) ;
#28401=ORIENTED_EDGE ( 'NONE', *, *, #16174, .F. ) ;
#28403=CARTESIAN_POINT ( 'NONE',  ( 6.500168698208244500, 202.3363017425938324, 55.29886208192144892 ) ) ;
#28411=CARTESIAN_POINT ( 'NONE',  ( 10.01549611932659545, 203.7984951890123853, 49.14886208192143613 ) ) ;
#28416=CARTESIAN_POINT ( 'NONE',  ( 2.426778023690075337, 214.6231898156240447, 39.39886208192144323 ) ) ;
#28417=CARTESIAN_POINT ( 'NONE',  ( 10.00000000000000711, 206.9523078486586201, 71.00113791807858377 ) ) ;
#28420=CARTESIAN_POINT ( 'NONE',  ( -9.984503880673473830, 210.2968891136704315, 51.65113791807855392 ) ) ;
#28423=CARTESIAN_POINT ( 'NONE',  ( 8.118202686958039038, 212.8392687619912635, 31.70113791807856884 ) ) ;
#28424=CARTESIAN_POINT ( 'NONE',  ( -7.984503880673488041, 209.6470497212046098, 12.65113791807856636 ) ) ;
#28428=CARTESIAN_POINT ( 'NONE',  ( 9.736236675707914401, 214.0148392665762458, 37.70113791807857240 ) ) ;
#28430=CARTESIAN_POINT ( 'NONE',  ( 0.05014649552810505201, 217.5146222423826714, 82.25113791807858377 ) ) ;
#28431=CARTESIAN_POINT ( 'NONE',  ( -10.01549611932653860, 203.7984951890123000, 63.35113791807857098 ) ) ;
#28433=CARTESIAN_POINT ( 'NONE',  ( -7.375838497908014268, 196.7627149292498530, 20.04886208192143471 ) ) ;
#28434=CARTESIAN_POINT ( 'NONE',  ( 8.062137200540822946, 212.9164362838583315, 30.69886208192144039 ) ) ;
#28436=CARTESIAN_POINT ( 'NONE',  ( 3.662846001190051659, 195.5725841191953691, 65.60113791807857808 ) ) ;
#28437=CARTESIAN_POINT ( 'NONE',  ( -6.500168698208129925, 202.3363017425936050, 75.20113791807857240 ) ) ;
#28439=CARTESIAN_POINT ( 'NONE',  ( 6.220909254589681581, 198.5229672870052582, 37.44886208192143329 ) ) ;
#28443=CARTESIAN_POINT ( 'NONE',  ( -12.01549611932659722, 210.8513442034533227, 47.64886208192143613 ) ) ;
#28450=CARTESIAN_POINT ( 'NONE',  ( 8.000000000000008882, 206.9523078486586485, 38.00113791807857666 ) ) ;
#28452=CARTESIAN_POINT ( 'NONE',  ( -10.01549611932659722, 210.2015048109875011, 20.64886208192143613 ) ) ;
#28458=CARTESIAN_POINT ( 'NONE',  ( 7.984503880673422316, 209.6470497212048372, 3.848862081921434530 ) ) ;
#28460=CARTESIAN_POINT ( 'NONE',  ( -0.05014649552810635652, 196.4853777576173002, 38.75113791807856956 ) ) ;
#28463=CARTESIAN_POINT ( 'NONE',  ( 10.00000000000000711, 206.9523078486586201, 26.00113791807856956 ) ) ;
#28464=CARTESIAN_POINT ( 'NONE',  ( 10.01549611932659367, 203.7984951890124421, 103.1488620819214219 ) ) ;
#28466=CARTESIAN_POINT ( 'NONE',  ( 2.426778023690075337, 214.6231898156240447, 81.39886208192143613 ) ) ;
#28470=CARTESIAN_POINT ( 'NONE',  ( 7.375838497908181246, 196.7627149292499666, 14.45113791807856707 ) ) ;
#28474=CARTESIAN_POINT ( 'NONE',  ( -0.05014649552810635652, 196.4853777576173002, 59.75113791807857666 ) ) ;
#28479=CARTESIAN_POINT ( 'NONE',  ( 8.118202686958138514, 201.1607312380088501, 1.298862081921434486 ) ) ;
#28482=CARTESIAN_POINT ( 'NONE',  ( -7.375838497908182134, 217.2372850707499765, 39.95113791807856529 ) ) ;
#28484=CARTESIAN_POINT ( 'NONE',  ( 8.062137200540822946, 212.9164362838583315, 15.69886208192143506 ) ) ;
#28488=CARTESIAN_POINT ( 'NONE',  ( 6.220909254589536808, 215.4770327129947702, 7.551137918078564049 ) ) ;
#28489=CARTESIAN_POINT ( 'NONE',  ( 3.135527875058820690, 216.4958274776887492, 73.40113791807857524 ) ) ;
#28492=CARTESIAN_POINT ( 'NONE',  ( 8.015496119326595448, 204.4483345814782638, 31.14886208192143968 ) ) ;
#28495=CARTESIAN_POINT ( 'NONE',  ( 0.05014649552807626948, 215.4116977939061144, 16.25113791807856600 ) ) ;
#28497=CARTESIAN_POINT ( 'NONE',  ( -7.375838497908014268, 196.7627149292498530, 98.04886208192144181 ) ) ;
#28502=CARTESIAN_POINT ( 'NONE',  ( 8.062137200540920645, 201.0835637161417822, 11.30113791807856671 ) ) ;
#28504=CARTESIAN_POINT ( 'NONE',  ( 9.984503880673420539, 210.2968891136705167, 81.84886208192143897 ) ) ;
#28507=CARTESIAN_POINT ( 'NONE',  ( -0.05014649552810635652, 196.4853777576173002, 11.75113791807856778 ) ) ;
#28513=CARTESIAN_POINT ( 'NONE',  ( -8.118202686958039038, 201.1607312380087080, 96.20113791807857240 ) ) ;
#28515=CARTESIAN_POINT ( 'NONE',  ( 0.05014649552810505201, 217.5146222423826714, 85.25113791807854113 ) ) ;
#28518=CARTESIAN_POINT ( 'NONE',  ( -1.474514954580286030E-14, 206.9977241638431167, -6.000000000000014211 ) ) ;
#28519=CARTESIAN_POINT ( 'NONE',  ( 3.662846001189864698, 218.4274158808046593, 93.39886208192143613 ) ) ;
#28524=CARTESIAN_POINT ( 'NONE',  ( 9.736236675707914401, 214.0148392665762458, 100.7011379180785866 ) ) ;
#28529=CARTESIAN_POINT ( 'NONE',  ( -8.062137200540822946, 201.0835637161416400, 89.19886208192144750 ) ) ;
#28530=CARTESIAN_POINT ( 'NONE',  ( -12.01549611932659722, 210.8513442034533227, 26.64886208192143968 ) ) ;
#28532=CARTESIAN_POINT ( 'NONE',  ( 10.00000000000000711, 206.9523078486586201, 38.00113791807857666 ) ) ;
#28535=CARTESIAN_POINT ( 'NONE',  ( 2.426778023690075337, 214.6231898156240447, 3.398862081921434797 ) ) ;
#28539=CARTESIAN_POINT ( 'NONE',  ( 2.426778023690075337, 214.6231898156240447, 90.39886208192143613 ) ) ;
#28543=CARTESIAN_POINT ( 'NONE',  ( -8.000000000000008882, 207.0476921513413515, 30.50113791807856600 ) ) ;
#28549=CARTESIAN_POINT ( 'NONE',  ( -8.000000000000008882, 207.0476921513413515, 90.50113791807858377 ) ) ;
#28553=CARTESIAN_POINT ( 'NONE',  ( 2.426778023690075337, 214.6231898156240447, 60.39886208192144323 ) ) ;
#28556=CARTESIAN_POINT ( 'NONE',  ( 0.05014649552810506589, 217.5146222423826714, 4.251137918078566003 ) ) ;
#28560=CARTESIAN_POINT ( 'NONE',  ( -12.00000000000000711, 207.0476921513413515, 63.50113791807856956 ) ) ;
#28562=CARTESIAN_POINT ( 'NONE',  ( -12.00000000000000711, 207.0476921513413515, 6.501137918078566891 ) ) ;
#28564=CARTESIAN_POINT ( 'NONE',  ( -10.00000000000000711, 207.0476921513413515, 84.50113791807856956 ) ) ;
#28565=CARTESIAN_POINT ( 'NONE',  ( -12.01549611932659722, 210.8513442034533227, 50.64886208192143613 ) ) ;
#28566=CARTESIAN_POINT ( 'NONE',  ( -9.984503880673420539, 203.7031108863293980, 59.34886208192143187 ) ) ;
#28567=CARTESIAN_POINT ( 'NONE',  ( 3.753561863808689836, 218.3979405102790565, 100.4011379180785895 ) ) ;
#28568=CARTESIAN_POINT ( 'NONE',  ( -3.135527875058821579, 197.5041725223112223, 8.901137918078566358 ) ) ;
#28570=CARTESIAN_POINT ( 'NONE',  ( -8.118202686958138514, 212.8392687619910930, 77.79886208192144181 ) ) ;
#28572=CARTESIAN_POINT ( 'NONE',  ( 3.753561863808876797, 195.6020594897209719, 79.59886208192143897 ) ) ;
#28573=CARTESIAN_POINT ( 'NONE',  ( -6.139770520408369237, 215.5359834540460042, 96.95113791807857240 ) ) ;
#28576=CARTESIAN_POINT ( 'NONE',  ( 4.984841277089891776, 200.2242689037093726, 55.44886208192143329 ) ) ;
#28583=CARTESIAN_POINT ( 'NONE',  ( -8.118202686958138514, 212.8392687619910930, 50.79886208192143471 ) ) ;
#28584=ORIENTED_EDGE ( 'NONE', *, *, #15586, .T. ) ;
#28588=CARTESIAN_POINT ( 'NONE',  ( 8.015496119326595448, 204.4483345814782638, 34.14886208192144323 ) ) ;
#28589=CARTESIAN_POINT ( 'NONE',  ( 9.984503880673470277, 203.7031108863295401, 74.15113791807854682 ) ) ;
#28591=CARTESIAN_POINT ( 'NONE',  ( -8.062137200540920645, 212.9164362838581894, 51.80113791807857382 ) ) ;
#28593=CARTESIAN_POINT ( 'NONE',  ( 6.139770520408368348, 198.4640165459539674, 23.45113791807856884 ) ) ;
#28594=CARTESIAN_POINT ( 'NONE',  ( -2.426778023690262742, 214.6231898156240163, 16.10113791807856742 ) ) ;
#28597=CARTESIAN_POINT ( 'NONE',  ( 12.00000000000000711, 206.9523078486586485, 35.00113791807857666 ) ) ;
#28599=CARTESIAN_POINT ( 'NONE',  ( -9.984503880673473830, 210.2968891136704315, 87.65113791807854682 ) ) ;
#28600=CARTESIAN_POINT ( 'NONE',  ( -10.00000000000000711, 207.0476921513413515, 57.50113791807856956 ) ) ;
#28602=CARTESIAN_POINT ( 'NONE',  ( -12.00000000000000711, 206.9523078486584780, 26.49886208192143400 ) ) ;
#28603=CARTESIAN_POINT ( 'NONE',  ( -6.220909254589682469, 215.4770327129947134, 32.94886208192144039 ) ) ;
#28605=CARTESIAN_POINT ( 'NONE',  ( -11.98450388067348804, 210.9467285061362247, 66.65113791807856103 ) ) ;
#28606=CARTESIAN_POINT ( 'NONE',  ( 6.500168698208129925, 211.6636982574063381, 88.70113791807857240 ) ) ;
#28607=CARTESIAN_POINT ( 'NONE',  ( -3.044812012439970683, 197.4746971517856196, 43.89886208192142902 ) ) ;
#28611=CARTESIAN_POINT ( 'NONE',  ( 7.375838497908012492, 217.2372850707501186, 48.54886208192142050 ) ) ;
#28617=CARTESIAN_POINT ( 'NONE',  ( -8.000000000000008882, 207.0476921513413515, 45.50113791807857666 ) ) ;
#28619=CARTESIAN_POINT ( 'NONE',  ( -8.062137200540822946, 201.0835637161416400, 20.19886208192143684 ) ) ;
#28621=ORIENTED_EDGE ( 'NONE', *, *, #22607, .F. ) ;
#28624=CARTESIAN_POINT ( 'NONE',  ( 2.517493886309087436, 199.4062855549015865, 7.598862081921434530 ) ) ;
#28625=CARTESIAN_POINT ( 'NONE',  ( 0.05014649552810505201, 217.5146222423826714, 43.25113791807856956 ) ) ;
#28627=CARTESIAN_POINT ( 'NONE',  ( 6.139770520408368348, 198.4640165459539674, 29.45113791807856529 ) ) ;
#28628=CARTESIAN_POINT ( 'NONE',  ( -8.062137200540822946, 201.0835637161416400, 101.1988620819214475 ) ) ;
#28630=CARTESIAN_POINT ( 'NONE',  ( 8.000000000000008882, 207.0476921513415220, 90.99886208192144466 ) ) ;
#28634=CARTESIAN_POINT ( 'NONE',  ( 12.00000000000000711, 206.9523078486586485, 14.00113791807856600 ) ) ;
#28637=CARTESIAN_POINT ( 'NONE',  ( -3.135527875058821579, 197.5041725223112223, 56.90113791807857524 ) ) ;
#28643=CARTESIAN_POINT ( 'NONE',  ( 12.01549611932652972, 210.8513442034534933, 34.85113791807856387 ) ) ;
#28645=CARTESIAN_POINT ( 'NONE',  ( 8.118202686958138514, 201.1607312380088501, 10.29886208192143471 ) ) ;
#28648=CARTESIAN_POINT ( 'NONE',  ( -10.00000000000000711, 207.0476921513413515, 69.50113791807856956 ) ) ;
#28650=CARTESIAN_POINT ( 'NONE',  ( -4.984841277089891776, 213.7757310962905990, 35.94886208192144039 ) ) ;
#28654=CARTESIAN_POINT ( 'NONE',  ( -4.903702542908602524, 213.8346818373418898, 12.95113791807856707 ) ) ;
#28656=CARTESIAN_POINT ( 'NONE',  ( 3.662846001189864698, 218.4274158808046593, 99.39886208192146455 ) ) ;
#28661=CARTESIAN_POINT ( 'NONE',  ( -3.135527875058821579, 197.5041725223112223, 8.901137918078566358 ) ) ;
#28662=CARTESIAN_POINT ( 'NONE',  ( 3.135527875058981895, 197.5041725223112792, 76.59886208192142476 ) ) ;
#28665=CARTESIAN_POINT ( 'NONE',  ( 8.118202686958039038, 212.8392687619912635, 16.70113791807856529 ) ) ;
#28669=CARTESIAN_POINT ( 'NONE',  ( -10.01549611932653860, 203.7984951890123284, 96.35113791807853545 ) ) ;
#28671=CARTESIAN_POINT ( 'NONE',  ( -8.062137200540920645, 212.9164362838581894, 87.80113791807856671 ) ) ;
#28674=CARTESIAN_POINT ( 'NONE',  ( 9.680171189290716072, 214.0920067884432854, 99.69886208192144750 ) ) ;
#28679=CARTESIAN_POINT ( 'NONE',  ( 11.98450388067348271, 203.0532714938637753, 101.1511379180785895 ) ) ;
#28686=CARTESIAN_POINT ( 'NONE',  ( 9.984503880673420539, 210.2968891136705736, 87.84886208192142476 ) ) ;
#28687=CARTESIAN_POINT ( 'NONE',  ( -12.00000000000000711, 206.9523078486584780, 23.49886208192144110 ) ) ;
#28689=CARTESIAN_POINT ( 'NONE',  ( 0.05014649552810505201, 217.5146222423826714, 46.25113791807855534 ) ) ;
#28691=CARTESIAN_POINT ( 'NONE',  ( -4.903702542908436435, 200.1653181626580249, 8.048862081921434708 ) ) ;
#28696=CARTESIAN_POINT ( 'NONE',  ( -7.984503880673422316, 204.3529502787951628, 92.34886208192143897 ) ) ;
#28698=CARTESIAN_POINT ( 'NONE',  ( -2.426778023690262742, 214.6231898156240163, 28.10113791807856742 ) ) ;
#28704=CARTESIAN_POINT ( 'NONE',  ( -2.426778023690262742, 214.6231898156240163, 88.10113791807857808 ) ) ;
#28709=CARTESIAN_POINT ( 'NONE',  ( -2.426778023690076225, 199.3768101843759553, 67.89886208192143613 ) ) ;
#28716=CARTESIAN_POINT ( 'NONE',  ( 9.984503880673473830, 203.7031108863295401, 5.151137918078566358 ) ) ;
#28717=DIRECTION ( 'NONE',  ( 0.9366133782696128840, 0.000000000000000000, 0.3503646381220332229 ) ) ;
#28720=CARTESIAN_POINT ( 'NONE',  ( 3.753561863808689836, 218.3979405102790565, 67.40113791807856103 ) ) ;
#28722=CARTESIAN_POINT ( 'NONE',  ( 7.375838497908181246, 196.7627149292499666, 11.45113791807856529 ) ) ;
#28723=CARTESIAN_POINT ( 'NONE',  ( 9.984503880673473830, 203.7031108863295401, 92.15113791807854682 ) ) ;
#28725=CARTESIAN_POINT ( 'NONE',  ( 11.98450388067341876, 210.9467285061363953, 48.84886208192143897 ) ) ;
#28726=CARTESIAN_POINT ( 'NONE',  ( -6.139770520408224463, 198.4640165459539105, 62.04886208192143471 ) ) ;
#28727=CARTESIAN_POINT ( 'NONE',  ( 9.680171189290831535, 199.9079932115568852, 101.3011379180785951 ) ) ;
#28729=CARTESIAN_POINT ( 'NONE',  ( -9.984503880673473830, 210.2968891136704315, 15.65113791807856813 ) ) ;
#28730=CARTESIAN_POINT ( 'NONE',  ( -6.139770520408224463, 198.4640165459539389, 80.04886208192139918 ) ) ;
#28732=CARTESIAN_POINT ( 'NONE',  ( 7.375838497908012492, 217.2372850707501186, 81.54886208192144181 ) ) ;
#28734=CARTESIAN_POINT ( 'NONE',  ( 8.062137200540920645, 201.0835637161417822, 101.3011379180785809 ) ) ;
#28735=VERTEX_POINT ( 'NONE', #26732 ) ;
#28737=CARTESIAN_POINT ( 'NONE',  ( -6.500168698208244500, 211.6636982574061676, 65.79886208192144181 ) ) ;
#28747=CARTESIAN_POINT ( 'NONE',  ( 10.00000000000000711, 207.0476921513415220, 51.99886208192143755 ) ) ;
#28751=CARTESIAN_POINT ( 'NONE',  ( 4.984841277089891776, 200.2242689037093726, 31.44886208192143684 ) ) ;
#28752=CARTESIAN_POINT ( 'NONE',  ( -10.01549611932653860, 203.7984951890123284, 84.35113791807856387 ) ) ;
#28755=CARTESIAN_POINT ( 'NONE',  ( -9.984503880673473830, 210.2968891136704315, 57.65113791807858235 ) ) ;
#28757=CARTESIAN_POINT ( 'NONE',  ( 8.062137200540920645, 201.0835637161417822, 32.30113791807857382 ) ) ;
#28758=CARTESIAN_POINT ( 'NONE',  ( -6.500168698208129925, 202.3363017425936050, 12.20113791807856707 ) ) ;
#28762=CARTESIAN_POINT ( 'NONE',  ( 11.98450388067348271, 203.0532714938637753, 35.15113791807856103 ) ) ;
#28765=CARTESIAN_POINT ( 'NONE',  ( 3.044812012440130555, 197.4746971517856764, 83.60113791807857808 ) ) ;
#28766=CARTESIAN_POINT ( 'NONE',  ( 0.05014649552810506589, 217.5146222423826714, 55.25113791807857666 ) ) ;
#28768=CARTESIAN_POINT ( 'NONE',  ( 9.680171189290716072, 214.0920067884432854, 18.69886208192143684 ) ) ;
#28769=CARTESIAN_POINT ( 'NONE',  ( 10.00000000000000711, 207.0476921513415220, 24.99886208192143400 ) ) ;
#28771=CARTESIAN_POINT ( 'NONE',  ( -7.456977232089304408, 196.8216656703010301, 63.05113791807858092 ) ) ;
#28772=CARTESIAN_POINT ( 'NONE',  ( -2.426778023690262742, 214.6231898156240163, 91.10113791807859229 ) ) ;
#28773=CARTESIAN_POINT ( 'NONE',  ( -8.062137200540822946, 201.0835637161416400, 53.19886208192143329 ) ) ;
#28777=CARTESIAN_POINT ( 'NONE',  ( -9.680171189290716072, 199.9079932115567146, 56.19886208192144039 ) ) ;
#28778=ORIENTED_EDGE ( 'NONE', *, *, #20637, .F. ) ;
#28782=CARTESIAN_POINT ( 'NONE',  ( -3.135527875058982783, 216.4958274776886924, 54.09886208192143897 ) ) ;
#28784=CARTESIAN_POINT ( 'NONE',  ( -2.426778023690262742, 214.6231898156240163, 43.10113791807857808 ) ) ;
#28787=CARTESIAN_POINT ( 'NONE',  ( -8.062137200540822946, 201.0835637161416400, 23.19886208192143684 ) ) ;
#28794=CARTESIAN_POINT ( 'NONE',  ( 4.984841277089891776, 200.2242689037093726, 1.448862081921434841 ) ) ;
#28795=CARTESIAN_POINT ( 'NONE',  ( 9.984503880673470277, 203.7031108863295401, 38.15113791807856813 ) ) ;
#28796=CARTESIAN_POINT ( 'NONE',  ( 8.118202686958039038, 212.8392687619912635, 31.70113791807856884 ) ) ;
#28797=CARTESIAN_POINT ( 'NONE',  ( -8.118202686958138514, 212.8392687619910930, 101.7988620819214418 ) ) ;
#28799=CARTESIAN_POINT ( 'NONE',  ( -6.500168698208244500, 211.6636982574061676, 92.79886208192142760 ) ) ;
#28803=CARTESIAN_POINT ( 'NONE',  ( -3.662846001190052991, 218.4274158808045740, 13.10113791807856742 ) ) ;
#28807=CARTESIAN_POINT ( 'NONE',  ( -10.01549611932653860, 203.7984951890123284, 54.35113791807856387 ) ) ;
#28808=CARTESIAN_POINT ( 'NONE',  ( -3.044812012440131443, 216.5253028482142952, 31.10113791807856742 ) ) ;
#28813=CARTESIAN_POINT ( 'NONE',  ( -9.680171189290831535, 214.0920067884431148, 42.80113791807857382 ) ) ;
#28816=CARTESIAN_POINT ( 'NONE',  ( 3.044812012439969795, 216.5253028482143520, 21.39886208192143613 ) ) ;
#28819=CARTESIAN_POINT ( 'NONE',  ( -0.05014649552810635652, 196.4853777576173002, 74.75113791807858377 ) ) ;
#28823=CARTESIAN_POINT ( 'NONE',  ( -8.015496119326531499, 204.4483345814780364, 12.35113791807856565 ) ) ;
#28825=CARTESIAN_POINT ( 'NONE',  ( -9.680171189290716072, 199.9079932115567146, 101.1988620819214475 ) ) ;
#28830=CARTESIAN_POINT ( 'NONE',  ( -3.044812012440131443, 216.5253028482142952, 13.10113791807856742 ) ) ;
#28831=CARTESIAN_POINT ( 'NONE',  ( -8.062137200540822946, 201.0835637161416400, 77.19886208192143329 ) ) ;
#28834=CARTESIAN_POINT ( 'NONE',  ( 6.220909254589536808, 215.4770327129947702, 10.55113791807856138 ) ) ;
#28838=CARTESIAN_POINT ( 'NONE',  ( -6.139770520408369237, 215.5359834540460042, 96.95113791807857240 ) ) ;
#28840=CARTESIAN_POINT ( 'NONE',  ( 10.01549611932653860, 210.2015048109876716, 88.85113791807857808 ) ) ;
#28843=CARTESIAN_POINT ( 'NONE',  ( 9.736236675708031640, 199.9851607334238963, 94.29886208192142760 ) ) ;
#28849=CARTESIAN_POINT ( 'NONE',  ( -12.00000000000000711, 206.9523078486584780, 5.498862081921433997 ) ) ;
#28852=CARTESIAN_POINT ( 'NONE',  ( -6.139770520408224463, 198.4640165459539105, 95.04886208192144181 ) ) ;
#28853=CARTESIAN_POINT ( 'NONE',  ( 7.456977232089471386, 196.8216656703012006, 34.44886208192142618 ) ) ;
#28855=CARTESIAN_POINT ( 'NONE',  ( -0.05014649552810635652, 196.4853777576173002, 44.75113791807858377 ) ) ;
#28857=CARTESIAN_POINT ( 'NONE',  ( 8.000000000000008882, 207.0476921513415220, 0.9988620819214347746 ) ) ;
#28860=CARTESIAN_POINT ( 'NONE',  ( 8.000000000000008882, 207.0476921513415220, 93.99886208192144466 ) ) ;
#28861=CARTESIAN_POINT ( 'NONE',  ( 0.05014649552807626948, 215.4116977939061144, 28.25113791807856245 ) ) ;
#28867=CARTESIAN_POINT ( 'NONE',  ( -4.984841277089726574, 200.2242689037092305, 93.05113791807858092 ) ) ;
#28870=CARTESIAN_POINT ( 'NONE',  ( 0.05014649552828262524, 198.5883022060938572, 58.74886208192143755 ) ) ;
#28875=CARTESIAN_POINT ( 'NONE',  ( -8.062137200540920645, 212.9164362838581894, 12.80113791807856671 ) ) ;
#28881=CARTESIAN_POINT ( 'NONE',  ( -3.753561863808691168, 195.6020594897209435, 62.90113791807858945 ) ) ;
#28883=CARTESIAN_POINT ( 'NONE',  ( -8.118202686958039038, 201.1607312380087080, 90.20113791807857240 ) ) ;
#28887=CARTESIAN_POINT ( 'NONE',  ( 12.00000000000000711, 207.0476921513415220, 54.99886208192144466 ) ) ;
#28888=CARTESIAN_POINT ( 'NONE',  ( 10.01549611932659367, 203.7984951890124421, 70.14886208192142192 ) ) ;
#28889=CARTESIAN_POINT ( 'NONE',  ( -11.98450388067348804, 210.9467285061362247, 96.65113791807858945 ) ) ;
#28891=CARTESIAN_POINT ( 'NONE',  ( 6.139770520408368348, 198.4640165459539674, 11.45113791807856707 ) ) ;
#28892=CARTESIAN_POINT ( 'NONE',  ( 9.984503880673420539, 210.2968891136705167, 78.84886208192139634 ) ) ;
#28894=CARTESIAN_POINT ( 'NONE',  ( -3.044812012440131443, 216.5253028482142952, 97.10113791807857808 ) ) ;
#28897=CARTESIAN_POINT ( 'NONE',  ( -4.984841277089891776, 213.7757310962905990, 59.94886208192144039 ) ) ;
#28906=CARTESIAN_POINT ( 'NONE',  ( -8.000000000000008882, 207.0476921513413515, 60.50113791807857666 ) ) ;
#28910=CARTESIAN_POINT ( 'NONE',  ( 4.903702542908435547, 213.8346818373419751, 30.54886208192144181 ) ) ;
#28911=CARTESIAN_POINT ( 'NONE',  ( -6.139770520408369237, 215.5359834540460042, 81.95113791807854398 ) ) ;
#28913=CARTESIAN_POINT ( 'NONE',  ( -8.118202686958039038, 201.1607312380087080, 60.20113791807857240 ) ) ;
#28914=CARTESIAN_POINT ( 'NONE',  ( -6.220909254589537696, 198.5229672870051161, 27.05113791807856671 ) ) ;
#28915=CARTESIAN_POINT ( 'NONE',  ( 8.000000000000008882, 206.9523078486586485, 14.00113791807856600 ) ) ;
#28919=CARTESIAN_POINT ( 'NONE',  ( 3.662846001190051659, 195.5725841191953691, 35.60113791807855677 ) ) ;
#28921=CARTESIAN_POINT ( 'NONE',  ( -6.139770520408369237, 215.5359834540460042, 81.95113791807854398 ) ) ;
#28922=CARTESIAN_POINT ( 'NONE',  ( 0.05014649552810506589, 217.5146222423826714, 61.25113791807856956 ) ) ;
#28923=CARTESIAN_POINT ( 'NONE',  ( -12.00000000000000711, 206.9523078486584780, 20.49886208192143755 ) ) ;
#28924=CARTESIAN_POINT ( 'NONE',  ( 3.044812012439969795, 216.5253028482143520, 24.39886208192143613 ) ) ;
#28927=CARTESIAN_POINT ( 'NONE',  ( -3.662846001190052991, 218.4274158808045740, 67.10113791807857808 ) ) ;
#28928=CARTESIAN_POINT ( 'NONE',  ( -7.984503880673488041, 209.6470497212046098, 87.65113791807857524 ) ) ;
#28930=CARTESIAN_POINT ( 'NONE',  ( 3.044812012439969795, 216.5253028482143520, 54.39886208192143613 ) ) ;
#28934=CARTESIAN_POINT ( 'NONE',  ( -12.00000000000000711, 206.9523078486584780, 56.49886208192144466 ) ) ;
#28942=CARTESIAN_POINT ( 'NONE',  ( 2.426778023690261410, 199.3768101843759837, 41.60113791807857808 ) ) ;
#28946=CARTESIAN_POINT ( 'NONE',  ( 6.220909254589681581, 198.5229672870052582, 25.44886208192143684 ) ) ;
#28952=CARTESIAN_POINT ( 'NONE',  ( 4.984841277089891776, 200.2242689037093726, 10.44886208192143506 ) ) ;
#28953=CARTESIAN_POINT ( 'NONE',  ( 8.062137200540920645, 201.0835637161417822, 56.30113791807857382 ) ) ;
#28955=CARTESIAN_POINT ( 'NONE',  ( 6.139770520408368348, 198.4640165459539674, 23.45113791807856884 ) ) ;
#28958=CARTESIAN_POINT ( 'NONE',  ( -8.015496119326597224, 209.5516654185217362, 92.64886208192143613 ) ) ;
#28962=CARTESIAN_POINT ( 'NONE',  ( 11.98450388067348271, 203.0532714938637753, 11.15113791807856636 ) ) ;
#28966=CARTESIAN_POINT ( 'NONE',  ( 3.135527875058820690, 216.4958274776887492, 52.40113791807857524 ) ) ;
#28967=CARTESIAN_POINT ( 'NONE',  ( -9.984503880673475606, 210.2968891136704315, 33.65113791807856813 ) ) ;
#28969=CYLINDRICAL_SURFACE ( 'NONE', #11409, 0.9999999999999953371 ) ;
#28970=CARTESIAN_POINT ( 'NONE',  ( -0.05014649552828402690, 217.5146222423826714, 3.248862081921434442 ) ) ;
#28973=CARTESIAN_POINT ( 'NONE',  ( 11.98450388067348271, 203.0532714938637753, 35.15113791807856103 ) ) ;
#28975=CARTESIAN_POINT ( 'NONE',  ( 9.984503880673420539, 210.2968891136705167, 24.84886208192143897 ) ) ;
#28980=CARTESIAN_POINT ( 'NONE',  ( 10.01549611932653860, 210.2015048109876716, 76.85113791807857808 ) ) ;
#28987=CARTESIAN_POINT ( 'NONE',  ( 4.984841277089725686, 213.7757310962907411, 16.55113791807857027 ) ) ;
#28989=CARTESIAN_POINT ( 'NONE',  ( 7.456977232089471386, 196.8216656703012006, 97.44886208192143329 ) ) ;
#28994=CARTESIAN_POINT ( 'NONE',  ( -8.062137200540920645, 212.9164362838581894, 6.801137918078565825 ) ) ;
#28995=CARTESIAN_POINT ( 'NONE',  ( 0.05014649552828275708, 196.4853777576173002, 85.74886208192140202 ) ) ;
#28997=CARTESIAN_POINT ( 'NONE',  ( 0.05014649552810505201, 217.5146222423826714, 25.25113791807856245 ) ) ;
#29001=CARTESIAN_POINT ( 'NONE',  ( -3.044812012440131443, 216.5253028482142952, 100.1011379180785781 ) ) ;
#29003=CARTESIAN_POINT ( 'NONE',  ( 3.135527875058820690, 216.4958274776887492, 82.40113791807857524 ) ) ;
#29006=CARTESIAN_POINT ( 'NONE',  ( 9.736236675708031640, 199.9851607334238963, 97.29886208192142760 ) ) ;
#29012=AXIS2_PLACEMENT_3D ( 'NONE', #19474, #27808, #9584 ) ;
#29018=CARTESIAN_POINT ( 'NONE',  ( 3.135527875058981895, 197.5041725223112792, 94.59886208192143897 ) ) ;
#29019=CARTESIAN_POINT ( 'NONE',  ( 3.662846001189864698, 218.4274158808046593, 33.39886208192143613 ) ) ;
#29021=CARTESIAN_POINT ( 'NONE',  ( -10.00000000000000711, 207.0476921513413515, 42.50113791807856956 ) ) ;
#29023=CARTESIAN_POINT ( 'NONE',  ( -0.05014649552828365914, 215.4116977939061144, 3.248862081921435330 ) ) ;
#29027=CARTESIAN_POINT ( 'NONE',  ( -4.984841277089891776, 213.7757310962905990, 92.94886208192144750 ) ) ;
#29028=EDGE_CURVE ( 'NONE', #17153, #31012, #11319, .T. ) ;
#29030=CARTESIAN_POINT ( 'NONE',  ( -7.984503880673488041, 209.6470497212046098, 33.65113791807856813 ) ) ;
#29038=CARTESIAN_POINT ( 'NONE',  ( 6.444103211791042618, 202.2591342207267644, 86.30113791807858092 ) ) ;
#29041=CARTESIAN_POINT ( 'NONE',  ( -4.903702542908436435, 200.1653181626580249, 74.04886208192142760 ) ) ;
#29044=CARTESIAN_POINT ( 'NONE',  ( -10.01549611932653860, 203.7984951890123000, 9.351137918078569200 ) ) ;
#29048=CARTESIAN_POINT ( 'NONE',  ( 3.662846001190051659, 195.5725841191953691, 74.60113791807854966 ) ) ;
#29051=CARTESIAN_POINT ( 'NONE',  ( 3.135527875058820690, 216.4958274776887492, 94.40113791807857524 ) ) ;
#29054=CARTESIAN_POINT ( 'NONE',  ( -9.736236675708031640, 214.0148392665760753, 65.79886208192144181 ) ) ;
#29055=CARTESIAN_POINT ( 'NONE',  ( -8.062137200540822946, 201.0835637161416400, 65.19886208192143329 ) ) ;
#29057=CARTESIAN_POINT ( 'NONE',  ( -7.456977232089304408, 196.8216656703010301, 102.0511379180785809 ) ) ;
#29059=CARTESIAN_POINT ( 'NONE',  ( 8.118202686958039038, 212.8392687619912635, 16.70113791807856529 ) ) ;
#29061=CARTESIAN_POINT ( 'NONE',  ( 10.01549611932659545, 203.7984951890123853, 76.14886208192143613 ) ) ;
#29065=CARTESIAN_POINT ( 'NONE',  ( 8.015496119326595448, 204.4483345814782638, 58.14886208192145034 ) ) ;
#29074=CARTESIAN_POINT ( 'NONE',  ( -7.984503880673488041, 209.6470497212046098, 63.65113791807855392 ) ) ;
#29081=CARTESIAN_POINT ( 'NONE',  ( 2.426778023690075337, 214.6231898156240447, 48.39886208192144323 ) ) ;
#29082=CARTESIAN_POINT ( 'NONE',  ( -0.05014649552810635652, 196.4853777576173002, 80.75113791807854113 ) ) ;
#29084=CARTESIAN_POINT ( 'NONE',  ( -8.118202686958039038, 201.1607312380087080, 66.20113791807857240 ) ) ;
#29086=CARTESIAN_POINT ( 'NONE',  ( 0.05014649552807626948, 215.4116977939061144, 13.25113791807856423 ) ) ;
#29090=CARTESIAN_POINT ( 'NONE',  ( 7.375838497908181246, 196.7627149292499666, 47.45113791807857950 ) ) ;
#29092=CARTESIAN_POINT ( 'NONE',  ( -6.139770520408369237, 215.5359834540460042, 96.95113791807857240 ) ) ;
#29093=CARTESIAN_POINT ( 'NONE',  ( 0.05014649552810506589, 217.5146222423826714, 67.25113791807856956 ) ) ;
#29094=CARTESIAN_POINT ( 'NONE',  ( -0.05014649552828442242, 219.6175466908591716, 24.24886208192144110 ) ) ;
#29095=CARTESIAN_POINT ( 'NONE',  ( -10.01549611932659545, 210.2015048109875011, 38.64886208192142902 ) ) ;
#29097=CARTESIAN_POINT ( 'NONE',  ( -9.680171189290831535, 214.0920067884431148, 78.80113791807858092 ) ) ;
#29098=CARTESIAN_POINT ( 'NONE',  ( -2.517493886308901807, 199.4062855549015012, 83.90113791807856103 ) ) ;
#29100=CARTESIAN_POINT ( 'NONE',  ( -6.139770520408224463, 198.4640165459539389, 50.04886208192143471 ) ) ;
#29103=CARTESIAN_POINT ( 'NONE',  ( 7.456977232089471386, 196.8216656703012006, 49.44886208192144039 ) ) ;
#29109=CARTESIAN_POINT ( 'NONE',  ( 4.984841277089725686, 213.7757310962907411, 55.55113791807858092 ) ) ;
#29111=CARTESIAN_POINT ( 'NONE',  ( -10.01549611932659722, 210.2015048109875011, 29.64886208192143968 ) ) ;
#29117=CARTESIAN_POINT ( 'NONE',  ( -6.500168698208244500, 211.6636982574061676, 8.798862081921434708 ) ) ;
#29118=CARTESIAN_POINT ( 'NONE',  ( 10.00000000000000711, 206.9523078486586201, 53.00113791807857666 ) ) ;
#29121=CARTESIAN_POINT ( 'NONE',  ( -10.00000000000000711, 207.0476921513413515, 33.50113791807856956 ) ) ;
#29124=CARTESIAN_POINT ( 'NONE',  ( -7.984503880673422316, 204.3529502787951628, 89.34886208192143897 ) ) ;
#29127=CARTESIAN_POINT ( 'NONE',  ( 0.05014649552807549926, 219.6175466908591716, 13.25113791807856423 ) ) ;
#29131=CARTESIAN_POINT ( 'NONE',  ( 8.062137200540920645, 201.0835637161417822, 62.30113791807858092 ) ) ;
#29132=CARTESIAN_POINT ( 'NONE',  ( -10.00000000000000711, 207.0476921513413515, 30.50113791807856600 ) ) ;
#29134=DIRECTION ( 'NONE',  ( 0.000000000000000000, -0.9988620819214357738, -0.04769215134144155765 ) ) ;
#29135=CARTESIAN_POINT ( 'NONE',  ( -3.044812012439970683, 197.4746971517856196, 4.898862081921434353 ) ) ;
#29138=CARTESIAN_POINT ( 'NONE',  ( -12.00000000000000711, 207.0476921513413515, 39.50113791807856245 ) ) ;
#29141=CARTESIAN_POINT ( 'NONE',  ( -10.01549611932659722, 210.2015048109875011, 20.64886208192143613 ) ) ;
#29144=CARTESIAN_POINT ( 'NONE',  ( 8.118202686958039038, 212.8392687619912635, 76.70113791807857240 ) ) ;
#29149=CARTESIAN_POINT ( 'NONE',  ( 0.05014649552807626948, 215.4116977939061144, 10.25113791807856600 ) ) ;
#29151=CARTESIAN_POINT ( 'NONE',  ( 11.98450388067341876, 210.9467285061363953, 102.8488620819214390 ) ) ;
#29157=CARTESIAN_POINT ( 'NONE',  ( -10.01549611932659722, 210.2015048109875011, 80.64886208192143613 ) ) ;
#29159=CARTESIAN_POINT ( 'NONE',  ( 10.01549611932653860, 210.2015048109876716, 19.85113791807856387 ) ) ;
#29163=CARTESIAN_POINT ( 'NONE',  ( -11.98450388067341876, 203.0532714938636047, 77.34886208192143897 ) ) ;
#29168=CARTESIAN_POINT ( 'NONE',  ( 6.220909254589536808, 215.4770327129947702, 85.55113791807858092 ) ) ;
#29174=CARTESIAN_POINT ( 'NONE',  ( -11.98450388067341876, 203.0532714938636047, 95.34886208192143897 ) ) ;
#29176=VERTEX_POINT ( 'NONE', #23316 ) ;
#29182=CARTESIAN_POINT ( 'NONE',  ( -3.044812012439970683, 197.4746971517856196, 94.89886208192143613 ) ) ;
#29183=CARTESIAN_POINT ( 'NONE',  ( -7.456977232089471386, 217.1783343296987709, 29.94886208192143684 ) ) ;
#29185=CARTESIAN_POINT ( 'NONE',  ( -3.135527875058821579, 197.5041725223112223, 47.90113791807857524 ) ) ;
#29188=CARTESIAN_POINT ( 'NONE',  ( 6.220909254589681581, 198.5229672870052582, 103.4488620819214049 ) ) ;
#29193=CARTESIAN_POINT ( 'NONE',  ( 4.984841277089891776, 200.2242689037093726, 88.44886208192144750 ) ) ;
#29194=CARTESIAN_POINT ( 'NONE',  ( -4.984841277089726574, 200.2242689037092305, 27.05113791807857027 ) ) ;
#29201=CARTESIAN_POINT ( 'NONE',  ( -4.984841277089726574, 200.2242689037092305, 102.0511379180785809 ) ) ;
#29204=CARTESIAN_POINT ( 'NONE',  ( 0.05014649552828262524, 198.5883022060938572, 70.74886208192144466 ) ) ;
#29209=CARTESIAN_POINT ( 'NONE',  ( 9.984503880673473830, 203.7031108863295401, 8.151137918078566358 ) ) ;
#29213=CARTESIAN_POINT ( 'NONE',  ( -3.662846001190052991, 218.4274158808045740, 73.10113791807857808 ) ) ;
#29215=CARTESIAN_POINT ( 'NONE',  ( -6.139770520408368348, 215.5359834540460042, 99.95113791807855819 ) ) ;
#29218=CARTESIAN_POINT ( 'NONE',  ( -12.01549611932659722, 210.8513442034533227, 101.6488620819214361 ) ) ;
#29219=CARTESIAN_POINT ( 'NONE',  ( 12.01549611932659367, 203.1486557965466773, 64.14886208192143613 ) ) ;
#29220=CARTESIAN_POINT ( 'NONE',  ( 8.118202686958138514, 201.1607312380088501, 67.29886208192144181 ) ) ;
#29221=CARTESIAN_POINT ( 'NONE',  ( -0.05014649552807705357, 194.3824533091408000, 101.7511379180785696 ) ) ;
#29223=CARTESIAN_POINT ( 'NONE',  ( 0.05014649552810505201, 217.5146222423826714, 25.25113791807856245 ) ) ;
#29224=CARTESIAN_POINT ( 'NONE',  ( -10.00000000000000711, 206.9523078486584495, 83.49886208192143044 ) ) ;
#29226=CARTESIAN_POINT ( 'NONE',  ( 8.062137200540920645, 201.0835637161417822, 98.30113791807858092 ) ) ;
#29229=CARTESIAN_POINT ( 'NONE',  ( 4.903702542908435547, 213.8346818373419751, 57.54886208192142760 ) ) ;
#29239=CARTESIAN_POINT ( 'NONE',  ( -8.000000000000008882, 207.0476921513413515, 69.50113791807856956 ) ) ;
#29245=CARTESIAN_POINT ( 'NONE',  ( 8.000000000000008882, 207.0476921513415220, 39.99886208192145176 ) ) ;
#29246=CARTESIAN_POINT ( 'NONE',  ( -3.044812012440131443, 216.5253028482142952, 82.10113791807857808 ) ) ;
#29247=CARTESIAN_POINT ( 'NONE',  ( 3.044812012440130555, 197.4746971517856764, 65.60113791807857808 ) ) ;
#29249=CARTESIAN_POINT ( 'NONE',  ( -4.984841277089726574, 200.2242689037092305, 24.05113791807857027 ) ) ;
#29253=CARTESIAN_POINT ( 'NONE',  ( 7.456977232089302632, 217.1783343296989131, 49.55113791807856671 ) ) ;
#29255=CARTESIAN_POINT ( 'NONE',  ( -8.118202686958039038, 201.1607312380087080, 99.20113791807858661 ) ) ;
#29257=CARTESIAN_POINT ( 'NONE',  ( 6.220909254589536808, 215.4770327129947987, 70.55113791807856671 ) ) ;
#29259=CARTESIAN_POINT ( 'NONE',  ( -9.736236675708031640, 214.0148392665760753, 32.79886208192143471 ) ) ;
#29260=CARTESIAN_POINT ( 'NONE',  ( -10.01549611932659545, 210.2015048109875011, 35.64886208192142902 ) ) ;
#29262=CARTESIAN_POINT ( 'NONE',  ( 3.662846001190051659, 195.5725841191953691, 74.60113791807854966 ) ) ;
#29263=CARTESIAN_POINT ( 'NONE',  ( -7.984503880673488041, 209.6470497212046098, 90.65113791807857524 ) ) ;
#29264=CARTESIAN_POINT ( 'NONE',  ( -8.062137200540822946, 201.0835637161416400, 47.19886208192143329 ) ) ;
#29268=CARTESIAN_POINT ( 'NONE',  ( -7.375838497908014268, 196.7627149292498530, 62.04886208192144181 ) ) ;
#29270=CARTESIAN_POINT ( 'NONE',  ( 8.000000000000008882, 207.0476921513415220, 33.99886208192143755 ) ) ;
#29275=CARTESIAN_POINT ( 'NONE',  ( -2.517493886308901807, 199.4062855549015012, 53.90113791807858235 ) ) ;
#29279=CARTESIAN_POINT ( 'NONE',  ( 3.135527875058981895, 197.5041725223112792, 28.59886208192143897 ) ) ;
#29284=CARTESIAN_POINT ( 'NONE',  ( -4.903702542908436435, 200.1653181626580249, 17.04886208192143471 ) ) ;
#29285=CARTESIAN_POINT ( 'NONE',  ( -3.135527875058821579, 197.5041725223112223, 53.90113791807857524 ) ) ;
#29287=CARTESIAN_POINT ( 'NONE',  ( 6.139770520408368348, 198.4640165459539674, 32.45113791807856529 ) ) ;
#29291=CARTESIAN_POINT ( 'NONE',  ( 6.500168698208244500, 202.3363017425938324, 97.29886208192142760 ) ) ;
#29295=CARTESIAN_POINT ( 'NONE',  ( -12.01549611932652972, 203.1486557965464499, 18.35113791807856387 ) ) ;
#29298=CARTESIAN_POINT ( 'NONE',  ( 6.139770520408368348, 198.4640165459539674, 65.45113791807857240 ) ) ;
#29300=CARTESIAN_POINT ( 'NONE',  ( 3.044812012440130555, 197.4746971517856764, 35.60113791807857098 ) ) ;
#29302=FACE_OUTER_BOUND ( 'NONE', #21133, .T. ) ;
#29303=CARTESIAN_POINT ( 'NONE',  ( -8.062137200540822946, 201.0835637161416400, 14.19886208192143684 ) ) ;
#29306=CARTESIAN_POINT ( 'NONE',  ( -9.736236675707914401, 199.9851607334237542, 48.20113791807858661 ) ) ;
#29308=FACE_OUTER_BOUND ( 'NONE', #23023, .T. ) ;
#29309=CARTESIAN_POINT ( 'NONE',  ( 9.984503880673420539, 210.2968891136705167, 18.84886208192143542 ) ) ;
#29315=CARTESIAN_POINT ( 'NONE',  ( -9.984503880673473830, 210.2968891136704315, 78.65113791807854682 ) ) ;
#29321=CARTESIAN_POINT ( 'NONE',  ( 8.000000000000008882, 206.9523078486586485, 20.00113791807856956 ) ) ;
#29324=CARTESIAN_POINT ( 'NONE',  ( 3.135527875058981895, 197.5041725223112792, 4.598862081921434530 ) ) ;
#29331=AXIS2_PLACEMENT_3D ( 'NONE', #4328, #16764, #14712 ) ;
#29332=CARTESIAN_POINT ( 'NONE',  ( 3.135527875058981895, 197.5041725223112792, 91.59886208192143897 ) ) ;
#29335=CARTESIAN_POINT ( 'NONE',  ( 10.01549611932653860, 210.2015048109876716, 22.85113791807856742 ) ) ;
#29337=CARTESIAN_POINT ( 'NONE',  ( 12.01549611932659367, 203.1486557965466773, 76.14886208192143613 ) ) ;
#29342=CARTESIAN_POINT ( 'NONE',  ( 8.062137200540920645, 201.0835637161417822, 98.30113791807858092 ) ) ;
#29345=CARTESIAN_POINT ( 'NONE',  ( -9.984503880673473830, 210.2968891136704315, 33.65113791807856813 ) ) ;
#29350=CARTESIAN_POINT ( 'NONE',  ( 9.680171189290831535, 199.9079932115568852, 23.30113791807857027 ) ) ;
#29353=ORIENTED_EDGE ( 'NONE', *, *, #5342, .T. ) ;
#29354=CARTESIAN_POINT ( 'NONE',  ( -0.05014649552828402690, 217.5146222423826714, 93.24886208192143044 ) ) ;
#29355=CARTESIAN_POINT ( 'NONE',  ( 12.00000000000000711, 207.0476921513415220, 33.99886208192143044 ) ) ;
#29358=CARTESIAN_POINT ( 'NONE',  ( 9.984503880673470277, 203.7031108863295401, 47.15113791807857524 ) ) ;
#29360=CARTESIAN_POINT ( 'NONE',  ( -4.903702542908436435, 200.1653181626580249, 11.04886208192143648 ) ) ;
#29362=EDGE_CURVE ( 'NONE', #25118, #860, #3172, .T. ) ;
#29365=CARTESIAN_POINT ( 'NONE',  ( -7.984503880673422316, 204.3529502787951628, 101.3488620819214390 ) ) ;
#29366=ADVANCED_FACE ( 'NONE', ( #21575 ), #33113, .T. ) ;
#29367=CARTESIAN_POINT ( 'NONE',  ( -8.015496119326531499, 204.4483345814780364, 39.35113791807857098 ) ) ;
#29371=CARTESIAN_POINT ( 'NONE',  ( -9.984503880673420539, 203.7031108863293980, 53.34886208192143897 ) ) ;
#29374=CARTESIAN_POINT ( 'NONE',  ( 4.984841277089725686, 213.7757310962907411, 94.55113791807855250 ) ) ;
#29377=CARTESIAN_POINT ( 'NONE',  ( 8.000000000000008882, 207.0476921513415220, 72.99886208192144466 ) ) ;
#29380=CARTESIAN_POINT ( 'NONE',  ( -3.044812012440131443, 216.5253028482142952, 13.10113791807856742 ) ) ;
#29384=CARTESIAN_POINT ( 'NONE',  ( -0.05014649552807705357, 194.3824533091408000, 74.75113791807856956 ) ) ;
#29385=CARTESIAN_POINT ( 'NONE',  ( 6.139770520408367460, 198.4640165459539389, 101.4511379180785866 ) ) ;
#29389=CARTESIAN_POINT ( 'NONE',  ( -7.375838497908014268, 196.7627149292498530, 104.0488620819214560 ) ) ;
#29390=CARTESIAN_POINT ( 'NONE',  ( -0.05014649552828442242, 219.6175466908591716, 57.24886208192144466 ) ) ;
#29391=CARTESIAN_POINT ( 'NONE',  ( -8.062137200540822946, 201.0835637161416400, 68.19886208192144750 ) ) ;
#29392=CARTESIAN_POINT ( 'NONE',  ( -0.05014649552828442242, 219.6175466908591716, 6.248862081921433997 ) ) ;
#29394=CARTESIAN_POINT ( 'NONE',  ( -3.044812012440131443, 216.5253028482142952, 22.10113791807856742 ) ) ;
#29395=CARTESIAN_POINT ( 'NONE',  ( 6.139770520408223575, 215.5359834540460611, 84.54886208192141339 ) ) ;
#29400=CARTESIAN_POINT ( 'NONE',  ( -0.05014649552828365914, 215.4116977939061144, 63.24886208192142334 ) ) ;
#29406=CARTESIAN_POINT ( 'NONE',  ( 4.984841277089725686, 213.7757310962907411, 64.55113791807856671 ) ) ;
#29407=FILL_AREA_STYLE_COLOUR ( '', #16754 ) ;
#29410=CARTESIAN_POINT ( 'NONE',  ( 4.984841277089891776, 200.2242689037093726, 43.44886208192144039 ) ) ;
#29411=CARTESIAN_POINT ( 'NONE',  ( -10.01549611932653860, 203.7984951890123284, 81.35113791807857808 ) ) ;
#29412=CARTESIAN_POINT ( 'NONE',  ( -6.139770520408369237, 215.5359834540460042, 69.95113791807857240 ) ) ;
#29414=CARTESIAN_POINT ( 'NONE',  ( -2.426778023690262742, 214.6231898156240163, 22.10113791807856742 ) ) ;
#29418=CARTESIAN_POINT ( 'NONE',  ( 11.98450388067348271, 203.0532714938637753, 44.15113791807856813 ) ) ;
#29420=CARTESIAN_POINT ( 'NONE',  ( 0.05014649552810505201, 217.5146222423826714, 97.25113791807854113 ) ) ;
#29422=CARTESIAN_POINT ( 'NONE',  ( -6.220909254589537696, 198.5229672870051445, 72.05113791807855250 ) ) ;
#29423=CARTESIAN_POINT ( 'NONE',  ( -11.98450388067341876, 203.0532714938636047, 35.34886208192142476 ) ) ;
#29424=CARTESIAN_POINT ( 'NONE',  ( 3.135527875058981895, 197.5041725223112792, 34.59886208192143897 ) ) ;
#29426=CARTESIAN_POINT ( 'NONE',  ( -12.01549611932652972, 203.1486557965464499, 78.35113791807857808 ) ) ;
#29427=CARTESIAN_POINT ( 'NONE',  ( -6.444103211791042618, 211.7408657792732356, 99.80113791807858092 ) ) ;
#29428=CARTESIAN_POINT ( 'NONE',  ( 10.00000000000000711, 207.0476921513415220, 48.99886208192143044 ) ) ;
#29431=CARTESIAN_POINT ( 'NONE',  ( 12.00000000000000711, 207.0476921513415220, 57.99886208192143044 ) ) ;
#29434=CARTESIAN_POINT ( 'NONE',  ( -6.500168698208244500, 211.6636982574061676, 29.79886208192143826 ) ) ;
#29439=CARTESIAN_POINT ( 'NONE',  ( -4.903702542908602524, 213.8346818373418898, 51.95113791807857240 ) ) ;
#29442=CARTESIAN_POINT ( 'NONE',  ( 10.01549611932659545, 203.7984951890123853, 34.14886208192143613 ) ) ;
#29448=CARTESIAN_POINT ( 'NONE',  ( -8.000000000000008882, 206.9523078486584780, 17.49886208192143400 ) ) ;
#29449=CARTESIAN_POINT ( 'NONE',  ( 9.984503880673470277, 203.7031108863295401, 56.15113791807856103 ) ) ;
#29451=CARTESIAN_POINT ( 'NONE',  ( -9.984503880673473830, 210.2968891136704315, 33.65113791807856813 ) ) ;
#29454=CARTESIAN_POINT ( 'NONE',  ( -2.517493886309087880, 214.5937144450984135, 102.0988620819214532 ) ) ;
#29458=CARTESIAN_POINT ( 'NONE',  ( -7.375838497908182134, 217.2372850707499765, 21.95113791807856884 ) ) ;
#29461=CARTESIAN_POINT ( 'NONE',  ( 3.044812012440130555, 197.4746971517856764, 65.60113791807857808 ) ) ;
#29462=CARTESIAN_POINT ( 'NONE',  ( 6.220909254589536808, 215.4770327129947987, 37.55113791807856671 ) ) ;
#29465=CARTESIAN_POINT ( 'NONE',  ( -11.98450388067341876, 203.0532714938636047, 5.348862081921434530 ) ) ;
#29466=CARTESIAN_POINT ( 'NONE',  ( 8.062137200540822946, 212.9164362838583315, 6.698862081921435063 ) ) ;
#29469=CARTESIAN_POINT ( 'NONE',  ( -11.98450388067348804, 210.9467285061362247, 48.65113791807857524 ) ) ;
#29471=CARTESIAN_POINT ( 'NONE',  ( 8.000000000000008882, 206.9523078486586485, 68.00113791807856956 ) ) ;
#29473=CARTESIAN_POINT ( 'NONE',  ( -6.139770520408224463, 198.4640165459539389, 20.04886208192142760 ) ) ;
#29475=CARTESIAN_POINT ( 'NONE',  ( 0.05014649552810505201, 217.5146222423826714, 85.25113791807854113 ) ) ;
#29480=CARTESIAN_POINT ( 'NONE',  ( 2.426778023690261410, 199.3768101843759837, 20.60113791807856742 ) ) ;
#29483=CARTESIAN_POINT ( 'NONE',  ( 9.984503880673420539, 210.2968891136705167, 3.848862081921433642 ) ) ;
#29492=CARTESIAN_POINT ( 'NONE',  ( -0.05014649552828403384, 217.5146222423826714, 90.24886208192141623 ) ) ;
#29494=CARTESIAN_POINT ( 'NONE',  ( -9.984503880673473830, 210.2968891136704315, 18.65113791807856813 ) ) ;
#29496=CARTESIAN_POINT ( 'NONE',  ( 11.98450388067341876, 210.9467285061363953, 81.84886208192142476 ) ) ;
#29501=CARTESIAN_POINT ( 'NONE',  ( 3.044812012440130555, 197.4746971517856764, 92.60113791807857808 ) ) ;
#29504=CARTESIAN_POINT ( 'NONE',  ( 10.01549611932653860, 210.2015048109876716, 37.85113791807854966 ) ) ;
#29510=CARTESIAN_POINT ( 'NONE',  ( -0.05014649552807705357, 194.3824533091408000, 17.75113791807856956 ) ) ;
#29516=CARTESIAN_POINT ( 'NONE',  ( 3.753561863808876797, 195.6020594897209719, 28.59886208192143897 ) ) ;
#29518=CARTESIAN_POINT ( 'NONE',  ( -3.135527875058821579, 197.5041725223112223, 53.90113791807857524 ) ) ;
#29522=CARTESIAN_POINT ( 'NONE',  ( -7.984503880673422316, 204.3529502787951628, 14.34886208192143364 ) ) ;
#29526=CARTESIAN_POINT ( 'NONE',  ( -6.444103211790928043, 202.2591342207265939, 101.1988620819214475 ) ) ;
#29528=CARTESIAN_POINT ( 'NONE',  ( 6.500168698208129925, 211.6636982574063381, 37.70113791807857240 ) ) ;
#29533=CARTESIAN_POINT ( 'NONE',  ( 8.118202686958138514, 201.1607312380088501, 61.29886208192143471 ) ) ;
#29536=CARTESIAN_POINT ( 'NONE',  ( 2.517493886308900919, 214.5937144450984420, 94.40113791807857524 ) ) ;
#29539=CARTESIAN_POINT ( 'NONE',  ( 6.444103211790928043, 211.7408657792734061, 75.69886208192143329 ) ) ;
#29545=CARTESIAN_POINT ( 'NONE',  ( 10.00000000000000711, 206.9523078486586201, 14.00113791807856600 ) ) ;
#29549=CARTESIAN_POINT ( 'NONE',  ( -0.05014649552807705357, 194.3824533091408000, 77.75113791807856956 ) ) ;
#29551=CARTESIAN_POINT ( 'NONE',  ( -6.220909254589537696, 198.5229672870051445, 102.0511379180785525 ) ) ;
#29554=CARTESIAN_POINT ( 'NONE',  ( 3.135527875058981895, 197.5041725223112792, 4.598862081921434530 ) ) ;
#29555=CARTESIAN_POINT ( 'NONE',  ( 9.680171189290716072, 214.0920067884432854, 63.69886208192144039 ) ) ;
#29557=CARTESIAN_POINT ( 'NONE',  ( 10.01549611932659367, 203.7984951890124421, 64.14886208192143613 ) ) ;
#29558=CARTESIAN_POINT ( 'NONE',  ( 7.456977232089471386, 196.8216656703012006, 1.448862081921433953 ) ) ;
#29560=CARTESIAN_POINT ( 'NONE',  ( 0.05014649552810505201, 217.5146222423826714, 19.25113791807856600 ) ) ;
#29562=CARTESIAN_POINT ( 'NONE',  ( 6.220909254589681581, 198.5229672870052582, 85.44886208192140487 ) ) ;
#29568=CARTESIAN_POINT ( 'NONE',  ( -2.426778023690076225, 199.3768101843759553, 73.89886208192143613 ) ) ;
#29576=CARTESIAN_POINT ( 'NONE',  ( 8.000000000000008882, 206.9523078486586485, 68.00113791807856956 ) ) ;
#29578=FACE_OUTER_BOUND ( 'NONE', #26537, .T. ) ;
#29581=CARTESIAN_POINT ( 'NONE',  ( -8.015496119326597224, 209.5516654185217362, 41.64886208192143613 ) ) ;
#29582=CARTESIAN_POINT ( 'NONE',  ( -9.984503880673473830, 210.2968891136704315, 93.65113791807857524 ) ) ;
#29583=EDGE_CURVE ( 'NONE', #16076, #24063, #32008, .T. ) ;
#29584=CARTESIAN_POINT ( 'NONE',  ( 10.01549611932653860, 210.2015048109876716, 61.85113791807857098 ) ) ;
#29587=CARTESIAN_POINT ( 'NONE',  ( -6.500168698208129925, 202.3363017425936050, 21.20113791807856529 ) ) ;
#29592=CARTESIAN_POINT ( 'NONE',  ( 3.662846001190051659, 195.5725841191953691, 50.60113791807857808 ) ) ;
#29595=CARTESIAN_POINT ( 'NONE',  ( 8.118202686958039038, 212.8392687619912635, 91.70113791807857240 ) ) ;
#29597=CARTESIAN_POINT ( 'NONE',  ( 6.139770520408367460, 198.4640165459539389, 65.45113791807857240 ) ) ;
#29598=CARTESIAN_POINT ( 'NONE',  ( -7.375838497908014268, 196.7627149292498530, 35.04886208192143471 ) ) ;
#29599=CARTESIAN_POINT ( 'NONE',  ( -8.062137200540822946, 201.0835637161416400, 35.19886208192143329 ) ) ;
#29601=CARTESIAN_POINT ( 'NONE',  ( 11.98450388067348271, 203.0532714938637753, 77.15113791807857524 ) ) ;
#29602=CARTESIAN_POINT ( 'NONE',  ( -7.949154985843430055, 215.5765611960900117, 102.9933096652613642 ) ) ;
#29604=CARTESIAN_POINT ( 'NONE',  ( 3.044812012439969795, 216.5253028482143520, 57.39886208192143613 ) ) ;
#29607=CARTESIAN_POINT ( 'NONE',  ( 3.662846001189864698, 218.4274158808046593, 63.39886208192144323 ) ) ;
#29611=CARTESIAN_POINT ( 'NONE',  ( 7.984503880673422316, 209.6470497212048372, 42.84886208192143897 ) ) ;
#29615=DIRECTION ( 'NONE',  ( -0.2649168722799616349, 0.9642688156137669830, -0.002168413296787739895 ) ) ;
#29616=CARTESIAN_POINT ( 'NONE',  ( 2.517493886308900919, 214.5937144450984420, 49.40113791807856813 ) ) ;
#29618=CARTESIAN_POINT ( 'NONE',  ( 0.05014649552828275708, 196.4853777576173002, 37.74886208192143755 ) ) ;
#29624=CARTESIAN_POINT ( 'NONE',  ( 2.517493886309087436, 199.4062855549015865, 13.59886208192143719 ) ) ;
#29625=CARTESIAN_POINT ( 'NONE',  ( -3.044812012440131443, 216.5253028482142952, 52.10113791807857808 ) ) ;
#29626=CARTESIAN_POINT ( 'NONE',  ( -3.135527875058821579, 197.5041725223112223, 32.90113791807857524 ) ) ;
#29630=CARTESIAN_POINT ( 'NONE',  ( -7.984503880673422316, 204.3529502787951628, 98.34886208192145318 ) ) ;
#29634=CARTESIAN_POINT ( 'NONE',  ( 7.456977232089302632, 217.1783343296989131, 22.55113791807857027 ) ) ;
#29636=CARTESIAN_POINT ( 'NONE',  ( -10.00000000000000711, 207.0476921513413515, 69.50113791807856956 ) ) ;
#29637=CARTESIAN_POINT ( 'NONE',  ( 3.135527875058820690, 216.4958274776887492, 43.40113791807856813 ) ) ;
#29640=CARTESIAN_POINT ( 'NONE',  ( 7.375838497908181246, 196.7627149292499666, 101.4511379180785866 ) ) ;
#29641=CARTESIAN_POINT ( 'NONE',  ( 8.118202686958138514, 201.1607312380088501, 7.298862081921435596 ) ) ;
#29644=CARTESIAN_POINT ( 'NONE',  ( 9.736236675707914401, 214.0148392665762458, 49.70113791807856529 ) ) ;
#29645=CARTESIAN_POINT ( 'NONE',  ( 8.000000000000008882, 206.9523078486586485, 71.00113791807856956 ) ) ;
#29646=CARTESIAN_POINT ( 'NONE',  ( 4.931287292257855448, 207.3577873115561943, -9.395021131069748677 ) ) ;
#29647=CARTESIAN_POINT ( 'NONE',  ( 10.01549611932659545, 203.7984951890123853, 34.14886208192143613 ) ) ;
#29650=CARTESIAN_POINT ( 'NONE',  ( 8.062137200540920645, 201.0835637161417822, 77.30113791807858092 ) ) ;
#29655=CARTESIAN_POINT ( 'NONE',  ( 8.015496119326531499, 209.5516654185219636, 22.85113791807856742 ) ) ;
#29657=CARTESIAN_POINT ( 'NONE',  ( -10.00000000000000711, 206.9523078486584495, 5.498862081921434886 ) ) ;
#29661=CARTESIAN_POINT ( 'NONE',  ( -2.517493886308901807, 199.4062855549015012, 50.90113791807858235 ) ) ;
#29664=CARTESIAN_POINT ( 'NONE',  ( 3.044812012439969795, 216.5253028482143520, 90.39886208192143613 ) ) ;
#29666=CARTESIAN_POINT ( 'NONE',  ( -6.139770520408369237, 215.5359834540460042, 18.95113791807856884 ) ) ;
#29668=CARTESIAN_POINT ( 'NONE',  ( -3.753561863808878130, 218.3979405102790281, 81.09886208192143897 ) ) ;
#29672=CARTESIAN_POINT ( 'NONE',  ( -6.220909254589537696, 198.5229672870051161, 96.05113791807858092 ) ) ;
#29675=CARTESIAN_POINT ( 'NONE',  ( -6.139770520408369237, 215.5359834540460042, 33.95113791807855108 ) ) ;
#29680=CARTESIAN_POINT ( 'NONE',  ( 12.01549611932652972, 210.8513442034534933, 19.85113791807856387 ) ) ;
#29685=CARTESIAN_POINT ( 'NONE',  ( 3.753561863808876797, 195.6020594897209719, 46.59886208192143187 ) ) ;
#29687=CARTESIAN_POINT ( 'NONE',  ( -3.044812012440131443, 216.5253028482142952, 52.10113791807857808 ) ) ;
#29689=CARTESIAN_POINT ( 'NONE',  ( -6.500168698208244500, 211.6636982574061676, 17.79886208192143471 ) ) ;
#29692=CARTESIAN_POINT ( 'NONE',  ( -2.426778023690076225, 199.3768101843759553, 97.89886208192146455 ) ) ;
#29694=CARTESIAN_POINT ( 'NONE',  ( 6.500168698208129925, 211.6636982574063381, 43.70113791807857240 ) ) ;
#29695=CARTESIAN_POINT ( 'NONE',  ( 9.379977934355910207, 208.8253170565643870, -1.014254689207407356 ) ) ;
#29698=CARTESIAN_POINT ( 'NONE',  ( 10.01549611932659545, 203.7984951890123853, 64.14886208192145034 ) ) ;
#29701=CARTESIAN_POINT ( 'NONE',  ( 2.517493886308900919, 214.5937144450984420, 97.40113791807858945 ) ) ;
#29704=CARTESIAN_POINT ( 'NONE',  ( -7.984503880673422316, 204.3529502787951628, 77.34886208192143897 ) ) ;
#29709=CARTESIAN_POINT ( 'NONE',  ( 9.984503880673473830, 203.7031108863295401, 23.15113791807856813 ) ) ;
#29713=CARTESIAN_POINT ( 'NONE',  ( -12.00000000000000711, 207.0476921513413515, 81.50113791807856956 ) ) ;
#29714=CARTESIAN_POINT ( 'NONE',  ( 6.139770520408367460, 198.4640165459539389, 95.45113791807855819 ) ) ;
#29719=CARTESIAN_POINT ( 'NONE',  ( -12.05084501415679199, 219.7456114157811271, 104.9910338291041114 ) ) ;
#29720=CARTESIAN_POINT ( 'NONE',  ( -11.98450388067341876, 203.0532714938636047, 62.34886208192143187 ) ) ;
#29721=CIRCLE ( 'NONE', #33551, 0.9999999999999947820 ) ;
#29722=CARTESIAN_POINT ( 'NONE',  ( -3.135527875058982783, 216.4958274776886924, 78.09886208192143897 ) ) ;
#29723=CARTESIAN_POINT ( 'NONE',  ( 7.375838497908181246, 196.7627149292499666, 101.4511379180785866 ) ) ;
#29725=CARTESIAN_POINT ( 'NONE',  ( -10.00000000000000711, 207.0476921513413515, 18.50113791807856956 ) ) ;
#29726=CARTESIAN_POINT ( 'NONE',  ( -10.01549611932659722, 210.2015048109875011, 92.64886208192143613 ) ) ;
#29732=DIRECTION ( 'NONE',  ( -0.9891821073486148919, -0.1466927349985451545, 0.000000000000000000 ) ) ;
#29733=CARTESIAN_POINT ( 'NONE',  ( 2.517493886309087436, 199.4062855549015865, 70.59886208192142476 ) ) ;
#29740=CARTESIAN_POINT ( 'NONE',  ( -8.000000000000008882, 207.0476921513413515, 72.50113791807856956 ) ) ;
#29746=CARTESIAN_POINT ( 'NONE',  ( 8.000000000000008882, 207.0476921513415220, 45.99886208192144466 ) ) ;
#29748=CARTESIAN_POINT ( 'NONE',  ( 9.984503880673470277, 203.7031108863295401, 89.15113791807857524 ) ) ;
#29749=CARTESIAN_POINT ( 'NONE',  ( 10.01549611932653860, 210.2015048109876716, 76.85113791807857808 ) ) ;
#29755=CARTESIAN_POINT ( 'NONE',  ( -12.01549611932652972, 203.1486557965464499, 48.35113791807857098 ) ) ;
#29757=CARTESIAN_POINT ( 'NONE',  ( -10.01549611932653860, 203.7984951890123284, 90.35113791807857808 ) ) ;
#29758=CARTESIAN_POINT ( 'NONE',  ( 3.135527875058820690, 216.4958274776887492, 67.40113791807857524 ) ) ;
#29759=CARTESIAN_POINT ( 'NONE',  ( -12.00000000000000711, 206.9523078486584780, 29.49886208192143400 ) ) ;
#29760=CARTESIAN_POINT ( 'NONE',  ( 8.118202686958138514, 201.1607312380088501, 40.29886208192143471 ) ) ;
#29762=CARTESIAN_POINT ( 'NONE',  ( 12.00000000000000711, 206.9523078486586485, 74.00113791807856956 ) ) ;
#29764=CARTESIAN_POINT ( 'NONE',  ( -2.426778023690262742, 214.6231898156240163, 97.10113791807857808 ) ) ;
#29765=CARTESIAN_POINT ( 'NONE',  ( 6.220909254589681581, 198.5229672870052582, 61.44886208192141908 ) ) ;
#29769=CARTESIAN_POINT ( 'NONE',  ( -11.98450388067341876, 203.0532714938636047, 59.34886208192144608 ) ) ;
#29772=CARTESIAN_POINT ( 'NONE',  ( 2.426778023690075337, 214.6231898156240447, 45.39886208192144323 ) ) ;
#29774=EDGE_CURVE ( 'NONE', #18219, #22743, #18167, .T. ) ;
#29779=CARTESIAN_POINT ( 'NONE',  ( 7.984503880673485376, 204.3529502787953902, 53.15113791807857524 ) ) ;
#29783=CARTESIAN_POINT ( 'NONE',  ( 0.05014649552828275708, 196.4853777576173002, 28.74886208192144110 ) ) ;
#29789=CARTESIAN_POINT ( 'NONE',  ( 6.444103211790928043, 211.7408657792734061, 12.69886208192143684 ) ) ;
#29792=CARTESIAN_POINT ( 'NONE',  ( -3.044812012440131443, 216.5253028482142952, 58.10113791807857808 ) ) ;
#29793=CARTESIAN_POINT ( 'NONE',  ( 8.118202686958039038, 212.8392687619912635, 34.70113791807857240 ) ) ;
#29798=CARTESIAN_POINT ( 'NONE',  ( -6.500168698208129925, 202.3363017425936050, 0.2011379180785659582 ) ) ;
#29802=CARTESIAN_POINT ( 'NONE',  ( -9.736236675707914401, 199.9851607334237542, 15.20113791807857062 ) ) ;
#29805=CARTESIAN_POINT ( 'NONE',  ( 0.05014649552810505201, 217.5146222423826714, 70.25113791807858377 ) ) ;
#29806=CARTESIAN_POINT ( 'NONE',  ( -10.01549611932653860, 203.7984951890123000, 36.35113791807857098 ) ) ;
#29810=CARTESIAN_POINT ( 'NONE',  ( -9.680171189290716072, 199.9079932115567146, 8.198862081921433287 ) ) ;
#29811=CARTESIAN_POINT ( 'NONE',  ( 3.044812012439969795, 216.5253028482143520, 12.39886208192143435 ) ) ;
#29814=CARTESIAN_POINT ( 'NONE',  ( -0.05014649552807705357, 194.3824533091408000, 50.75113791807857666 ) ) ;
#29815=CARTESIAN_POINT ( 'NONE',  ( -4.984841277089726574, 200.2242689037092305, 72.05113791807858092 ) ) ;
#29816=CARTESIAN_POINT ( 'NONE',  ( 6.139770520408223575, 215.5359834540460611, 33.54886208192143471 ) ) ;
#29819=CARTESIAN_POINT ( 'NONE',  ( 10.00000000000000711, 206.9523078486586201, 95.00113791807856956 ) ) ;
#29823=TOROIDAL_SURFACE ( 'NONE', #12407, 4.999999999999993783, 1.000000000000000222 ) ;
#29828=CARTESIAN_POINT ( 'NONE',  ( 4.984841277089725686, 213.7757310962907411, 25.55113791807857027 ) ) ;
#29830=CARTESIAN_POINT ( 'NONE',  ( 10.00000000000000711, 207.0476921513415220, 0.9988620819214343305 ) ) ;
#29835=CARTESIAN_POINT ( 'NONE',  ( 2.426778023690261410, 199.3768101843759837, 47.60113791807857808 ) ) ;
#29838=CARTESIAN_POINT ( 'NONE',  ( 3.135527875058981895, 197.5041725223112792, 94.59886208192143897 ) ) ;
#29840=CARTESIAN_POINT ( 'NONE',  ( 3.044812012440130555, 197.4746971517856764, 29.60113791807856742 ) ) ;
#29842=CARTESIAN_POINT ( 'NONE',  ( -9.736236675708031640, 214.0148392665760753, 77.79886208192142760 ) ) ;
#29846=CARTESIAN_POINT ( 'NONE',  ( 3.044812012440130555, 197.4746971517856764, 98.60113791807857808 ) ) ;
#29850=CARTESIAN_POINT ( 'NONE',  ( -8.118202686958039038, 201.1607312380087080, 33.20113791807857240 ) ) ;
#29857=CARTESIAN_POINT ( 'NONE',  ( 3.662846001190051659, 195.5725841191953691, 23.60113791807857098 ) ) ;
#29861=CARTESIAN_POINT ( 'NONE',  ( -9.680171189290716072, 199.9079932115567146, 47.19886208192143329 ) ) ;
#29862=FACE_OUTER_BOUND ( 'NONE', #3364, .T. ) ;
#29863=CARTESIAN_POINT ( 'NONE',  ( 8.062137200540920645, 201.0835637161417822, 47.30113791807857382 ) ) ;
#29864=CARTESIAN_POINT ( 'NONE',  ( -2.517493886309087880, 214.5937144450984135, 9.098862081921435419 ) ) ;
#29867=CARTESIAN_POINT ( 'NONE',  ( -4.984841277089891776, 213.7757310962905990, 95.94886208192144750 ) ) ;
#29870=CARTESIAN_POINT ( 'NONE',  ( -2.517493886308901807, 199.4062855549015012, 38.90113791807856813 ) ) ;
#29877=CARTESIAN_POINT ( 'NONE',  ( -6.139770520408224463, 198.4640165459539389, 65.04886208192144181 ) ) ;
#29880=CARTESIAN_POINT ( 'NONE',  ( 4.903702542908601636, 200.1653181626581102, 98.45113791807858661 ) ) ;
#29886=CARTESIAN_POINT ( 'NONE',  ( 2.426778023690075337, 214.6231898156240447, 78.39886208192143613 ) ) ;
#29890=CARTESIAN_POINT ( 'NONE',  ( -3.135527875058821579, 197.5041725223112223, 23.90113791807856813 ) ) ;
#29894=CARTESIAN_POINT ( 'NONE',  ( 3.753561863808689836, 218.3979405102790565, 85.40113791807856103 ) ) ;
#29898=ORIENTED_EDGE ( 'NONE', *, *, #14125, .T. ) ;
#29899=CARTESIAN_POINT ( 'NONE',  ( -9.680171189290716072, 199.9079932115567146, 74.19886208192143329 ) ) ;
#29900=CARTESIAN_POINT ( 'NONE',  ( -6.220909254589682469, 215.4770327129947134, 80.94886208192143329 ) ) ;
#29901=CARTESIAN_POINT ( 'NONE',  ( 9.736236675708031640, 199.9851607334238963, 13.29886208192143826 ) ) ;
#29903=CARTESIAN_POINT ( 'NONE',  ( -6.139770520408369237, 215.5359834540460042, 18.95113791807856884 ) ) ;
#29904=CARTESIAN_POINT ( 'NONE',  ( -3.135527875058982783, 216.4958274776886924, 93.09886208192145318 ) ) ;
#29909=CARTESIAN_POINT ( 'NONE',  ( 2.426778023690075337, 214.6231898156240447, 69.39886208192143613 ) ) ;
#29913=ORIENTED_EDGE ( 'NONE', *, *, #21677, .F. ) ;
#29918=CARTESIAN_POINT ( 'NONE',  ( -2.517493886308901807, 199.4062855549015012, 71.90113791807856103 ) ) ;
#29922=CARTESIAN_POINT ( 'NONE',  ( 4.984841277089891776, 200.2242689037093726, 49.44886208192144750 ) ) ;
#29924=CARTESIAN_POINT ( 'NONE',  ( 10.00000000000000711, 206.9523078486586201, 71.00113791807858377 ) ) ;
#29929=CARTESIAN_POINT ( 'NONE',  ( 11.98450388067348271, 203.0532714938637753, 56.15113791807857524 ) ) ;
#29931=CARTESIAN_POINT ( 'NONE',  ( -9.680171189290831535, 214.0920067884431148, 0.8011379180785656029 ) ) ;
#29932=CARTESIAN_POINT ( 'NONE',  ( -10.01549611932653860, 203.7984951890123000, 78.35113791807857808 ) ) ;
#29933=CARTESIAN_POINT ( 'NONE',  ( 7.456977232089471386, 196.8216656703012006, 34.44886208192142618 ) ) ;
#29934=CARTESIAN_POINT ( 'NONE',  ( -9.984503880673420539, 203.7031108863293980, 47.34886208192143187 ) ) ;
#29936=CARTESIAN_POINT ( 'NONE',  ( -12.00000000000000711, 207.0476921513413515, 90.50113791807858377 ) ) ;
#29937=CARTESIAN_POINT ( 'NONE',  ( 4.984841277089725686, 213.7757310962907411, 100.5511379180785809 ) ) ;
#29939=CARTESIAN_POINT ( 'NONE',  ( -6.139770520408224463, 198.4640165459539389, 56.04886208192142050 ) ) ;
#29941=CARTESIAN_POINT ( 'NONE',  ( 0.05014649552828288198, 194.3824533091408000, 61.74886208192143755 ) ) ;
#29944=CARTESIAN_POINT ( 'NONE',  ( -4.903702542908436435, 200.1653181626580249, 38.04886208192144892 ) ) ;
#29948=CARTESIAN_POINT ( 'NONE',  ( -9.000000000000001776, 206.9999999999998863, 103.5000000000000426 ) ) ;
#29950=CARTESIAN_POINT ( 'NONE',  ( -4.903702542908602524, 213.8346818373418898, 60.95113791807857240 ) ) ;
#29951=CARTESIAN_POINT ( 'NONE',  ( -3.942127870247283283, 206.4478425060960376, -5.603442290337207865 ) ) ;
#29952=CARTESIAN_POINT ( 'NONE',  ( 3.135527875058981895, 197.5041725223112792, 46.59886208192143187 ) ) ;
#29959=CARTESIAN_POINT ( 'NONE',  ( 8.000000000000008882, 207.0476921513415220, 18.99886208192143400 ) ) ;
#29960=CARTESIAN_POINT ( 'NONE',  ( -6.139770520408369237, 215.5359834540460042, 63.95113791807857950 ) ) ;
#29961=CARTESIAN_POINT ( 'NONE',  ( -6.139770520408369237, 215.5359834540460042, 48.95113791807855108 ) ) ;
#29963=CARTESIAN_POINT ( 'NONE',  ( 3.135527875058820690, 216.4958274776887492, 22.40113791807856458 ) ) ;
#29964=CARTESIAN_POINT ( 'NONE',  ( 8.015496119326595448, 204.4483345814782638, 103.1488620819214361 ) ) ;
#29968=CARTESIAN_POINT ( 'NONE',  ( -7.456977232089304408, 196.8216656703010301, 24.05113791807857027 ) ) ;
#29971=CARTESIAN_POINT ( 'NONE',  ( 10.00000000000000711, 206.9523078486586201, 77.00113791807858377 ) ) ;
#29972=CARTESIAN_POINT ( 'NONE',  ( -8.118202686958039038, 201.1607312380087080, 36.20113791807857240 ) ) ;
#29975=CARTESIAN_POINT ( 'NONE',  ( -9.736236675708031640, 214.0148392665760753, 8.798862081921434708 ) ) ;
#29976=CARTESIAN_POINT ( 'NONE',  ( -9.984503880673420539, 203.7031108863293980, 23.34886208192143187 ) ) ;
#29980=CARTESIAN_POINT ( 'NONE',  ( -9.680171189290831535, 214.0920067884431148, 45.80113791807856671 ) ) ;
#29981=CARTESIAN_POINT ( 'NONE',  ( 8.015496119326531499, 209.5516654185219636, 73.85113791807857808 ) ) ;
#29983=CARTESIAN_POINT ( 'NONE',  ( 6.139770520408223575, 215.5359834540460611, 27.54886208192142760 ) ) ;
#29986=CARTESIAN_POINT ( 'NONE',  ( -6.139770520408369237, 215.5359834540460042, 93.95113791807854398 ) ) ;
#29992=CARTESIAN_POINT ( 'NONE',  ( 8.000000000000008882, 206.9523078486586485, 23.00113791807856600 ) ) ;
#29994=CARTESIAN_POINT ( 'NONE',  ( -3.044812012439970683, 197.4746971517856196, 4.898862081921434353 ) ) ;
#29997=CARTESIAN_POINT ( 'NONE',  ( 8.000000000000008882, 206.9523078486586485, 50.00113791807856956 ) ) ;
#30000=CARTESIAN_POINT ( 'NONE',  ( 9.984503880673420539, 210.2968891136705167, 87.84886208192141055 ) ) ;
#30002=CARTESIAN_POINT ( 'NONE',  ( 0.05014649552810505201, 217.5146222423826714, 31.25113791807857311 ) ) ;
#30004=CARTESIAN_POINT ( 'NONE',  ( 10.01549611932653860, 210.2015048109876716, 16.85113791807856032 ) ) ;
#30008=CARTESIAN_POINT ( 'NONE',  ( -6.220909254589537696, 198.5229672870051161, 90.05113791807858092 ) ) ;
#30011=CARTESIAN_POINT ( 'NONE',  ( 8.062137200540920645, 201.0835637161417822, 35.30113791807857382 ) ) ;
#30018=CARTESIAN_POINT ( 'NONE',  ( -3.662846001190052991, 218.4274158808045740, 19.10113791807856742 ) ) ;
#30024=CARTESIAN_POINT ( 'NONE',  ( -9.680171189290716072, 199.9079932115567146, 38.19886208192142618 ) ) ;
#30026=CARTESIAN_POINT ( 'NONE',  ( -10.01549611932653860, 203.7984951890123284, 60.35113791807857808 ) ) ;
#30027=CARTESIAN_POINT ( 'NONE',  ( -8.000000000000008882, 206.9523078486584780, 14.49886208192143577 ) ) ;
#30030=CARTESIAN_POINT ( 'NONE',  ( -4.984841277089891776, 213.7757310962905990, 98.94886208192143329 ) ) ;
#30032=CARTESIAN_POINT ( 'NONE',  ( 4.903702542908601636, 200.1653181626581102, 38.45113791807856529 ) ) ;
#30037=CARTESIAN_POINT ( 'NONE',  ( -8.062137200540920645, 212.9164362838581894, 0.8011379180785658249 ) ) ;
#30039=CARTESIAN_POINT ( 'NONE',  ( 3.044812012439969795, 216.5253028482143520, 66.39886208192143613 ) ) ;
#30042=CARTESIAN_POINT ( 'NONE',  ( 6.139770520408368348, 198.4640165459539674, 5.451137918078567068 ) ) ;
#30045=CARTESIAN_POINT ( 'NONE',  ( 2.517493886309087436, 199.4062855549015865, 85.59886208192143897 ) ) ;
#30049=CARTESIAN_POINT ( 'NONE',  ( -8.062137200540920645, 212.9164362838581894, 24.80113791807857027 ) ) ;
#30054=CARTESIAN_POINT ( 'NONE',  ( -3.753561863808691168, 195.6020594897209435, 89.90113791807857524 ) ) ;
#30059=CARTESIAN_POINT ( 'NONE',  ( -12.01549611932659722, 210.8513442034533227, 71.64886208192143613 ) ) ;
#30060=CARTESIAN_POINT ( 'NONE',  ( -0.05014649552828402690, 217.5146222423826714, 75.24886208192144466 ) ) ;
#30061=CARTESIAN_POINT ( 'NONE',  ( 12.01549611932659367, 203.1486557965466773, 16.14886208192143613 ) ) ;
#30063=CARTESIAN_POINT ( 'NONE',  ( 3.135527875058820690, 216.4958274776887492, 28.40113791807856813 ) ) ;
#30064=CARTESIAN_POINT ( 'NONE',  ( 9.379977934355910207, 208.8253170565643870, -1.014254689207407356 ) ) ;
#30065=CARTESIAN_POINT ( 'NONE',  ( -9.984503880673420539, 203.7031108863293980, 86.34886208192143897 ) ) ;
#30069=DIRECTION ( 'NONE',  ( -0.1461455375466716444, 0.9854922318508084755, -0.08629335326029916042 ) ) ;
#30070=CARTESIAN_POINT ( 'NONE',  ( -7.984503880673422316, 204.3529502787951628, 71.34886208192142476 ) ) ;
#30079=CARTESIAN_POINT ( 'NONE',  ( -2.517493886308901807, 199.4062855549015012, 80.90113791807858945 ) ) ;
#30082=CARTESIAN_POINT ( 'NONE',  ( -2.517493886309087880, 214.5937144450984135, 54.09886208192143897 ) ) ;
#30089=CARTESIAN_POINT ( 'NONE',  ( 12.00000000000000711, 206.9523078486586485, 56.00113791807856956 ) ) ;
#30092=CARTESIAN_POINT ( 'NONE',  ( 0.05014649552807549926, 219.6175466908591716, 4.251137918078565114 ) ) ;
#30093=CARTESIAN_POINT ( 'NONE',  ( 3.135527875058820690, 216.4958274776887492, 79.40113791807857524 ) ) ;
#30094=CARTESIAN_POINT ( 'NONE',  ( -3.753561863808878130, 218.3979405102790281, 42.09886208192143897 ) ) ;
#30095=CARTESIAN_POINT ( 'NONE',  ( -6.139770520408224463, 198.4640165459539105, 50.04886208192143471 ) ) ;
#30098=CARTESIAN_POINT ( 'NONE',  ( -3.662846001190052991, 218.4274158808045740, 91.10113791807859229 ) ) ;
#30099=CARTESIAN_POINT ( 'NONE',  ( -6.500168698208129925, 202.3363017425936050, 102.2011379180785866 ) ) ;
#30101=CARTESIAN_POINT ( 'NONE',  ( -6.220909254589682469, 215.4770327129946850, 56.94886208192141908 ) ) ;
#30106=CARTESIAN_POINT ( 'NONE',  ( 12.00000000000000711, 207.0476921513415220, 69.99886208192144466 ) ) ;
#30109=CARTESIAN_POINT ( 'NONE',  ( -4.903702542908436435, 200.1653181626580249, 41.04886208192144181 ) ) ;
#30116=CARTESIAN_POINT ( 'NONE',  ( 7.984503880673485376, 204.3529502787953902, 62.15113791807858945 ) ) ;
#30118=CARTESIAN_POINT ( 'NONE',  ( -6.139770520408224463, 198.4640165459539389, 41.04886208192142760 ) ) ;
#30122=FILL_AREA_STYLE ('',( #11557 ) ) ;
#30125=CARTESIAN_POINT ( 'NONE',  ( -4.903702542908436435, 200.1653181626580249, 23.04886208192143826 ) ) ;
#30127=CARTESIAN_POINT ( 'NONE',  ( 8.118202686958039038, 212.8392687619912635, 64.70113791807857240 ) ) ;
#30128=CARTESIAN_POINT ( 'NONE',  ( -9.984503880673473830, 210.2968891136704315, 45.65113791807855392 ) ) ;
#30131=CARTESIAN_POINT ( 'NONE',  ( 0.05014649552810505201, 217.5146222423826714, 19.25113791807856600 ) ) ;
#30132=CARTESIAN_POINT ( 'NONE',  ( 4.984841277089725686, 213.7757310962907411, 7.551137918078564049 ) ) ;
#30136=CARTESIAN_POINT ( 'NONE',  ( 12.00000000000000711, 206.9523078486586485, 26.00113791807856600 ) ) ;
#30139=CARTESIAN_POINT ( 'NONE',  ( -6.220909254589537696, 198.5229672870051161, 75.05113791807858092 ) ) ;
#30140=CARTESIAN_POINT ( 'NONE',  ( 10.00000000000000711, 206.9523078486586201, 53.00113791807857666 ) ) ;
#30144=CARTESIAN_POINT ( 'NONE',  ( -7.456977232089471386, 217.1783343296987709, 17.94886208192143684 ) ) ;
#30145=CARTESIAN_POINT ( 'NONE',  ( 10.00000000000000711, 207.0476921513415220, 15.99886208192143400 ) ) ;
#30148=CARTESIAN_POINT ( 'NONE',  ( 3.753561863808689836, 218.3979405102790565, 58.40113791807858235 ) ) ;
#30149=CARTESIAN_POINT ( 'NONE',  ( 6.500168698208129925, 211.6636982574063381, 67.70113791807857240 ) ) ;
#30150=CARTESIAN_POINT ( 'NONE',  ( -10.01549611932659722, 210.2015048109875011, 35.64886208192143613 ) ) ;
#30154=CARTESIAN_POINT ( 'NONE',  ( -3.135527875058821579, 197.5041725223112223, 86.90113791807857524 ) ) ;
#30161=CARTESIAN_POINT ( 'NONE',  ( -7.984503880673488041, 209.6470497212046098, 30.65113791807856458 ) ) ;
#30163=CARTESIAN_POINT ( 'NONE',  ( 0.05014649552828275708, 196.4853777576173002, 16.74886208192143755 ) ) ;
#30166=CARTESIAN_POINT ( 'NONE',  ( -2.517493886308901807, 199.4062855549015012, 53.90113791807858235 ) ) ;
#30170=CARTESIAN_POINT ( 'NONE',  ( -9.984503880673420539, 203.7031108863293980, 101.3488620819213963 ) ) ;
#30172=CARTESIAN_POINT ( 'NONE',  ( -3.044812012440131443, 216.5253028482142952, 28.10113791807857098 ) ) ;
#30175=CARTESIAN_POINT ( 'NONE',  ( -8.062137200540920645, 212.9164362838581894, 18.80113791807856671 ) ) ;
#30180=CARTESIAN_POINT ( 'NONE',  ( -3.662846001190052991, 218.4274158808045740, 1.101137918078565647 ) ) ;
#30184=CARTESIAN_POINT ( 'NONE',  ( 8.062137200540920645, 201.0835637161417822, 44.30113791807857382 ) ) ;
#30190=CARTESIAN_POINT ( 'NONE',  ( 9.680171189290831535, 199.9079932115568852, 26.30113791807856316 ) ) ;
#30194=CARTESIAN_POINT ( 'NONE',  ( -11.98450388067341876, 203.0532714938636047, 44.34886208192143897 ) ) ;
#30195=CARTESIAN_POINT ( 'NONE',  ( -6.220909254589537696, 198.5229672870051161, 3.051137918078564937 ) ) ;
#30196=CARTESIAN_POINT ( 'NONE',  ( 0.05014649552810505201, 217.5146222423826714, 61.25113791807856245 ) ) ;
#30197=CARTESIAN_POINT ( 'NONE',  ( -0.05014649552828365914, 215.4116977939061144, 27.24886208192143755 ) ) ;
#30200=CARTESIAN_POINT ( 'NONE',  ( 8.000000000000008882, 206.9523078486586485, -0.9988620819214343305 ) ) ;
#30204=CARTESIAN_POINT ( 'NONE',  ( 0.05014649552828288198, 194.3824533091408000, 88.74886208192143044 ) ) ;
#30206=ORIENTED_EDGE ( 'NONE', *, *, #1654, .T. ) ;
#30210=CARTESIAN_POINT ( 'NONE',  ( 6.139770520408223575, 215.5359834540460611, 57.54886208192142050 ) ) ;
#30214=CARTESIAN_POINT ( 'NONE',  ( 3.135527875058820690, 216.4958274776887492, 1.401137918078565914 ) ) ;
#30219=CARTESIAN_POINT ( 'NONE',  ( 4.984841277089891776, 200.2242689037093726, 79.44886208192144750 ) ) ;
#30223=CARTESIAN_POINT ( 'NONE',  ( -7.375838497908014268, 196.7627149292498530, 83.04886208192144181 ) ) ;
#30225=CARTESIAN_POINT ( 'NONE',  ( -8.118202686958039038, 201.1607312380087080, 18.20113791807856884 ) ) ;
#30227=CARTESIAN_POINT ( 'NONE',  ( -10.00000000000000178, 206.0011379180784559, 103.4523078486585916 ) ) ;
#30229=CARTESIAN_POINT ( 'NONE',  ( -3.662846001190052991, 218.4274158808045740, 82.10113791807857808 ) ) ;
#30232=CARTESIAN_POINT ( 'NONE',  ( -9.680171189290716072, 199.9079932115567146, 68.19886208192143329 ) ) ;
#30233=CARTESIAN_POINT ( 'NONE',  ( 9.984503880673420539, 210.2968891136705736, 75.84886208192143897 ) ) ;
#30234=CARTESIAN_POINT ( 'NONE',  ( -0.05014649552828442242, 219.6175466908591716, 18.24886208192143755 ) ) ;
#30236=CARTESIAN_POINT ( 'NONE',  ( 0.05014649552810505201, 217.5146222423826714, 31.25113791807857311 ) ) ;
#30238=CARTESIAN_POINT ( 'NONE',  ( 10.01549611932659545, 203.7984951890123853, 103.1488620819214077 ) ) ;
#30242=CARTESIAN_POINT ( 'NONE',  ( 2.517493886309087436, 199.4062855549015865, 67.59886208192143897 ) ) ;
#30250=CARTESIAN_POINT ( 'NONE',  ( 4.903702542908601636, 200.1653181626581102, 77.45113791807855819 ) ) ;
#30253=CARTESIAN_POINT ( 'NONE',  ( -4.903702542908436435, 200.1653181626580249, 50.04886208192144181 ) ) ;
#30260=CARTESIAN_POINT ( 'NONE',  ( -12.00000000000000711, 207.0476921513413515, 54.50113791807857666 ) ) ;
#30262=CARTESIAN_POINT ( 'NONE',  ( -9.736236675707914401, 199.9851607334237542, 0.2011379180785655418 ) ) ;
#30263=CARTESIAN_POINT ( 'NONE',  ( -8.062137200540920645, 212.9164362838581894, 81.80113791807858092 ) ) ;
#30264=CARTESIAN_POINT ( 'NONE',  ( -3.753561863808878130, 218.3979405102790281, 45.09886208192143897 ) ) ;
#30265=CARTESIAN_POINT ( 'NONE',  ( -8.062137200540822946, 201.0835637161416400, 50.19886208192144039 ) ) ;
#30267=CARTESIAN_POINT ( 'NONE',  ( 7.456977232089302632, 217.1783343296989131, 91.55113791807858092 ) ) ;
#30269=CARTESIAN_POINT ( 'NONE',  ( 10.01549611932653860, 210.2015048109876716, 4.851137918078563871 ) ) ;
#30270=CARTESIAN_POINT ( 'NONE',  ( 9.984503880673420539, 210.2968891136705167, 66.84886208192141055 ) ) ;
#30273=CARTESIAN_POINT ( 'NONE',  ( 3.753561863808876797, 195.6020594897209719, 67.59886208192143897 ) ) ;
#30276=CARTESIAN_POINT ( 'NONE',  ( -2.517493886309087880, 214.5937144450984135, 45.09886208192144608 ) ) ;
#30284=CARTESIAN_POINT ( 'NONE',  ( -10.01549611932659722, 210.2015048109875011, 44.64886208192143613 ) ) ;
#30290=CARTESIAN_POINT ( 'NONE',  ( 2.426778023690075337, 214.6231898156240447, 27.39886208192143613 ) ) ;
#30291=CARTESIAN_POINT ( 'NONE',  ( 3.044812012440130555, 197.4746971517856764, 56.60113791807857098 ) ) ;
#30293=CARTESIAN_POINT ( 'NONE',  ( 8.062137200540920645, 201.0835637161417822, 47.30113791807857382 ) ) ;
#30296=CARTESIAN_POINT ( 'NONE',  ( -10.01549611932653860, 203.7984951890123284, 15.35113791807856565 ) ) ;
#30297=CARTESIAN_POINT ( 'NONE',  ( -6.500168698208129925, 202.3363017425936050, 3.201137918078566624 ) ) ;
#30301=CARTESIAN_POINT ( 'NONE',  ( 3.753561863808689836, 218.3979405102790565, 31.40113791807856813 ) ) ;
#30304=CARTESIAN_POINT ( 'NONE',  ( 3.135527875058820690, 216.4958274776887492, 76.40113791807857524 ) ) ;
#30305=CARTESIAN_POINT ( 'NONE',  ( -6.139770520408368348, 215.5359834540460042, 48.95113791807857240 ) ) ;
#30309=CARTESIAN_POINT ( 'NONE',  ( -12.01549611932659722, 210.8513442034533227, 11.64886208192143613 ) ) ;
#30310=CARTESIAN_POINT ( 'NONE',  ( -6.220909254589682469, 215.4770327129947134, 17.94886208192143684 ) ) ;
#30313=CARTESIAN_POINT ( 'NONE',  ( -3.753561863808691168, 195.6020594897209435, 53.90113791807858235 ) ) ;
#30314=CARTESIAN_POINT ( 'NONE',  ( 2.517493886308900919, 214.5937144450984420, 82.40113791807856103 ) ) ;
#30315=CARTESIAN_POINT ( 'NONE',  ( -8.118202686958138514, 212.8392687619910930, 26.79886208192143826 ) ) ;
#30324=CARTESIAN_POINT ( 'NONE',  ( -4.984841277089726574, 200.2242689037092305, 33.05113791807857382 ) ) ;
#30328=CARTESIAN_POINT ( 'NONE',  ( -8.118202686958138514, 212.8392687619910930, 17.79886208192143826 ) ) ;
#30331=CARTESIAN_POINT ( 'NONE',  ( -8.000000000000008882, 207.0476921513413515, 48.50113791807856956 ) ) ;
#30336=CARTESIAN_POINT ( 'NONE',  ( 6.139770520408223575, 215.5359834540460611, 96.54886208192141339 ) ) ;
#30338=CARTESIAN_POINT ( 'NONE',  ( -3.135527875058821579, 197.5041725223112223, 32.90113791807857524 ) ) ;
#30341=CARTESIAN_POINT ( 'NONE',  ( -6.139770520408369237, 215.5359834540460042, 15.95113791807856884 ) ) ;
#30347=CARTESIAN_POINT ( 'NONE',  ( -3.753561863808691168, 195.6020594897209435, -0.09886208192143448870 ) ) ;
#30350=CARTESIAN_POINT ( 'NONE',  ( -8.062137200540920645, 212.9164362838581894, 48.80113791807857382 ) ) ;
#30357=CARTESIAN_POINT ( 'NONE',  ( -9.680171189290831535, 214.0920067884431148, 30.80113791807857027 ) ) ;
#30360=CARTESIAN_POINT ( 'NONE',  ( 10.00000000000000711, 207.0476921513415220, 6.998862081921434886 ) ) ;
#30365=CARTESIAN_POINT ( 'NONE',  ( 0.05014649552810505201, 217.5146222423826714, 4.251137918078566003 ) ) ;
#30366=CARTESIAN_POINT ( 'NONE',  ( 8.062137200540920645, 201.0835637161417822, 65.30113791807858092 ) ) ;
#30368=CARTESIAN_POINT ( 'NONE',  ( 4.984841277089891776, 200.2242689037093726, 25.44886208192143684 ) ) ;
#30372=CARTESIAN_POINT ( 'NONE',  ( 7.984503880673485376, 204.3529502787953902, 5.151137918078566358 ) ) ;
#30375=CARTESIAN_POINT ( 'NONE',  ( 7.375838497908012492, 217.2372850707501186, 90.54886208192144181 ) ) ;
#30382=CARTESIAN_POINT ( 'NONE',  ( 10.00000000000000711, 207.0476921513415220, 72.99886208192144466 ) ) ;
#30385=CARTESIAN_POINT ( 'NONE',  ( 6.220909254589536808, 215.4770327129947702, 7.551137918078564049 ) ) ;
#30388=CARTESIAN_POINT ( 'NONE',  ( -0.05014649552810635652, 196.4853777576173002, 89.75113791807854113 ) ) ;
#30390=CARTESIAN_POINT ( 'NONE',  ( -7.984503880673422316, 204.3529502787951628, 80.34886208192143897 ) ) ;
#30393=CARTESIAN_POINT ( 'NONE',  ( 12.00000000000000711, 207.0476921513415220, 84.99886208192144466 ) ) ;
#30396=CARTESIAN_POINT ( 'NONE',  ( 6.220909254589536808, 215.4770327129947987, 22.55113791807856671 ) ) ;
#30398=LINE ( 'NONE', #30227, #22245 ) ;
#30400=CARTESIAN_POINT ( 'NONE',  ( -7.456977232089304408, 196.8216656703010301, 90.05113791807858092 ) ) ;
#30405=CARTESIAN_POINT ( 'NONE',  ( -0.05014649552828442242, 219.6175466908591716, 72.24886208192143044 ) ) ;
#30406=CARTESIAN_POINT ( 'NONE',  ( 10.00000000000000711, 207.0476921513415220, 72.99886208192144466 ) ) ;
#30407=CARTESIAN_POINT ( 'NONE',  ( 7.375838497908012492, 217.2372850707501186, 18.54886208192143116 ) ) ;
#30410=CARTESIAN_POINT ( 'NONE',  ( 6.139770520408368348, 198.4640165459539674, 35.45113791807857240 ) ) ;
#30413=CARTESIAN_POINT ( 'NONE',  ( -3.044812012439970683, 197.4746971517856196, 100.8988620819214361 ) ) ;
#30418=CARTESIAN_POINT ( 'NONE',  ( 2.517493886309087436, 199.4062855549015865, 76.59886208192142476 ) ) ;
#30426=CARTESIAN_POINT ( 'NONE',  ( 4.984841277089725686, 213.7757310962907411, 82.55113791807858092 ) ) ;
#30429=CARTESIAN_POINT ( 'NONE',  ( 8.015496119326595448, 204.4483345814782638, 58.14886208192145034 ) ) ;
#30436=CARTESIAN_POINT ( 'NONE',  ( -3.753561863808691168, 195.6020594897209435, 53.90113791807858235 ) ) ;
#30438=CARTESIAN_POINT ( 'NONE',  ( 10.00000000000000711, 206.9523078486586201, 101.0011379180785696 ) ) ;
#30440=CARTESIAN_POINT ( 'NONE',  ( -6.139770520408368348, 215.5359834540460042, 75.95113791807857240 ) ) ;
#30441=CARTESIAN_POINT ( 'NONE',  ( -7.456977232089471386, 217.1783343296987709, 44.94886208192144039 ) ) ;
#30442=CARTESIAN_POINT ( 'NONE',  ( -8.118202686958138514, 212.8392687619910930, 50.79886208192143471 ) ) ;
#30444=CARTESIAN_POINT ( 'NONE',  ( -9.736236675707914401, 199.9851607334237542, 87.20113791807858661 ) ) ;
#30446=CARTESIAN_POINT ( 'NONE',  ( 6.139770520408368348, 198.4640165459539674, 5.451137918078567068 ) ) ;
#30447=CARTESIAN_POINT ( 'NONE',  ( -10.01549611932659722, 210.2015048109875011, 65.64886208192143613 ) ) ;
#30450=CARTESIAN_POINT ( 'NONE',  ( 11.98450388067341876, 210.9467285061363953, 69.84886208192143897 ) ) ;
#30453=CARTESIAN_POINT ( 'NONE',  ( -6.500168698208244500, 211.6636982574061676, 50.79886208192144892 ) ) ;
#30461=CARTESIAN_POINT ( 'NONE',  ( 9.984503880673420539, 210.2968891136705167, 45.84886208192141765 ) ) ;
#30467=CARTESIAN_POINT ( 'NONE',  ( -4.984841277089891776, 213.7757310962905990, 26.94886208192142973 ) ) ;
#30468=CARTESIAN_POINT ( 'NONE',  ( -8.118202686958039038, 201.1607312380087080, 57.20113791807857950 ) ) ;
#30469=CARTESIAN_POINT ( 'NONE',  ( 8.118202686958039038, 212.8392687619912635, 49.70113791807857240 ) ) ;
#30470=CARTESIAN_POINT ( 'NONE',  ( 3.135527875058820690, 216.4958274776887492, 13.40113791807856636 ) ) ;
#30471=CARTESIAN_POINT ( 'NONE',  ( 2.517493886308900919, 214.5937144450984420, 1.401137918078566136 ) ) ;
#30475=CARTESIAN_POINT ( 'NONE',  ( -7.375838497908182134, 217.2372850707499765, 24.95113791807856884 ) ) ;
#30476=DIRECTION ( 'NONE',  ( 0.000000000000000000, -0.04769215134144040580, 0.9988620819214356628 ) ) ;
#30477=CARTESIAN_POINT ( 'NONE',  ( -10.01549611932653860, 203.7984951890123284, 72.35113791807859229 ) ) ;
#30478=CARTESIAN_POINT ( 'NONE',  ( 10.00000000000000711, 206.9523078486586201, 47.00113791807856956 ) ) ;
#30481=CARTESIAN_POINT ( 'NONE',  ( 12.00000000000000711, 207.0476921513415220, 15.99886208192143400 ) ) ;
#30482=CARTESIAN_POINT ( 'NONE',  ( 6.139770520408223575, 215.5359834540460611, 21.54886208192143826 ) ) ;
#30485=CARTESIAN_POINT ( 'NONE',  ( 9.736236675707914401, 214.0148392665762458, 55.70113791807856529 ) ) ;
#30486=CARTESIAN_POINT ( 'NONE',  ( 0.05014649552807626948, 215.4116977939061144, 82.25113791807856956 ) ) ;
#30487=CARTESIAN_POINT ( 'NONE',  ( 9.984503880673420539, 210.2968891136705167, 39.84886208192141765 ) ) ;
#30496=CARTESIAN_POINT ( 'NONE',  ( 7.984503880673485376, 204.3529502787953902, 35.15113791807856103 ) ) ;
#30497=DIRECTION ( 'NONE',  ( 0.000000000000000000, 0.9988620819214357738, 0.04769215134144196705 ) ) ;
#30498=CARTESIAN_POINT ( 'NONE',  ( -9.984503880673420539, 203.7031108863293980, 11.34886208192143187 ) ) ;
#30501=CARTESIAN_POINT ( 'NONE',  ( -4.903702542908602524, 213.8346818373418898, 63.95113791807857240 ) ) ;
#30504=CARTESIAN_POINT ( 'NONE',  ( -8.118202686958138514, 212.8392687619910930, 101.7988620819214418 ) ) ;
#30506=CARTESIAN_POINT ( 'NONE',  ( 10.00000000000000711, 206.9523078486586201, 35.00113791807856956 ) ) ;
#30508=CARTESIAN_POINT ( 'NONE',  ( 0.05014649552810505201, 217.5146222423826714, 22.25113791807856956 ) ) ;
#30514=CARTESIAN_POINT ( 'NONE',  ( -3.753561863808691168, 195.6020594897209435, 2.901137918078565470 ) ) ;
#30517=CARTESIAN_POINT ( 'NONE',  ( 6.139770520408368348, 198.4640165459539674, 44.45113791807855819 ) ) ;
#30523=CARTESIAN_POINT ( 'NONE',  ( -7.456977232089304408, 196.8216656703010301, 30.05113791807857027 ) ) ;
#30525=CARTESIAN_POINT ( 'NONE',  ( 6.220909254589681581, 198.5229672870052582, 13.44886208192143151 ) ) ;
#30529=CARTESIAN_POINT ( 'NONE',  ( 8.062137200540920645, 201.0835637161417822, 2.301137918078566269 ) ) ;
#30530=CARTESIAN_POINT ( 'NONE',  ( -9.984503880673473830, 210.2968891136704315, 60.65113791807856103 ) ) ;
#30532=CARTESIAN_POINT ( 'NONE',  ( -8.000000000000008882, 206.9523078486584780, 20.49886208192143755 ) ) ;
#30537=CARTESIAN_POINT ( 'NONE',  ( -7.984503880673488041, 209.6470497212046098, 3.651137918078566802 ) ) ;
#30540=CARTESIAN_POINT ( 'NONE',  ( -3.662846001189865142, 195.5725841191952838, 91.89886208192143613 ) ) ;
#30545=EDGE_CURVE ( 'NONE', #19921, #24261, #5663, .T. ) ;
#30547=CARTESIAN_POINT ( 'NONE',  ( 0.05014649552828275708, 196.4853777576173002, 73.74886208192144466 ) ) ;
#30550=CARTESIAN_POINT ( 'NONE',  ( -6.220909254589537696, 198.5229672870051161, 0.05113791807856577637 ) ) ;
#30554=CARTESIAN_POINT ( 'NONE',  ( -10.01549611932653860, 203.7984951890123284, 93.35113791807857808 ) ) ;
#30556=CARTESIAN_POINT ( 'NONE',  ( 10.01549611932653860, 210.2015048109876716, 70.85113791807854966 ) ) ;
#30559=CARTESIAN_POINT ( 'NONE',  ( 9.736236675708031640, 199.9851607334238963, 91.29886208192142760 ) ) ;
#30561=CARTESIAN_POINT ( 'NONE',  ( -8.062137200540920645, 212.9164362838581894, 33.80113791807857382 ) ) ;
#30565=CARTESIAN_POINT ( 'NONE',  ( -9.736236675707914401, 199.9851607334237542, 84.20113791807858661 ) ) ;
#30567=ADVANCED_FACE ( 'NONE', ( #15510 ), #31351, .T. ) ;
#30570=CARTESIAN_POINT ( 'NONE',  ( 6.139770520408223575, 215.5359834540460611, 84.54886208192142760 ) ) ;
#30572=CARTESIAN_POINT ( 'NONE',  ( 11.98450388067341876, 210.9467285061363953, 15.84886208192143719 ) ) ;
#30574=CARTESIAN_POINT ( 'NONE',  ( -10.00000000000000711, 207.0476921513413515, 33.50113791807856956 ) ) ;
#30576=CARTESIAN_POINT ( 'NONE',  ( -3.135527875058982783, 216.4958274776886924, 99.09886208192143897 ) ) ;
#30580=CARTESIAN_POINT ( 'NONE',  ( -9.945352646237287431, 205.9548993908332193, 104.4520571433695579 ) ) ;
#30581=CARTESIAN_POINT ( 'NONE',  ( -4.984841277089891776, 213.7757310962905990, 77.94886208192143329 ) ) ;
#30590=CARTESIAN_POINT ( 'NONE',  ( 4.903702542908601636, 200.1653181626581102, 83.45113791807857240 ) ) ;
#30596=CARTESIAN_POINT ( 'NONE',  ( -7.984503880673422316, 204.3529502787951628, 53.34886208192144608 ) ) ;
#30603=CARTESIAN_POINT ( 'NONE',  ( -7.375838497908182134, 217.2372850707499765, 60.95113791807857240 ) ) ;
#30606=CARTESIAN_POINT ( 'NONE',  ( 3.044812012440130555, 197.4746971517856764, 101.6011379180785781 ) ) ;
#30607=CARTESIAN_POINT ( 'NONE',  ( 6.139770520408367460, 198.4640165459539389, 74.45113791807857240 ) ) ;
#30608=CARTESIAN_POINT ( 'NONE',  ( -9.680171189290716072, 199.9079932115567146, 47.19886208192143329 ) ) ;
#30610=CARTESIAN_POINT ( 'NONE',  ( 8.062137200540822946, 212.9164362838583315, 51.69886208192143329 ) ) ;
#30612=CARTESIAN_POINT ( 'NONE',  ( -7.375838497908182134, 217.2372850707499765, 87.95113791807857240 ) ) ;
#30614=CARTESIAN_POINT ( 'NONE',  ( 8.118202686958039038, 212.8392687619912635, 7.701137918078566180 ) ) ;
#30615=CARTESIAN_POINT ( 'NONE',  ( -8.118202686958138514, 212.8392687619910930, 68.79886208192144181 ) ) ;
#30618=CARTESIAN_POINT ( 'NONE',  ( 12.00000000000000711, 207.0476921513415220, 75.99886208192144466 ) ) ;
#30621=CARTESIAN_POINT ( 'NONE',  ( 7.984503880673422316, 209.6470497212048372, 51.84886208192144608 ) ) ;
#30632=CARTESIAN_POINT ( 'NONE',  ( -8.118202686958138514, 212.8392687619910930, 41.79886208192143471 ) ) ;
#30638=CARTESIAN_POINT ( 'NONE',  ( -8.015496119326597224, 209.5516654185217362, 29.64886208192143968 ) ) ;
#30639=CARTESIAN_POINT ( 'NONE',  ( 3.044812012440130555, 197.4746971517856764, 74.60113791807856387 ) ) ;
#30642=CARTESIAN_POINT ( 'NONE',  ( -3.135527875058821579, 197.5041725223112223, 50.90113791807856813 ) ) ;
#30643=CARTESIAN_POINT ( 'NONE',  ( -8.062137200540920645, 212.9164362838581894, 18.80113791807856671 ) ) ;
#30644=CARTESIAN_POINT ( 'NONE',  ( 7.984503880673485376, 204.3529502787953902, 8.151137918078566358 ) ) ;
#30648=CARTESIAN_POINT ( 'NONE',  ( 9.680171189290831535, 199.9079932115568852, 32.30113791807855961 ) ) ;
#30651=CARTESIAN_POINT ( 'NONE',  ( -8.062137200540920645, 212.9164362838581894, 75.80113791807858092 ) ) ;
#30652=CARTESIAN_POINT ( 'NONE',  ( 10.00000000000000711, 206.9523078486586201, 50.00113791807856956 ) ) ;
#30656=CARTESIAN_POINT ( 'NONE',  ( -3.662846001189865142, 195.5725841191952838, 16.89886208192143613 ) ) ;
#30657=CARTESIAN_POINT ( 'NONE',  ( 10.01549611932659367, 203.7984951890124421, 19.14886208192143258 ) ) ;
#30660=CARTESIAN_POINT ( 'NONE',  ( -3.662846001190052991, 218.4274158808045740, 55.10113791807857808 ) ) ;
#30661=CARTESIAN_POINT ( 'NONE',  ( 4.984841277089725686, 213.7757310962907411, 79.55113791807858092 ) ) ;
#30662=CARTESIAN_POINT ( 'NONE',  ( -6.139770520408224463, 198.4640165459539389, 44.04886208192143471 ) ) ;
#30673=CARTESIAN_POINT ( 'NONE',  ( 2.517493886308900919, 214.5937144450984420, 28.40113791807856813 ) ) ;
#30676=CARTESIAN_POINT ( 'NONE',  ( 3.044812012439969795, 216.5253028482143520, 15.39886208192143613 ) ) ;
#30680=CARTESIAN_POINT ( 'NONE',  ( 0.05014649552807626948, 215.4116977939061144, 55.25113791807857666 ) ) ;
#30684=CARTESIAN_POINT ( 'NONE',  ( 8.000000000000008882, 207.0476921513415220, 0.9988620819214347746 ) ) ;
#30686=CARTESIAN_POINT ( 'NONE',  ( 8.118202686958039038, 212.8392687619912635, 46.70113791807857240 ) ) ;
#30688=CARTESIAN_POINT ( 'NONE',  ( -9.984503880673473830, 210.2968891136704315, 15.65113791807856813 ) ) ;
#30689=CARTESIAN_POINT ( 'NONE',  ( 6.220909254589680693, 198.5229672870052582, 100.4488620819214475 ) ) ;
#30693=DIRECTION ( 'NONE',  ( 0.01265860800194867734, -0.08535984102820122488, -0.9962697712884263090 ) ) ;
#30694=CARTESIAN_POINT ( 'NONE',  ( 7.456977232089302632, 217.1783343296989131, 4.551137918078565825 ) ) ;
#30697=CARTESIAN_POINT ( 'NONE',  ( 8.062137200540920645, 201.0835637161417822, 50.30113791807857382 ) ) ;
#30703=CARTESIAN_POINT ( 'NONE',  ( -3.662846001190052991, 218.4274158808045740, 34.10113791807857098 ) ) ;
#30705=CARTESIAN_POINT ( 'NONE',  ( 10.01549611932659545, 203.7984951890123853, 13.14886208192143258 ) ) ;
#30709=CARTESIAN_POINT ( 'NONE',  ( -6.220909254589537696, 198.5229672870051161, 9.051137918078561384 ) ) ;
#30710=CARTESIAN_POINT ( 'NONE',  ( 6.139770520408368348, 198.4640165459539674, 62.45113791807857950 ) ) ;
#30711=( BOUNDED_SURFACE ( )  B_SPLINE_SURFACE ( 3, 2, ( 
 ( #7194, #33080, #14851, #12299, #32572, #6851, #24912, #25077, #4462, #14355, #11635, #11791, #12133, #9750, #9570, #27464, #22184, #14685, #11965, #32914, #1573, #20134, #30529, #22018, #6520, #25413, #17579, #30195, #19632, #16900, #27972, #6688, #32738, #4639, #9242, #30365, #15024, #4296, #17239, #17077, #7027, #17411, #32401, #3954, #27797, #9066, #27298, #24749, #1404, #28319, #41, #12809, #23200, #33254, #12983, #10437, #9920, #28488, #15530, #2086, #31049, #4803, #15196, #25754, #20305, #33594, #12472, #30709, #20809, #23030, #7371, #20477, #25588, #23377, #17750, #2252, #10276, #12633, #28144, #20654, #7546, #22863, #33427, #10100, #30879, #17932, #18092, #7876, #31212, #4977, #15363, #7707, #2426, #5142, #25922, #2594, #30470, #14625, #32674, #1846, #32847, #9681, #12066, #33194, #20240, #32509, #17005, #12575, #9858, #30296, #6789, #4062, #22804, #17177, #9510, #25524, #9340, #20075, #17689, #25178, #1674, #27561, #7132, #6964, #9181, #24846, #14786, #17353, #22454, #17515, #1510, #12236, #30643, #27738, #19897, #30131, #27904, #4401, #2193, #19734, #4227, #7312, #28076, #25021, #22622, #6620, #4738, #14451, #33010, #14962, #4576, #25350, #2020, #12409, #15129, #19570, #29963, #27400, #11907, #22292, #15799, #10541, #23473, #28593, #5414, #8149, #2860, #15474, #140, #31144, #20418, #18532, #26361, #15298, #7474, #5574, #25865, #12751, #301, #30811, #23142, #20922, #33530, #17859, #15632, #2531, #15966, #28914, #10700, #26192, #13244, #10203, #18201, #12914, #2706, #23641, #25690, #22967, #20588, #31315, #21078, #7981, #5077, #30989, #26036, #23310, #18365, #22248, #31482, #3020, #33366, #28257, #10041, #4911, #20747, #7646, #2360, #18028, #28423, #10374, #7810, #5243, #28757, #13084, #14341, #32390, #887, #22007, #29850, #3606, #19446, #29345, #24737, #29675, #11126, #9231, #26609, #3437, #19283, #22169, #11284, #1220, #30011, #21670, #6158, #24564, #11779, #32063, #19114, #9054, #24224, #27286, #6509, #8724, #8887, #16553, #6327, #24053, #16887, #29504, #26947, #3941, #14000, #19621, #1391, #6674, #5992, #32557, #1064, #3272, #13660, #3783, #722, #21501, #31888, #8556, #18950, #16380, #26772, #13834, #24397, #11452, #21831, #32222, #16720, #27122, #14171, #11618, #32725, #19790, #23017, #24898, #1721, #25400, #12121, #4790, #11955, #14837, #33415, #17399, #9392, #27959, #30184, #30517, #7182, #1559, #15183, #10089, #22338, #9909, #7360, #27453, #2072, #6840, #27613, #22679, #17226, #17566, #30866, #4107, #25575, #22512, #4282, #9559, #14673, #28129, #14499, #25067, #4628, #32901, #19951, #9735, #30350, #20466, #12623, #2240, #20291, #17739, #7013, #12287, #27785, #15011, #30697, #4449, #17061, #25236, #12459, #1900, #22851, #33065, #20123, #33243, #7863, #18414, #20797, #8196, #28966, #7531, #25741, #21292, #18581, #5292, #15518, #12797, #31527, #25909, #18248, #523, #7696, #28807, #10748, #26087, #13455, #13131, #5463, #15685, #17917, #33582, #23524, #2755, #31197, #15849, #10261, #192, #5624, #10589, #28637, #5130, #26239, #20966, #10915, #18078, #2582, #16016, #26408, #28, #31360, #15351, #3066, #23188, #12969, #23686, #13295, #347, #21128, #28474, #8029, #2910, #28308, #23848, #4963, #2412, #20638, #31037, #23364, #10425, #14126, #16848, #11572, #24185, #8841, #6113, #29131, #27241, #1351, #24016, #16173, #14290, #3396, #16509, #3895, #11236, #27073, #18745, #26734, #8680, #680, #5779, #21961, #24348, #24692, #21623, #19072, #29298, #29461, #32350, #9014, #31846, #11738, #26908, #26563, #11412, #5950, #847, #31686, #1175, #3233, #3736, #32017, #13790, #3566, #8356, #13956, #18904, #32181, #21788, #1016, #13619, #11082, #19241, #29636, #6283, #19403, #24519, #16340, #29805, #6465, #16676, #21463, #8510, #9864, #25186, #6629, #4745, #22125, #32680, #14793, #17695, #6796, #30477, #25530, #17184, #1681, #20082, #7318, #27567, #14632, #27912, #19743, #22810, #2028, #4234, #4408, #12074, #1854, #19578, #4582, #30139, #22464, #33201, #25029, #15136, #30651, #2199, #1516, #25357, #30304, #12414, #20247, #33018, #29971, #28083, #32515, #17015, #9188, #14969, #27408, #4069, #32855, #14457, #11913, #22299, #24853, #9347, #9518, #22631, #19904, #6971, #17359, #27745, #12244, #7139, #9688, #17523, #7483, #10382, #18539, #12921, #4918, #23481, #25697, #7653, #18035, #28921, #20929, #28430, #10048, #17868, #30997, #20754, #5421, #147, #13091, #18208, #28765, #31489, #26199, #5086, #10549, #31151, #20425, #8157, #15975, #15305, #30818, #5581, #15481, #7819, #26368, #26043, #2714, #28264, #10707, #12581, #2369, #15806, #2867, #22974, #31322, #12758, #23149, #28599, #33537, #7988, #33374, #10211, #21086, #25872, #20595, #2539, #23317, #23648, #14074, #5250, #18373, #15641, #13253, #308, #16302, #29757, #32310, #14082, #6246, #27029, #23976, #31969, #26692, #16464, #29595, #5740, #3027, #3195, #3522, #16633, #969, #18859, #13584, #6070, #3353, #13915, #13744, #3691, #24477, #13413, #21252, #16803, #1138, #807, #11036, #8312, #11532, #21419, #24141, #6422, #638, #24300, #21914, #21576, #8974, #8639, #11369, #11197, #23807, #29092, #19032, #29420, #26865, #21748, #16131, #32138, #19363, #8800, #19197, #31805, #479, #10876, #31645, #8470, #29255, #18705, #26524, #5907, #9476, #1314, #17479, #32472, #22256, #9643, #32977, #20039, #30438, #27363, #27706, #19864, #30606, #12204, #27200, #4031, #4368, #7098, #25142, #9306, #14420 ),
 ( #27864, #12031, #33161, #32810, #14750, #1639, #3856, #19537, #30262, #22419, #17144, #1807, #29931, #6924, #4538, #24989, #4191, #24813, #22591, #27530, #20205, #1475, #11871, #25317, #1982, #19698, #17316, #11702, #14929, #9140, #32643, #12372, #22769, #9824, #7271, #30092, #14248, #24648, #22086, #6584, #16968, #6758, #14590, #5210, #18168, #23272, #106, #3277, #31285, #10164, #28562, #25833, #15092, #13664, #21506, #10000, #2159, #730, #23107, #2496, #24059, #31115, #7777, #25486, #16225, #11131, #12542, #10508, #7945, #28041, #25998, #7438, #28219, #33669, #22932, #15596, #31893, #4702, #26615, #2324, #33327, #20547, #17818, #28722, #20384, #4876, #2669, #15265, #30776, #10344, #30952, #17653, #25657, #5829, #20887, #18327, #12712, #12879, #7614, #13051, #33495, #17998, #28389, #5046, #15437, #20715, #23441, #22176, #32566, #8729, #4114, #19288, #3442, #22013, #16558, #1069, #27459, #11787, #13840, #14348, #11457, #24404, #3612, #24904, #16725, #29510, #9060, #32396, #24571, #1567, #11289, #27128, #21836, #3790, #30018, #24744, #26953, #3948, #9237, #29680, #1399, #21676, #6681, #11627, #26778, #11960, #8562, #19120, #1228, #14506, #14005, #16894, #22344, #32229, #8892, #6515, #18956, #6335, #14177, #19627, #6165, #17068, #29350, #19454, #29857, #27291, #5998, #16385, #24229, #892, #32069, #10095, #1907, #25747, #7538, #2419, #12127, #2247, #7188, #12629, #23024, #9915, #30190, #17925, #12803, #27619, #33421, #4796, #20472, #15358, #27791, #4290, #22520, #32907, #14679, #4970, #15191, #33249, #25073, #1727, #32732, #6846, #17406, #7366, #4455, #30874, #9565, #30523, #9400, #33072, #19959, #20298, #30357, #14844, #25242, #19797, #17745, #12293, #17234, #7021, #22686, #9744, #28136, #20129, #17573, #27966, #4634, #15018, #28314, #25407, #2078, #12466, #22858, #25582, #30703, #7870, #2761, #21134, #8363, #28643, #15690, #28973, #20803, #23855, #3076, #5299, #5470, #13138, #15856, #20646, #5633, #31205, #23531, #530, #26093, #16182, #31693, #26571, #2589, #26415, #31369, #13464, #10923, #356, #31043, #18754, #3240, #18085, #21299, #16024, #29138, #5786, #18254, #28482, #12976, #23372, #5137, #23195, #33589, #23694, #15524, #25916, #10269, #7702, #200, #31533, #10598, #35, #10431, #20974, #8037, #18421, #28813, #10756, #26247, #2918, #13302, #8203, #18588, #19081, #11090, #18912, #32025, #26916, #9023, #687, #8689, #24358, #16347, #21470, #27249, #6291, #29980, #3574, #1025, #11247, #11420, #3904, #14299, #13799, #9196, #21797, #8519, #27082, #21632, #6121, #32523, #16856, #29306, #19412, #16517, #29469, #13963, #6638, #32190, #855, #14134, #3745, #29644, #17023, #26741, #8849, #19249, #16685, #1358, #29814, #24529, #6473, #24701, #1184, #11746, #3403, #22133, #11580, #31854, #27417, #13627, #24193, #21970, #32358, #19586, #24024, #5958, #22473, #2206, #12588, #30313, #20090, #11921, #28091, #9356, #32864, #20256, #9873, #30660, #7327, #4243, #4592, #30485, #7492, #22818, #4077, #12252, #17703, #25365, #14978, #9698, #4754, #22982, #15145, #6980, #2037, #22640, #1525, #33381, #17876, #30148, #22307, #20432, #9526, #33028, #10055, #17533, #27920, #32688, #30825, #14465, #19751, #25538, #24862, #6805, #12424, #27577, #14640, #7148, #17192, #33209, #25037, #1689, #12083, #19913, #17367, #27753, #4417, #14803, #25195, #1863, #28771, #18043, #12766, #20935, #7826, #21257, #23814, #5587, #31495, #18544, #15488, #23487, #18214, #7993, #21093, #31004, #28271, #28436, #5426, #8162, #26205, #10388, #5093, #31327, #28605, #15811, #5256, #28927, #15981, #4926, #23157, #8318, #26373, #26049, #2545, #33544, #3033, #12929, #15650, #31651, #25879, #2873, #13418, #13096, #485, #153, #13258, #2719, #15313, #20602, #10556, #18379, #23654, #313, #7660, #10712, #10882, #25705, #2377, #23324, #10220, #8657, #20761, #31158, #13589, #8805, #32477, #5745, #16810, #3360, #26530, #11202, #8475, #29762, #16137, #18864, #19203, #29262, #3201, #11375, #31976, #11707, #14255, #6428, #21920, #8981, #5913, #13920, #8646, #32143, #11537, #21424, #18712, #16308, #29601, #32315, #16638, #812, #26697, #21754, #19037, #6251, #29426, #19368, #27205, #29097, #23983, #644, #3861, #16471, #13751, #11042, #24654, #24146, #6075, #22092, #21581, #27034, #1319, #3527, #31810, #24305, #3698, #26870, #976, #14088, #24482, #1144, #32816, #20045, #11877, #1814, #20211, #6929, #19871, #6764, #7104, #9481, #2164, #9311, #27535, #7278, #17659, #1645, #25148, #16973, #33167, #14426, #4197, #25322, #14934, #1988, #12377, #19704, #9649, #12209, #12547, #27870, #9146, #17322, #22775, #30444, #17484, #14755, #9831, #28047, #30612, #12038, #4545, #27712, #6590, #4708, #22938, #1481, #27369, #25493, #14597, #4373, #15097, #22596, #32984, #4036, #19543, #29936, #24818, #22262, #32649, #30098, #17149, #24994, #30267, #22425, #31290, #23278, #26332, #33500, #18003, #31453, #8122, #33334, #15601, #25662, #278, #13216, #15443, #26004, #33674, #2676, #30782, #5386, #30959, #10348, #10673, #2501, #2998, #18504, #13377, #12719, #2831, #7782, #23614, #21052, #10513, #7443, #28889, #10006, #28225, #5544, #15771, #15935, #20389, #28394, #4883, #23112, #10172, #15270, #17823, #26164, #111, #2331, #20552, #7619, #5052, #25839, #7951, #12885, #20720, #31119, #18173, #28567, #5215, #13056, #20893, #23446, #18334, #28727, #29723, #32108, #29221, #21217, #29057, #8440, #3321, #19161, #10844, #18827 ),
 ( #8942, #26995, #18666, #29558, #16272, #5873, #26658, #6385, #31935, #11000, #24265, #13882, #6039, #16773, #26492, #8605, #13705, #19002, #11503, #6212, #31774, #16600, #3656, #773, #14050, #3160, #21881, #26827, #8279, #27172, #23775, #16430, #3827, #8771, #441, #29392, #24446, #11333, #935, #3491, #1110, #19332, #32276, #24105, #21718, #31612, #5709, #16097, #13550, #23942, #604, #21380, #11169, #21545, #33124, #27669, #4337, #22055, #12341, #20174, #32439, #7068, #4503, #24617, #22565, #3998, #24786, #19838, #9106, #14721, #28009, #1278, #22737, #32612, #19502, #6727, #14395, #25286, #11672, #1442, #25112, #11837, #29901, #6891, #27501, #7234, #9791, #1952, #17450, #14894, #22222, #9448, #4158, #1773, #27833, #16937, #14219, #9275, #12174, #30572, #32950, #30061, #19669, #17282, #14555, #9611, #24953, #17622, #6554, #27333, #17118, #1611, #12001, #22387, #32776, #30234, #20007, #30407, #15403, #31414, #4844, #25961, #7915, #23240, #10638, #10312, #2636, #12846, #4675, #30746, #20688, #33634, #28359, #15564, #7405, #31087, #15735, #2465, #25801, #2292, #13020, #5013, #8083, #15235, #23071, #2800, #5346, #23412, #9962, #17788, #28687, #20349, #33463, #20852, #10476, #31251, #18295, #25624, #5179, #12676, #76, #26133, #7746, #13182, #28187, #23579, #18131, #22902, #21015, #15060, #10134, #28530, #247, #20516, #18467, #25455, #30919, #17968, #2129, #12513, #7582, #33296, #11137, #21178, #29516, #8733, #10964, #21512, #18794, #31898, #26294, #896, #26455, #29183, #6172, #31736, #21841, #3616, #32232, #8241, #32073, #3284, #19125, #16563, #6003, #2966, #14011, #8898, #23735, #26957, #11296, #24409, #11462, #23904, #401, #18629, #29019, #10804, #1074, #21682, #29355, #31575, #5676, #28853, #13344, #13510, #3450, #569, #5509, #16066, #26620, #15898, #5836, #3121, #16392, #21340, #8408, #16231, #13669, #13846, #24066, #736, #8572, #18962, #26784, #24233, #6339, #14354, #30024, #22017, #27132, #33386, #11964, #2382, #32571, #6687, #16899, #17076, #10060, #20437, #19461, #15318, #27463, #14182, #32737, #27297, #11790, #4932, #22988, #24576, #25546, #22183, #1403, #24748, #12771, #4118, #6519, #19803, #9407, #1572, #23162, #32400, #14510, #9241, #24911, #7499, #2211, #19631, #22348, #30194, #33550, #6850, #3953, #17238, #27626, #4295, #19293, #9065, #15150, #12593, #30833, #17882, #28278, #25711, #29685, #16731, #3794, #1233, #29861, #11634, #13264, #28443, #26536, #10228, #20767, #2880, #5751, #28611, #18549, #13594, #5262, #23493, #8168, #29103, #10394, #20608, #26211, #2551, #10888, #23820, #26054, #23659, #160, #318, #7666, #15987, #7832, #10561, #21263, #13102, #3206, #18718, #23988, #23331, #13423, #18385, #490, #31656, #21100, #18049, #16143, #31011, #5098, #8325, #26378, #15493, #25884, #15656, #12935, #497, #31164, #18220, #2727, #3039, #10717, #20940, #31332, #8000, #28777, #5433, #28934, #15819, #31500, #5594, #32148, #6596, #983, #26703, #11542, #13758, #29431, #6080, #16978, #8986, #16478, #31816, #5918, #19042, #13925, #29769, #21430, #26875, #11380, #3365, #8481, #14260, #27041, #27375, #24312, #21759, #31984, #8809, #24661, #1324, #818, #29941, #19209, #29268, #14094, #8651, #3532, #19547, #3867, #16313, #6435, #24151, #29607, #16816, #27212, #11712, #22097, #11208, #1149, #3705, #4041, #19373, #650, #6256, #32484, #21927, #32319, #16642, #9152, #14431, #11048, #24488, #18871, #21589, #22268, #20395, #28233, #17154, #9317, #7449, #30273, #32990, #10014, #4553, #14940, #32653, #22945, #30788, #19708, #17665, #15106, #1488, #33173, #14603, #1649, #30450, #30106, #25328, #4889, #11882, #33341, #9488, #6769, #17329, #24998, #2170, #27540, #12043, #1995, #22431, #4203, #17490, #4379, #17830, #24824, #12553, #28053, #25500, #32823, #20051, #14761, #12385, #4714, #19877, #6937, #27719, #22782, #25154, #9838, #1822, #12215, #27876, #22603, #20218, #9658, #7111, #30618, #7286, #12728, #26169, #20899, #33679, #28399, #23118, #10518, #5057, #23286, #15776, #30965, #15606, #117, #10353, #5392, #31124, #26010, #20727, #15276, #20560, #18179, #7787, #28572, #2683, #7625, #5221, #31295, #13061, #23451, #15451, #7957, #18340, #25669, #18008, #25845, #28732, #2338, #33505, #2506, #12890, #10178, #25442, #19827, #10124, #17959, #30223, #4833, #2279, #22374, #20336, #1761, #22554, #17610, #6878, #2118, #25789, #32763, #20505, #30393, #17267, #4489, #12161, #23061, #9436, #32939, #12501, #9600, #27656, #4665, #25274, #5003, #7572, #33453, #15224, #12663, #19993, #7221, #1939, #22890, #25613, #14708, #11988, #7055, #33282, #30907, #9949, #27820, #17437, #15049, #12328, #30735, #22724, #28349, #15391, #4324, #25100, #14881, #33112, #9778, #20162, #30559, #27999, #7395, #17776, #28174, #2623, #23726, #5667, #21004, #8398, #8071, #389, #10629, #2455, #28519, #18456, #31402, #26123, #13335, #5168, #28843, #13498, #236, #13171, #66, #10792, #2791, #29174, #13010, #20839, #560, #3109, #21166, #7735, #15554, #26445, #18120, #31242, #18619, #8230, #29006, #16056, #23403, #2956, #5499, #5824, #31563, #12836, #15888, #23892, #10953, #21328, #26282, #31725, #18784, #16218, #28674, #23227, #33623, #10303, #20679, #31077, #25948, #10465, #7904, #18285, #5333, #15724, #23567, #29218, #21878, #19961, #5870, #3824, #18999, #6036, #1107, #24101, #19329, #9746, #16268, #27794, #13879, #3318, #21715, #29389, #7023, #26655, #16427, #29719, #26823 ),
 ( #769, #8939, #3487, #32105, #14846, #32910, #11166, #1729, #8768, #11330, #24262, #12296, #3653, #932, #6382, #16770, #11500, #22688, #31932, #14047, #19158, #24443, #17408, #12129, #29554, #24614, #9567, #6208, #22525, #8602, #4458, #32272, #13702, #33075, #21542, #16597, #27169, #25246, #26991, #14216, #30360, #1911, #33425, #18087, #5302, #20301, #20131, #2423, #12468, #20805, #38, #2249, #12806, #10097, #23197, #17575, #25919, #17747, #20474, #31207, #23026, #13141, #28645, #23534, #33251, #23374, #28316, #10434, #7873, #31046, #27969, #15692, #202, #15021, #18256, #2591, #26096, #2763, #15193, #25410, #9917, #30705, #2082, #30525, #12979, #30876, #7191, #22860, #33591, #4972, #7542, #7704, #7368, #10272, #4636, #17927, #15360, #28140, #28484, #25749, #4800, #25584, #12630, #20651, #5139, #15526, #15859, #13304, #857, #26251, #5636, #26743, #16349, #3405, #13801, #10758, #11092, #3242, #13966, #29309, #10601, #18757, #24195, #31857, #21472, #16184, #11251, #29473, #21635, #3078, #8521, #29141, #8039, #6124, #24362, #2921, #28816, #26919, #16027, #5788, #16520, #24026, #689, #18425, #32028, #5472, #20976, #13629, #8692, #31370, #18914, #358, #21136, #26574, #23696, #5960, #31536, #8205, #19084, #28975, #18590, #13466, #26417, #3577, #23858, #532, #10926, #21301, #31695, #8365, #14302, #27755, #30315, #12086, #4245, #25039, #21973, #29983, #24703, #14467, #27579, #3750, #1030, #1187, #1527, #14643, #32691, #16859, #11583, #4079, #1361, #11924, #11748, #1691, #22476, #11422, #19252, #14805, #32867, #32525, #9025, #6294, #9528, #19414, #22135, #4419, #32361, #22309, #19915, #19589, #6982, #6641, #9359, #9199, #21800, #32192, #17370, #29816, #8852, #27252, #24532, #29647, #16688, #6478, #19754, #3906, #27086, #27419, #17025, #14138, #24864, #30150, #6808, #17194, #12427, #20434, #4757, #4928, #18045, #27922, #25198, #25368, #25708, #28439, #23159, #7329, #2039, #28274, #25542, #2379, #15147, #25881, #12931, #1866, #9700, #5258, #2547, #22985, #33211, #30487, #15490, #9875, #2208, #18216, #22821, #12768, #5095, #10057, #31161, #30828, #33546, #33383, #12255, #17535, #7495, #17879, #12590, #10223, #4595, #15315, #23327, #20605, #31008, #20259, #7662, #5384, #28607, #30662, #17706, #10391, #20763, #7829, #7150, #14981, #22642, #28094, #33031, #20093, #21427, #8478, #18866, #15814, #16139, #8322, #19039, #647, #15652, #23816, #29264, #3203, #26532, #21259, #31813, #815, #5915, #8165, #13591, #487, #13099, #11205, #29428, #7995, #156, #31979, #21096, #10885, #21585, #29100, #5747, #23490, #16310, #10558, #26051, #18715, #26699, #2723, #23985, #5430, #26208, #31653, #20937, #11045, #3362, #31329, #13754, #18381, #24148, #8648, #28773, #2877, #13260, #23656, #315, #10714, #18546, #31497, #28930, #5591, #15984, #26375, #3036, #13420, #22428, #11539, #14257, #24996, #19545, #29939, #13923, #9314, #3529, #6077, #32480, #30101, #16474, #14428, #29604, #16640, #11709, #979, #6593, #19874, #26872, #4200, #24484, #24309, #32317, #6253, #17151, #11377, #27038, #16975, #3701, #21756, #9148, #19370, #32819, #1647, #27537, #19706, #6766, #14091, #1321, #29765, #27371, #32651, #8807, #32145, #1146, #4038, #14600, #24821, #21923, #8983, #1484, #6431, #11879, #16813, #12040, #9484, #19206, #27209, #3863, #24657, #22094, #22264, #1819, #20556, #4549, #7282, #23283, #30447, #17826, #33503, #15101, #2504, #2167, #28228, #4711, #30270, #22598, #12550, #25496, #20215, #7446, #32987, #22942, #7622, #28050, #17662, #27873, #4886, #30615, #33677, #7108, #14937, #28397, #30962, #15273, #12212, #9653, #18006, #20048, #25325, #12724, #2335, #23115, #10175, #17487, #30785, #25151, #5055, #15448, #25843, #12888, #1991, #12381, #22778, #33170, #9835, #10351, #6933, #33338, #25666, #17325, #10010, #4376, #20392, #27716, #14758, #8443, #15604, #18508, #26663, #21058, #13059, #31615, #114, #15774, #26167, #3325, #29061, #2834, #18177, #26008, #5389, #281, #16101, #7785, #13219, #31458, #23449, #28570, #607, #13381, #13709, #10676, #8125, #18338, #28892, #11003, #21383, #20897, #16275, #5547, #2679, #447, #28730, #23618, #5877, #23946, #10516, #26495, #15939, #26336, #3001, #24108, #23778, #7955, #21220, #10848, #8282, #777, #31293, #18669, #5712, #3164, #18830, #13555, #31778, #29224, #20723, #31122, #5219, #13885, #32616, #14222, #29395, #27505, #11172, #21721, #3830, #6731, #29562, #19506, #14559, #6216, #24449, #9109, #30065, #11337, #21548, #27175, #3495, #11841, #24790, #26998, #24620, #1113, #1281, #8609, #16940, #8774, #11506, #22227, #14053, #4164, #19673, #24959, #24268, #14398, #19335, #1447, #9280, #22059, #19005, #17122, #31938, #3659, #938, #6043, #16434, #32111, #11676, #19166, #26830, #32442, #21884, #16603, #32281, #8946, #29726, #6388, #16777, #29904, #6557, #27336, #4002, #4341, #1614, #1777, #2134, #4848, #33301, #17454, #12178, #4679, #1956, #12517, #14898, #2297, #23075, #12005, #19842, #15408, #12681, #33129, #9615, #6895, #25628, #20011, #12345, #28363, #22569, #22907, #15239, #20179, #7587, #7238, #9966, #9796, #22391, #27675, #17626, #30576, #25290, #20354, #14725, #28013, #33468, #15064, #22741, #32954, #30750, #25459, #5017, #30413, #7073, #10138, #20520, #7409, #17288, #25116, #30923, #27837, #4507, #17792, #28191, #17972, #32780, #9453, #30238, #18473, #29188, #10809, #25806, #251, #18634, #13348, #26298, #31419, #8246, #10968 ),
 ( #28857, #16070, #2469, #406, #15568, #2640, #8087, #20692, #15902, #5840, #12851, #23910, #10480, #33638, #2804, #29023, #28535, #13515, #5513, #10317, #8412, #23244, #13025, #2970, #21345, #20857, #21183, #31091, #31255, #5350, #23739, #31740, #25966, #7750, #31580, #18135, #26459, #5680, #7920, #3125, #15741, #573, #5184, #18798, #23416, #26137, #80, #28691, #18300, #13186, #23583, #10642, #21019, #24413, #29864, #19464, #27136, #13673, #24752, #9244, #11141, #6524, #22021, #3957, #32574, #11301, #21516, #29360, #16397, #31902, #22186, #32403, #19130, #11638, #9068, #32078, #24071, #900, #24579, #21686, #14357, #8576, #14015, #19634, #16568, #18966, #3798, #6008, #8737, #29522, #30027, #1237, #6176, #740, #26789, #26961, #3620, #16902, #3289, #1079, #11466, #3454, #13850, #27300, #8904, #16235, #21845, #32238, #24237, #19297, #1407, #11793, #29689, #26626, #6343, #16736, #14185, #14687, #32916, #25591, #9923, #1575, #12475, #9572, #22530, #1736, #23033, #14854, #27630, #7197, #30532, #22695, #33430, #9411, #25251, #19965, #1917, #28148, #22867, #25079, #2089, #20309, #30713, #11967, #12136, #33258, #7374, #17753, #4806, #6853, #17583, #33084, #10103, #25417, #6691, #12302, #15199, #27975, #4642, #9754, #2256, #12637, #20480, #30368, #15027, #20138, #4123, #17079, #27466, #32740, #24914, #14514, #7030, #22351, #19806, #30197, #17242, #4298, #17413, #27799, #4465, #23540, #21592, #7549, #5920, #20657, #7710, #2769, #25758, #21433, #11383, #17935, #29434, #15533, #4980, #23380, #31052, #8653, #28322, #18095, #31818, #28492, #15367, #208, #10440, #24316, #26877, #19044, #820, #31986, #5145, #26101, #20812, #11051, #24154, #33598, #30883, #25925, #8483, #11210, #29270, #12986, #2598, #18874, #31216, #16315, #7880, #6083, #16480, #2429, #12812, #23204, #3534, #28650, #45, #10279, #13927, #18261, #5308, #986, #15699, #26706, #13148, #3368, #13760, #27378, #9321, #29944, #21762, #14097, #4044, #6600, #11715, #32656, #24491, #14434, #32826, #19550, #32487, #19376, #19712, #22100, #14765, #21930, #6438, #19880, #22434, #30109, #27045, #1153, #25158, #11545, #6259, #4382, #27215, #16982, #6942, #1491, #11886, #29611, #25001, #19212, #32152, #24827, #12047, #8812, #6773, #32323, #8989, #22271, #16645, #17157, #1825, #3708, #30276, #16819, #29772, #14263, #3871, #9492, #24664, #1327, #27543, #9155, #4208, #14606, #1652, #17332, #27722, #23290, #15455, #2510, #33176, #7453, #25503, #25674, #5062, #14944, #12218, #12388, #12733, #25849, #10182, #28057, #22785, #15280, #12558, #23122, #2173, #12894, #33683, #22606, #30453, #26015, #10357, #10018, #20222, #17494, #20731, #30621, #22950, #5225, #9841, #33509, #31128, #30792, #18183, #17835, #20565, #20399, #32993, #4556, #28237, #4893, #33346, #30969, #25331, #2343, #7792, #7629, #18012, #7289, #28403, #28576, #15610, #17669, #4717, #9661, #20054, #7114, #27880, #1998, #15109, #7961, #31463, #18836, #8448, #29229, #5883, #2839, #3170, #29065, #6048, #21390, #2687, #10853, #16280, #23951, #13562, #8287, #26668, #21552, #3330, #28897, #612, #21225, #122, #31944, #453, #13715, #24115, #13226, #8615, #13386, #31299, #16106, #10680, #5553, #19011, #782, #18344, #11176, #15946, #18514, #8131, #29400, #31621, #23623, #11010, #26500, #18675, #16440, #5396, #5718, #26343, #31783, #13065, #23455, #21062, #10523, #20903, #23783, #28737, #15779, #26172, #286, #3006, #9458, #26836, #3664, #19513, #22395, #11511, #1452, #30242, #21891, #6394, #24795, #12009, #27004, #3501, #9115, #19172, #27510, #6735, #8951, #29909, #16782, #6562, #24273, #32621, #24456, #27180, #4169, #29733, #19846, #1619, #6900, #6221, #30070, #1288, #17126, #14563, #4007, #943, #32785, #13890, #21726, #24965, #9284, #11344, #32116, #32287, #8779, #16610, #14058, #29568, #1118, #19677, #3836, #22233, #19339, #14228, #24626, #11681, #11845, #22065, #32448, #16946, #27341, #14403, #17631, #9620, #28195, #30418, #12350, #22745, #23248, #25634, #33137, #14730, #22573, #1960, #30581, #12686, #4346, #9800, #28018, #20015, #25120, #30926, #9972, #33641, #7244, #4683, #14903, #2138, #15069, #12523, #5022, #23081, #25294, #33473, #20523, #25463, #10142, #7077, #15412, #20360, #1782, #10321, #17292, #27842, #30754, #12856, #20183, #2301, #20695, #22911, #33305, #15243, #2473, #17459, #27681, #7413, #4512, #17975, #7592, #17797, #4853, #28366, #25809, #12183, #31094, #32958, #8091, #18801, #10647, #743, #16240, #11144, #20861, #10972, #15905, #21348, #31745, #18637, #5187, #26629, #21519, #2643, #8415, #13518, #29193, #7753, #16073, #5844, #3293, #21187, #31584, #15572, #13677, #25970, #18141, #410, #24075, #28539, #26463, #31260, #18304, #13351, #13028, #8249, #23419, #83, #10483, #26140, #7923, #254, #28696, #5354, #15744, #2807, #29027, #13189, #23588, #10812, #21023, #31423, #18477, #28860, #5516, #26303, #2974, #23745, #5684, #3131, #577, #23913, #31906, #32081, #32407, #1410, #29867, #14019, #8743, #1243, #32242, #9073, #11472, #32578, #19640, #8579, #16400, #11970, #9247, #29692, #6182, #3458, #22190, #16573, #8908, #24919, #30030, #11641, #26794, #14518, #18969, #19133, #24583, #27470, #26964, #6527, #1578, #3625, #21850, #16907, #17083, #29526, #29365, #14190, #24240, #6695, #11800, #24417, #22025, #19302, #19468, #6011, #3962, #1082, #6349, #4126, #16740, #13854, #906, #11305, #21689, #27140, #3801, #27303, #14362, #24756 ),
 ( #30200, #7033, #30717, #17417, #10106, #17246, #20141, #28325, #22699, #14690, #33262, #1740, #27802, #4469, #4984, #7377, #14858, #19809, #27634, #25254, #1920, #17756, #9414, #12305, #33089, #25082, #6857, #2260, #15029, #15370, #9757, #30537, #19970, #7201, #12641, #23037, #22534, #17938, #17587, #4302, #2093, #30372, #27978, #7552, #25594, #12139, #28153, #4645, #25421, #12480, #25763, #22870, #9575, #9928, #20313, #4810, #2435, #32919, #15202, #33434, #20483, #30887, #22355, #32744, #8213, #16035, #23543, #5647, #15537, #211, #26425, #25928, #541, #15868, #31056, #29149, #12816, #23383, #5480, #8378, #31220, #21147, #16195, #7884, #26104, #10770, #31705, #12990, #23208, #28823, #5148, #13476, #3088, #28654, #26263, #2772, #2932, #10283, #18600, #10444, #13152, #23869, #15703, #5797, #21310, #26585, #2603, #10934, #20984, #18766, #33604, #23706, #20661, #7713, #18099, #28495, #48, #28987, #20816, #18264, #5314, #10609, #31379, #8051, #18435, #13313, #366, #31544, #32369, #19423, #19092, #11102, #21645, #11592, #32039, #24713, #31866, #1040, #9210, #3585, #29321, #14146, #16357, #8701, #29480, #19600, #21982, #6135, #699, #8530, #16529, #26927, #9033, #24033, #13977, #24374, #5969, #21482, #16868, #29655, #29992, #11431, #21808, #867, #32200, #27261, #3916, #3414, #32534, #8861, #18925, #16697, #11261, #19262, #22144, #6489, #26752, #29828, #6303, #27099, #3761, #6649, #24541, #24204, #1195, #14313, #1369, #17036, #13811, #11758, #3250, #13639, #15160, #33220, #1701, #22829, #30673, #6817, #22489, #32877, #33394, #2050, #9537, #24873, #32703, #12097, #6992, #9885, #14476, #19926, #4427, #30161, #1537, #7339, #20102, #10067, #17379, #14815, #25048, #25210, #17717, #28105, #27588, #22996, #1877, #22317, #7158, #30324, #27763, #12600, #4766, #9370, #20268, #12263, #22655, #33041, #20443, #9712, #14652, #27935, #17544, #30496, #30842, #17204, #4606, #14990, #25379, #25553, #2217, #12438, #7506, #27430, #4087, #11934, #4258, #19764, #20945, #2390, #499, #17891, #28450, #10566, #13431, #2559, #26217, #21270, #12943, #31170, #15826, #3046, #18055, #28285, #167, #10235, #18557, #31506, #6, #31337, #7841, #8007, #15325, #23664, #15499, #18226, #28942, #20774, #10894, #26386, #31665, #31017, #21105, #26064, #8174, #5602, #28784, #25718, #23826, #4940, #12778, #15994, #323, #23168, #33559, #20618, #7673, #5108, #25890, #23341, #10402, #10724, #28617, #13272, #5269, #15662, #2734, #13109, #2886, #23500, #18390, #5440, #6088, #14269, #8659, #657, #19218, #26542, #22107, #8994, #16486, #16320, #13600, #32328, #26711, #19050, #1332, #8490, #29616, #11550, #26884, #24670, #13934, #6264, #3541, #8333, #11059, #24323, #992, #31992, #16654, #21440, #11391, #19382, #21768, #29439, #5927, #27052, #32157, #11720, #18882, #3373, #6444, #29779, #3714, #23994, #31824, #16826, #29275, #13767, #24498, #14103, #1158, #21936, #24161, #8817, #27221, #18725, #3877, #29109, #5758, #16151, #3213, #826, #11217, #21599, #25816, #30934, #17163, #15248, #22441, #19557, #2479, #33647, #4050, #10327, #32493, #12691, #15418, #12861, #28201, #4860, #16990, #7598, #6606, #9162, #25641, #5029, #27384, #33478, #32662, #9327, #17803, #14440, #2307, #29950, #11891, #24833, #32833, #19719, #20366, #4213, #1497, #30116, #1659, #28371, #25007, #6778, #20528, #23089, #22278, #27549, #14611, #12053, #9498, #17980, #30759, #23253, #7418, #10147, #19752, #26917, #27250, #8850, #4244, #19413, #3575, #22134, #16686, #1185, #27578, #11923, #13964, #14466, #11581, #17193, #1690, #24359, #22308, #24863, #30149, #1027, #29471, #21798, #6807, #19250, #11421, #14642, #1526, #21971, #4078, #32689, #24530, #16518, #27083, #17024, #3747, #25038, #32191, #6475, #12084, #9024, #29645, #19587, #6292, #14135, #32359, #22474, #27418, #29815, #6122, #16857, #3905, #14301, #9357, #24702, #1359, #11747, #32524, #9198, #8690, #29981, #19082, #6639, #9874, #19914, #10221, #17369, #17704, #33030, #28437, #20257, #27754, #12589, #7149, #25366, #18044, #2378, #4418, #4927, #2038, #14979, #27921, #15489, #7328, #20092, #33382, #22983, #15146, #25880, #1864, #28092, #12426, #4755, #20603, #15314, #17534, #28273, #12767, #30661, #25706, #12253, #31006, #2207, #14804, #2546, #32865, #9699, #25541, #5094, #4593, #7493, #12930, #22820, #33210, #30826, #9527, #30486, #30314, #10056, #25196, #33545, #23158, #20433, #17877, #7661, #6981, #22641, #29098, #20936, #23655, #645, #26206, #16309, #31811, #26698, #2721, #26531, #31496, #3202, #13590, #486, #20762, #31159, #23984, #7827, #23325, #15982, #11043, #7589, #31652, #13097, #154, #28928, #18215, #13419, #3361, #10389, #21425, #7994, #28606, #15812, #23488, #8476, #5257, #10557, #23815, #31328, #15651, #26374, #2874, #26050, #18865, #29263, #5914, #18380, #28772, #18545, #13259, #3034, #5428, #5746, #16138, #314, #10884, #10713, #21258, #21094, #8164, #8319, #5588, #18713, #27036, #14427, #1483, #13752, #31977, #27536, #24819, #11538, #21755, #19038, #4037, #32144, #24483, #6765, #13921, #1320, #16974, #32316, #19705, #19369, #11708, #21921, #24147, #6076, #29764, #8982, #3699, #24655, #16472, #6429, #11878, #16811, #1145, #11376, #22093, #14089, #17150, #24307, #8806, #22263, #32650, #32479, #29427, #26871, #9312, #3528, #19204, #29937, #19544, #6591, #27370, #977, #14256, #27206, #813, #9147, #11203, #3862, #30099, #21583, #8647, #29602, #6252 ),
 ( #16639, #7106, #30961, #12721, #7621, #17324, #7445, #12380, #17825, #28227, #15100, #1646, #23114, #18005, #32817, #4885, #10008, #25665, #22426, #24995, #27714, #15272, #4375, #19873, #10174, #20391, #17486, #33336, #30784, #20047, #12039, #22597, #12549, #32986, #2333, #9483, #1990, #20555, #4547, #30269, #25495, #14757, #9652, #30446, #4199, #22940, #27872, #6932, #25150, #14936, #25324, #33502, #1816, #22777, #33169, #12211, #9833, #14598, #30614, #20213, #7280, #17661, #28049, #4710, #2166, #13218, #28568, #23944, #5388, #23282, #8124, #2678, #20895, #13552, #31614, #33676, #444, #31292, #10515, #23448, #11002, #2833, #15603, #28891, #18507, #10675, #21382, #31121, #23616, #7953, #280, #16100, #10846, #13058, #23777, #8281, #15773, #21219, #7784, #26494, #31456, #12887, #31776, #28396, #5217, #21054, #606, #113, #3000, #8442, #18336, #28729, #26334, #5054, #26007, #15445, #5546, #20722, #29059, #18668, #26166, #15938, #13380, #5711, #3163, #25841, #18175, #2503, #10350, #8773, #29725, #21547, #11505, #29903, #16602, #29560, #16432, #16776, #19163, #11839, #19004, #3493, #16939, #19505, #6387, #24107, #31937, #9108, #775, #13884, #1280, #24619, #11674, #22057, #29394, #19334, #21883, #22225, #3829, #18829, #26997, #32441, #27174, #14221, #24448, #6556, #4001, #27335, #11336, #14397, #3658, #16274, #24788, #32614, #11171, #29223, #5876, #1444, #26660, #3323, #32278, #8944, #13708, #8608, #6041, #26829, #24267, #937, #21720, #32110, #6214, #14052, #1112, #4160, #33127, #23073, #30063, #7407, #27672, #17120, #1775, #32778, #20352, #6729, #9451, #9793, #19840, #27503, #1954, #22567, #2294, #4846, #30748, #12515, #33298, #30236, #4505, #32952, #22739, #14557, #15062, #25457, #25626, #20176, #22904, #7236, #25114, #6893, #12343, #9613, #30574, #20009, #9964, #17790, #9278, #24956, #19671, #28189, #7070, #17284, #1613, #15237, #4339, #30410, #12678, #14723, #17624, #12003, #27835, #22389, #14896, #28011, #12176, #17452, #25288, #4677, #2132, #18133, #8085, #3123, #28532, #13023, #31416, #18631, #33636, #33466, #15738, #25803, #403, #13346, #15566, #26135, #23414, #2802, #30921, #5511, #31089, #78, #10806, #2638, #26457, #8243, #13512, #12849, #2968, #7917, #23737, #21181, #10640, #7585, #29021, #10136, #28361, #31578, #15900, #5678, #17970, #20518, #23242, #16068, #10315, #15405, #5015, #26296, #10478, #28855, #2467, #25964, #20690, #5181, #18471, #20854, #7748, #31253, #18297, #28689, #5348, #13184, #21016, #23581, #249, #29358, #29863, #32234, #6005, #21342, #29185, #8574, #3452, #19295, #10966, #18964, #898, #26623, #31738, #3797, #16566, #6522, #13848, #11298, #8410, #1235, #18796, #8735, #24068, #19463, #21684, #5838, #3618, #31900, #16394, #9067, #27134, #16233, #29687, #26786, #24235, #32076, #16901, #19127, #11139, #24411, #14013, #6174, #27299, #3286, #29518, #26959, #1077, #11636, #6341, #11464, #16733, #14184, #21843, #24578, #13671, #22019, #8900, #738, #32402, #3955, #21514, #23907, #571, #14686, #25414, #17240, #7372, #22864, #17751, #27465, #17580, #22529, #27973, #4640, #25249, #11792, #33255, #28145, #9243, #15025, #20135, #2087, #32573, #1405, #4120, #12473, #14512, #30026, #20306, #30530, #27628, #9751, #7195, #30196, #22185, #32739, #22692, #9409, #9921, #19633, #12134, #30710, #25078, #6689, #1915, #24913, #19805, #6852, #14356, #33081, #4297, #17078, #1574, #1734, #32915, #24750, #11966, #9571, #19964, #22350, #30366, #7028, #17412, #27798, #4463, #14852, #12300, #15863, #23031, #23378, #4978, #362, #15531, #33428, #18259, #12810, #31050, #23700, #8042, #10101, #10605, #7708, #20655, #33595, #21140, #12984, #25755, #5305, #28648, #20810, #31540, #7547, #42, #18093, #10438, #26256, #20979, #23201, #205, #18429, #25923, #31374, #17933, #2925, #7877, #20478, #8208, #4804, #15364, #31213, #10762, #10277, #13145, #18594, #28489, #5143, #2767, #15197, #2427, #25589, #15697, #30880, #5475, #28819, #2595, #26099, #23538, #13308, #2253, #12634, #28320, #32363, #13633, #8525, #26922, #14141, #29144, #28980, #11255, #21304, #29650, #8855, #11095, #21638, #18917, #32033, #26420, #1034, #26580, #29315, #6297, #31860, #21977, #3754, #9028, #8370, #32195, #3408, #19255, #16692, #6127, #3083, #24536, #5640, #23863, #27090, #11426, #1190, #13470, #16030, #18760, #11587, #5792, #10929, #535, #21803, #5964, #24365, #31699, #21476, #16188, #24028, #3580, #693, #3245, #16352, #26746, #13805, #24198, #861, #16524, #8696, #19087, #29475, #13971, #28234, #24867, #16862, #24707, #4082, #32695, #15277, #6481, #14471, #30154, #22139, #27255, #33506, #12554, #2507, #9363, #6812, #3910, #30966, #14307, #4249, #19593, #15452, #17199, #1364, #33342, #27424, #11929, #5058, #23119, #11752, #25671, #22312, #1529, #19758, #12891, #27583, #6644, #20396, #10015, #1696, #23287, #32527, #14647, #25043, #22947, #7626, #2339, #30789, #12729, #10179, #7450, #20562, #9204, #18009, #17832, #29986, #33680, #19418, #17030, #4890, #28400, #25846, #29819, #31125, #5393, #21060, #13062, #18180, #23948, #3003, #26665, #23620, #31461, #7788, #21385, #28573, #28894, #10519, #5881, #8128, #5222, #23780, #18341, #2836, #29226, #13559, #15607, #16103, #13222, #26170, #15777, #3327, #18510, #31296, #10850, #450, #26339, #13712, #23452, #5549, #284, #15942, #31780, #26497, #28734, #5715, #609, #13383, #3167, #119, #8445, #21222, #26012, #24111, #10354 ) ),
 .UNSPECIFIED., .T., .F., .T. ) 
 B_SPLINE_SURFACE_WITH_KNOTS ( ( 4, 3, 4 ),
 ( 3, 2, 2, 2, 2, 2, 2, 2, 2, 2, 2, 2, 2, 2, 2, 2, 2, 2, 2, 2, 2, 2, 2, 2, 2, 2, 2, 2, 2, 2, 2, 2, 2, 2, 2, 2, 2, 2, 2, 2, 2, 2, 2, 2, 2, 2, 2, 2, 2, 2, 2, 2, 2, 2, 2, 2, 2, 2, 2, 2, 2, 2, 2, 2, 2, 2, 2, 2, 2, 2, 2, 2, 2, 2, 2, 2, 2, 2, 2, 2, 2, 2, 2, 2, 2, 2, 2, 2, 2, 2, 2, 2, 2, 2, 2, 2, 2, 2, 2, 2, 2, 2, 2, 2, 2, 2, 2, 2, 2, 2, 2, 2, 2, 2, 2, 2, 2, 2, 2, 2, 2, 2, 2, 2, 2, 2, 2, 2, 2, 2, 2, 2, 2, 2, 2, 2, 2, 2, 2, 2, 2, 2, 2, 2, 2, 2, 2, 2, 2, 2, 2, 2, 2, 2, 2, 2, 2, 2, 2, 2, 2, 2, 2, 2, 2, 2, 2, 2, 2, 2, 2, 2, 2, 2, 2, 2, 2, 2, 2, 2, 2, 2, 2, 2, 2, 2, 2, 2, 2, 2, 2, 2, 2, 2, 2, 2, 2, 2, 2, 2, 2, 2, 2, 2, 2, 2, 2, 2, 2, 2, 2, 2, 2, 2, 2, 2, 2, 2, 2, 2, 2, 2, 2, 2, 2, 2, 2, 2, 2, 2, 2, 2, 2, 2, 2, 2, 2, 2, 2, 2, 2, 2, 2, 2, 2, 2, 2, 2, 2, 2, 2, 2, 2, 2, 2, 2, 2, 2, 2, 2, 2, 2, 2, 2, 2, 2, 2, 2, 2, 2, 2, 2, 2, 2, 2, 2, 2, 2, 2, 2, 2, 2, 2, 2, 2, 2, 2, 2, 2, 2, 2, 2, 2, 2, 2, 2, 2, 2, 2, 2, 2, 2, 2, 2, 2, 2, 2, 2, 2, 2, 2, 2, 2, 2, 2, 2, 2, 2, 2, 2, 2, 2, 2, 2, 2, 2, 2, 2, 2, 2, 2, 2, 2, 2, 2, 2, 2, 2, 2, 2, 2, 2, 2, 2, 2, 2, 3 ),
 ( 0.000000000000000000, 0.5000000000000000000, 1.000000000000000000 ),
 ( 0.000000000000000000, 0.002857142857142857140, 0.005714285714285714281, 0.008571428571428571855, 0.01142857142857142856, 0.01428571428571428527, 0.01714285714285714371, 0.02000000000000000042, 0.02285714285714285712, 0.02571428571428571383, 0.02857142857142857054, 0.03142857142857143071, 0.03428571428571428742, 0.03714285714285714413, 0.04000000000000000083, 0.04285714285714285754, 0.04571428571428571425, 0.04857142857142857095, 0.05142857142857142766, 0.05428571428571428437, 0.05714285714285714107, 0.05999999999999999778, 0.06285714285714286143, 0.06571428571428571119, 0.06857142857142857484, 0.07142857142857142461, 0.07428571428571428825, 0.07714285714285713802, 0.08000000000000000167, 0.08285714285714285143, 0.08571428571428571508, 0.08857142857142856485, 0.09142857142857142849, 0.09428571428571429214, 0.09714285714285714191, 0.1000000000000000056, 0.1028571428571428553, 0.1057142857142857190, 0.1085714285714285687, 0.1114285714285714324, 0.1142857142857142821, 0.1171428571428571458, 0.1199999999999999956, 0.1228571428571428592, 0.1257142857142857229, 0.1285714285714285587, 0.1314285714285714224, 0.1342857142857142860, 0.1371428571428571497, 0.1400000000000000133, 0.1428571428571428492, 0.1457142857142857129, 0.1485714285714285765, 0.1514285714285714401, 0.1542857142857142760, 0.1571428571428571397, 0.1600000000000000033, 0.1628571428571428670, 0.1657142857142857029, 0.1685714285714285665, 0.1714285714285714302, 0.1742857142857142938, 0.1771428571428571297, 0.1799999999999999933, 0.1828571428571428570, 0.1857142857142857206, 0.1885714285714285843, 0.1914285714285714202, 0.1942857142857142838, 0.1971428571428571475, 0.2000000000000000111, 0.2028571428571428470, 0.2057142857142857106, 0.2085714285714285743, 0.2114285714285714379, 0.2142857142857142738, 0.2171428571428571375, 0.2200000000000000011, 0.2228571428571428648, 0.2257142857142857006, 0.2285714285714285643, 0.2314285714285714279, 0.2342857142857142916, 0.2371428571428571552, 0.2399999999999999911, 0.2428571428571428548, 0.2457142857142857184, 0.2485714285714285821, 0.2514285714285714457, 0.2542857142857142816, 0.2571428571428571175, 0.2600000000000000089, 0.2628571428571428448, 0.2657142857142857362, 0.2685714285714285721, 0.2714285714285714080, 0.2742857142857142994, 0.2771428571428571352, 0.2800000000000000266, 0.2828571428571428625, 0.2857142857142856984, 0.2885714285714285898, 0.2914285714285714257, 0.2942857142857142616, 0.2971428571428571530, 0.2999999999999999889, 0.3028571428571428803, 0.3057142857142857162, 0.3085714285714285521, 0.3114285714285714435, 0.3142857142857142794, 0.3171428571428571153, 0.3200000000000000067, 0.3228571428571428426, 0.3257142857142857340, 0.3285714285714285698, 0.3314285714285714057, 0.3342857142857142971, 0.3371428571428571330, 0.3400000000000000244, 0.3428571428571428603, 0.3457142857142856962, 0.3485714285714285876, 0.3514285714285714235, 0.3542857142857142594, 0.3571428571428571508, 0.3599999999999999867, 0.3628571428571428781, 0.3657142857142857140, 0.3685714285714285499, 0.3714285714285714413, 0.3742857142857142771, 0.3771428571428571686, 0.3800000000000000044, 0.3828571428571428403, 0.3857142857142857317, 0.3885714285714285676, 0.3914285714285714035, 0.3942857142857142949, 0.3971428571428571308, 0.4000000000000000222, 0.4028571428571428581, 0.4057142857142856940, 0.4085714285714285854, 0.4114285714285714213, 0.4142857142857143127, 0.4171428571428571486, 0.4199999999999999845, 0.4228571428571428759, 0.4257142857142857117, 0.4285714285714285476, 0.4314285714285714390, 0.4342857142857142749, 0.4371428571428571663, 0.4400000000000000022, 0.4428571428571428381, 0.4457142857142857295, 0.4485714285714285654, 0.4514285714285714013, 0.4542857142857142927, 0.4571428571428571286, 0.4600000000000000200, 0.4628571428571428559, 0.4657142857142856918, 0.4685714285714285832, 0.4714285714285714191, 0.4742857142857143105, 0.4771428571428571463, 0.4799999999999999822, 0.4828571428571428736, 0.4857142857142857095, 0.4885714285714285454, 0.4914285714285714368, 0.4942857142857142727, 0.4971428571428571641, 0.5000000000000000000, 0.5028571428571428914, 0.5057142857142856718, 0.5085714285714285632, 0.5114285714285714546, 0.5142857142857142350, 0.5171428571428571264, 0.5200000000000000178, 0.5228571428571429092, 0.5257142857142856895, 0.5285714285714285809, 0.5314285714285714723, 0.5342857142857142527, 0.5371428571428571441, 0.5400000000000000355, 0.5428571428571428159, 0.5457142857142857073, 0.5485714285714285987, 0.5514285714285713791, 0.5542857142857142705, 0.5571428571428571619, 0.5600000000000000533, 0.5628571428571428337, 0.5657142857142857251, 0.5685714285714286165, 0.5714285714285713969, 0.5742857142857142883, 0.5771428571428571797, 0.5799999999999999600, 0.5828571428571428514, 0.5857142857142857428, 0.5885714285714285232, 0.5914285714285714146, 0.5942857142857143060, 0.5971428571428571974, 0.5999999999999999778, 0.6028571428571428692, 0.6057142857142857606, 0.6085714285714285410, 0.6114285714285714324, 0.6142857142857143238, 0.6171428571428571042, 0.6199999999999999956, 0.6228571428571428870, 0.6257142857142856673, 0.6285714285714285587, 0.6314285714285714501, 0.6342857142857142305, 0.6371428571428571219, 0.6400000000000000133, 0.6428571428571429047, 0.6457142857142856851, 0.6485714285714285765, 0.6514285714285714679, 0.6542857142857142483, 0.6571428571428571397, 0.6600000000000000311, 0.6628571428571428115, 0.6657142857142857029, 0.6685714285714285943, 0.6714285714285713746, 0.6742857142857142660, 0.6771428571428571574, 0.6800000000000000488, 0.6828571428571428292, 0.6857142857142857206, 0.6885714285714286120, 0.6914285714285713924, 0.6942857142857142838, 0.6971428571428571752, 0.6999999999999999556, 0.7028571428571428470, 0.7057142857142857384, 0.7085714285714285188, 0.7114285714285714102, 0.7142857142857143016, 0.7171428571428571930, 0.7199999999999999734, 0.7228571428571428648, 0.7257142857142857562, 0.7285714285714285365, 0.7314285714285714279, 0.7342857142857143193, 0.7371428571428570997, 0.7399999999999999911, 0.7428571428571428825, 0.7457142857142856629, 0.7485714285714285543, 0.7514285714285714457, 0.7542857142857143371, 0.7571428571428571175, 0.7600000000000000089, 0.7628571428571429003, 0.7657142857142856807, 0.7685714285714285721, 0.7714285714285714635, 0.7742857142857142438, 0.7771428571428571352, 0.7800000000000000266, 0.7828571428571428070, 0.7857142857142856984, 0.7885714285714285898, 0.7914285714285714812, 0.7942857142857142616, 0.7971428571428571530, 0.8000000000000000444, 0.8028571428571428248, 0.8057142857142857162, 0.8085714285714286076, 0.8114285714285713880, 0.8142857142857142794, 0.8171428571428571708, 0.8199999999999999512, 0.8228571428571428426, 0.8257142857142857340, 0.8285714285714286254, 0.8314285714285714057, 0.8342857142857142971, 0.8371428571428571885, 0.8399999999999999689, 0.8428571428571428603, 0.8457142857142857517, 0.8485714285714285321, 0.8514285714285714235, 0.8542857142857143149, 0.8571428571428570953, 0.8599999999999999867, 0.8628571428571428781, 0.8657142857142857695, 0.8685714285714285499, 0.8714285714285714413, 0.8742857142857143327, 0.8771428571428571130, 0.8800000000000000044, 0.8828571428571428958, 0.8857142857142856762, 0.8885714285714285676, 0.8914285714285714590, 0.8942857142857142394, 0.8971428571428571308, 0.9000000000000000222, 0.9028571428571428026, 0.9057142857142856940, 0.9085714285714285854, 0.9114285714285714768, 0.9142857142857142572, 0.9171428571428571486, 0.9200000000000000400, 0.9228571428571428203, 0.9257142857142857117, 0.9285714285714286031, 0.9314285714285713835, 0.9342857142857142749, 0.9371428571428571663, 0.9399999999999999467, 0.9428571428571428381, 0.9457142857142857295, 0.9485714285714286209, 0.9514285714285714013, 0.9542857142857142927, 0.9571428571428571841, 0.9599999999999999645, 0.9628571428571428559, 0.9657142857142857473, 0.9685714285714285277, 0.9714285714285714191, 0.9742857142857143105, 0.9771428571428570908, 0.9799999999999999822, 0.9828571428571428736, 0.9857142857142857650, 0.9955714285714286627 ),
 .UNSPECIFIED. ) 
 GEOMETRIC_REPRESENTATION_ITEM ( )  RATIONAL_B_SPLINE_SURFACE ( (
 ( 1.000000000000000000, 0.9510565162951535312, 1.000000000000000000, 0.9510565162951535312, 1.000000000000000000, 0.9510565162951535312, 1.000000000000000000, 0.9510565162951535312, 1.000000000000000000, 0.9510565162951535312, 1.000000000000000000, 0.9510565162951535312, 1.000000000000000000, 0.9510565162951535312, 1.000000000000000000, 0.9510565162951535312, 1.000000000000000000, 0.9510565162951535312, 1.000000000000000000, 0.9510565162951535312, 1.000000000000000000, 0.9510565162951535312, 1.000000000000000000, 0.9510565162951535312, 1.000000000000000000, 0.9510565162951535312, 1.000000000000000000, 0.9510565162951535312, 1.000000000000000000, 0.9510565162951535312, 1.000000000000000000, 0.9510565162951535312, 1.000000000000000000, 0.9510565162951535312, 1.000000000000000000, 0.9510565162951535312, 1.000000000000000000, 0.9510565162951535312, 1.000000000000000000, 0.9510565162951535312, 1.000000000000000000, 0.9510565162951535312, 1.000000000000000000, 0.9510565162951535312, 1.000000000000000000, 0.9510565162951535312, 1.000000000000000000, 0.9510565162951535312, 1.000000000000000000, 0.9510565162951535312, 1.000000000000000000, 0.9510565162951535312, 1.000000000000000000, 0.9510565162951535312, 1.000000000000000000, 0.9510565162951535312, 1.000000000000000000, 0.9510565162951535312, 1.000000000000000000, 0.9510565162951535312, 1.000000000000000000, 0.9510565162951535312, 1.000000000000000000, 0.9510565162951535312, 1.000000000000000000, 0.9510565162951535312, 1.000000000000000000, 0.9510565162951535312, 1.000000000000000000, 0.9510565162951535312, 1.000000000000000000, 0.9510565162951535312, 1.000000000000000000, 0.9510565162951535312, 1.000000000000000000, 0.9510565162951535312, 1.000000000000000000, 0.9510565162951535312, 1.000000000000000000, 0.9510565162951535312, 1.000000000000000000, 0.9510565162951535312, 1.000000000000000000, 0.9510565162951535312, 1.000000000000000000, 0.9510565162951535312, 1.000000000000000000, 0.9510565162951535312, 1.000000000000000000, 0.9510565162951535312, 1.000000000000000000, 0.9510565162951535312, 1.000000000000000000, 0.9510565162951535312, 1.000000000000000000, 0.9510565162951535312, 1.000000000000000000, 0.9510565162951535312, 1.000000000000000000, 0.9510565162951535312, 1.000000000000000000, 0.9510565162951535312, 1.000000000000000000, 0.9510565162951535312, 1.000000000000000000, 0.9510565162951535312, 1.000000000000000000, 0.9510565162951535312, 1.000000000000000000, 0.9510565162951535312, 1.000000000000000000, 0.9510565162951535312, 1.000000000000000000, 0.9510565162951535312, 1.000000000000000000, 0.9510565162951535312, 1.000000000000000000, 0.9510565162951535312, 1.000000000000000000, 0.9510565162951535312, 1.000000000000000000, 0.9510565162951535312, 1.000000000000000000, 0.9510565162951535312, 1.000000000000000000, 0.9510565162951535312, 1.000000000000000000, 0.9510565162951535312, 1.000000000000000000, 0.9510565162951535312, 1.000000000000000000, 0.9510565162951535312, 1.000000000000000000, 0.9510565162951535312, 1.000000000000000000, 0.9510565162951535312, 1.000000000000000000, 0.9510565162951535312, 1.000000000000000000, 0.9510565162951535312, 1.000000000000000000, 0.9510565162951535312, 1.000000000000000000, 0.9510565162951535312, 1.000000000000000000, 0.9510565162951535312, 1.000000000000000000, 0.9510565162951535312, 1.000000000000000000, 0.9510565162951535312, 1.000000000000000000, 0.9510565162951535312, 1.000000000000000000, 0.9510565162951535312, 1.000000000000000000, 0.9510565162951535312, 1.000000000000000000, 0.9510565162951535312, 1.000000000000000000, 0.9510565162951535312, 1.000000000000000000, 0.9510565162951535312, 1.000000000000000000, 0.9510565162951535312, 1.000000000000000000, 0.9510565162951535312, 1.000000000000000000, 0.9510565162951535312, 1.000000000000000000, 0.9510565162951535312, 1.000000000000000000, 0.9510565162951535312, 1.000000000000000000, 0.9510565162951535312, 1.000000000000000000, 0.9510565162951535312, 1.000000000000000000, 0.9510565162951535312, 1.000000000000000000, 0.9510565162951535312, 1.000000000000000000, 0.9510565162951535312, 1.000000000000000000, 0.9510565162951535312, 1.000000000000000000, 0.9510565162951535312, 1.000000000000000000, 0.9510565162951535312, 1.000000000000000000, 0.9510565162951535312, 1.000000000000000000, 0.9510565162951535312, 1.000000000000000000, 0.9510565162951535312, 1.000000000000000000, 0.9510565162951535312, 1.000000000000000000, 0.9510565162951535312, 1.000000000000000000, 0.9510565162951535312, 1.000000000000000000, 0.9510565162951535312, 1.000000000000000000, 0.9510565162951535312, 1.000000000000000000, 0.9510565162951535312, 1.000000000000000000, 0.9510565162951535312, 1.000000000000000000, 0.9510565162951535312, 1.000000000000000000, 0.9510565162951535312, 1.000000000000000000, 0.9510565162951535312, 1.000000000000000000, 0.9510565162951535312, 1.000000000000000000, 0.9510565162951535312, 1.000000000000000000, 0.9510565162951535312, 1.000000000000000000, 0.9510565162951535312, 1.000000000000000000, 0.9510565162951535312, 1.000000000000000000, 0.9510565162951535312, 1.000000000000000000, 0.9510565162951535312, 1.000000000000000000, 0.9510565162951535312, 1.000000000000000000, 0.9510565162951535312, 1.000000000000000000, 0.9510565162951535312, 1.000000000000000000, 0.9510565162951535312, 1.000000000000000000, 0.9510565162951535312, 1.000000000000000000, 0.9510565162951535312, 1.000000000000000000, 0.9510565162951535312, 1.000000000000000000, 0.9510565162951535312, 1.000000000000000000, 0.9510565162951535312, 1.000000000000000000, 0.9510565162951535312, 1.000000000000000000, 0.9510565162951535312, 1.000000000000000000, 0.9510565162951535312, 1.000000000000000000, 0.9510565162951535312, 1.000000000000000000, 0.9510565162951535312, 1.000000000000000000, 0.9510565162951535312, 1.000000000000000000, 0.9510565162951535312, 1.000000000000000000, 0.9510565162951535312, 1.000000000000000000, 0.9510565162951535312, 1.000000000000000000, 0.9510565162951535312, 1.000000000000000000, 0.9510565162951535312, 1.000000000000000000, 0.9510565162951535312, 1.000000000000000000, 0.9510565162951535312, 1.000000000000000000, 0.9510565162951535312, 1.000000000000000000, 0.9510565162951535312, 1.000000000000000000, 0.9510565162951535312, 1.000000000000000000, 0.9510565162951535312, 1.000000000000000000, 0.9510565162951535312, 1.000000000000000000, 0.9510565162951535312, 1.000000000000000000, 0.9510565162951535312, 1.000000000000000000, 0.9510565162951535312, 1.000000000000000000, 0.9510565162951535312, 1.000000000000000000, 0.9510565162951535312, 1.000000000000000000, 0.9510565162951535312, 1.000000000000000000, 0.9510565162951535312, 1.000000000000000000, 0.9510565162951535312, 1.000000000000000000, 0.9510565162951535312, 1.000000000000000000, 0.9510565162951535312, 1.000000000000000000, 0.9510565162951535312, 1.000000000000000000, 0.9510565162951535312, 1.000000000000000000, 0.9510565162951535312, 1.000000000000000000, 0.9510565162951535312, 1.000000000000000000, 0.9510565162951535312, 1.000000000000000000, 0.9510565162951535312, 1.000000000000000000, 0.9510565162951535312, 1.000000000000000000, 0.9510565162951535312, 1.000000000000000000, 0.9510565162951535312, 1.000000000000000000, 0.9510565162951535312, 1.000000000000000000, 0.9510565162951535312, 1.000000000000000000, 0.9510565162951535312, 1.000000000000000000, 0.9510565162951535312, 1.000000000000000000, 0.9510565162951535312, 1.000000000000000000, 0.9510565162951535312, 1.000000000000000000, 0.9510565162951535312, 1.000000000000000000, 0.9510565162951535312, 1.000000000000000000, 0.9510565162951535312, 1.000000000000000000, 0.9510565162951535312, 1.000000000000000000, 0.9510565162951535312, 1.000000000000000000, 0.9510565162951535312, 1.000000000000000000, 0.9510565162951535312, 1.000000000000000000, 0.9510565162951535312, 1.000000000000000000, 0.9510565162951535312, 1.000000000000000000, 0.9510565162951535312, 1.000000000000000000, 0.9510565162951535312, 1.000000000000000000, 0.9510565162951535312, 1.000000000000000000, 0.9510565162951535312, 1.000000000000000000, 0.9510565162951535312, 1.000000000000000000, 0.9510565162951535312, 1.000000000000000000, 0.9510565162951535312, 1.000000000000000000, 0.9510565162951535312, 1.000000000000000000, 0.9510565162951535312, 1.000000000000000000, 0.9510565162951535312, 1.000000000000000000, 0.9510565162951535312, 1.000000000000000000, 0.9510565162951535312, 1.000000000000000000, 0.9510565162951535312, 1.000000000000000000, 0.9510565162951535312, 1.000000000000000000, 0.9510565162951535312, 1.000000000000000000, 0.9510565162951535312, 1.000000000000000000, 0.9510565162951535312, 1.000000000000000000, 0.9510565162951535312, 1.000000000000000000, 0.9510565162951535312, 1.000000000000000000, 0.9510565162951535312, 1.000000000000000000, 0.9510565162951535312, 1.000000000000000000, 0.9510565162951535312, 1.000000000000000000, 0.9510565162951535312, 1.000000000000000000, 0.9510565162951535312, 1.000000000000000000, 0.9510565162951535312, 1.000000000000000000, 0.9510565162951535312, 1.000000000000000000, 0.9510565162951535312, 1.000000000000000000, 0.9510565162951535312, 1.000000000000000000, 0.9510565162951535312, 1.000000000000000000, 0.9510565162951535312, 1.000000000000000000, 0.9510565162951535312, 1.000000000000000000, 0.9510565162951535312, 1.000000000000000000, 0.9510565162951535312, 1.000000000000000000, 0.9510565162951535312, 1.000000000000000000, 0.9510565162951535312, 1.000000000000000000, 0.9510565162951535312, 1.000000000000000000, 0.9510565162951535312, 1.000000000000000000, 0.9510565162951535312, 1.000000000000000000, 0.9510565162951535312, 1.000000000000000000, 0.9510565162951535312, 1.000000000000000000, 0.9510565162951535312, 1.000000000000000000, 0.9510565162951535312, 1.000000000000000000, 0.9510565162951535312, 1.000000000000000000, 0.9510565162951535312, 1.000000000000000000, 0.9510565162951535312, 1.000000000000000000, 0.9510565162951535312, 1.000000000000000000, 0.9510565162951535312, 1.000000000000000000, 0.9510565162951535312, 1.000000000000000000, 0.9510565162951535312, 1.000000000000000000, 0.9510565162951535312, 1.000000000000000000, 0.9510565162951535312, 1.000000000000000000, 0.9510565162951535312, 1.000000000000000000, 0.9510565162951535312, 1.000000000000000000, 0.9510565162951535312, 1.000000000000000000, 0.9510565162951535312, 1.000000000000000000, 0.9510565162951535312, 1.000000000000000000, 0.9510565162951535312, 1.000000000000000000, 0.9510565162951535312, 1.000000000000000000, 0.9510565162951535312, 1.000000000000000000, 0.9510565162951535312, 1.000000000000000000, 0.9510565162951535312, 1.000000000000000000, 0.9510565162951535312, 1.000000000000000000, 0.9510565162951535312, 1.000000000000000000, 0.9510565162951535312, 1.000000000000000000, 0.9510565162951535312, 1.000000000000000000, 0.9510565162951535312, 1.000000000000000000, 0.9510565162951535312, 1.000000000000000000, 0.9510565162951535312, 1.000000000000000000, 0.9510565162951535312, 1.000000000000000000, 0.9510565162951535312, 1.000000000000000000, 0.9510565162951535312, 1.000000000000000000, 0.9510565162951535312, 1.000000000000000000, 0.9510565162951535312, 1.000000000000000000, 0.9510565162951535312, 1.000000000000000000, 0.9510565162951535312, 1.000000000000000000, 0.9510565162951535312, 1.000000000000000000, 0.9510565162951535312, 1.000000000000000000, 0.9510565162951535312, 1.000000000000000000, 0.9510565162951535312, 1.000000000000000000, 0.9510565162951535312, 1.000000000000000000, 0.9510565162951535312, 1.000000000000000000, 0.9510565162951535312, 1.000000000000000000, 0.9510565162951535312, 1.000000000000000000, 0.9510565162951535312, 1.000000000000000000, 0.9510565162951535312, 1.000000000000000000, 0.9510565162951535312, 1.000000000000000000, 0.9510565162951535312, 1.000000000000000000, 0.9510565162951535312, 1.000000000000000000, 0.9510565162951535312, 1.000000000000000000, 0.9510565162951535312, 1.000000000000000000, 0.9510565162951535312, 1.000000000000000000, 0.9510565162951535312, 1.000000000000000000, 0.9510565162951535312, 1.000000000000000000, 0.9510565162951535312, 1.000000000000000000, 0.9510565162951535312, 1.000000000000000000, 0.9510565162951535312, 1.000000000000000000, 0.9510565162951535312, 1.000000000000000000, 0.9510565162951535312, 1.000000000000000000, 0.9510565162951535312, 1.000000000000000000, 0.9510565162951535312, 1.000000000000000000, 0.9510565162951535312, 1.000000000000000000, 0.9510565162951535312, 1.000000000000000000, 0.9510565162951535312, 1.000000000000000000, 0.9510565162951535312, 1.000000000000000000, 0.9510565162951535312, 1.000000000000000000, 0.9510565162951535312, 1.000000000000000000, 0.9510565162951535312, 1.000000000000000000, 0.9510565162951535312, 1.000000000000000000, 0.9510565162951535312, 1.000000000000000000, 0.9510565162951535312, 1.000000000000000000, 0.9510565162951535312, 1.000000000000000000, 0.9510565162951535312, 1.000000000000000000, 0.9510565162951535312, 1.000000000000000000, 0.9510565162951535312, 1.000000000000000000, 0.9510565162951535312, 1.000000000000000000, 0.9510565162951535312, 1.000000000000000000, 0.9510565162951535312, 1.000000000000000000, 0.9510565162951535312, 1.000000000000000000, 0.9510565162951535312, 1.000000000000000000, 0.9510565162951535312, 1.000000000000000000, 0.9510565162951535312, 1.000000000000000000, 0.9510565162951535312, 1.000000000000000000, 0.9510565162951535312, 1.000000000000000000, 0.9510565162951535312, 1.000000000000000000, 0.9510565162951535312, 1.000000000000000000, 0.9510565162951535312, 1.000000000000000000, 0.9510565162951535312, 1.000000000000000000, 0.9510565162951535312, 1.000000000000000000, 0.9510565162951535312, 1.000000000000000000, 0.9510565162951535312, 1.000000000000000000, 0.9510565162951535312, 1.000000000000000000, 0.9510565162951535312, 1.000000000000000000, 0.9510565162951535312, 1.000000000000000000, 0.9510565162951535312, 1.000000000000000000, 0.9510565162951535312, 1.000000000000000000, 0.9510565162951535312, 1.000000000000000000, 0.9510565162951535312, 1.000000000000000000, 0.9510565162951535312, 1.000000000000000000, 0.9510565162951535312, 1.000000000000000000, 0.9510565162951535312, 1.000000000000000000, 0.9510565162951535312, 1.000000000000000000, 0.9510565162951535312, 1.000000000000000000, 0.9510565162951535312, 1.000000000000000000, 0.9510565162951535312, 1.000000000000000000, 0.9510565162951535312, 1.000000000000000000, 0.9510565162951535312, 1.000000000000000000, 0.9510565162951535312, 1.000000000000000000, 0.9510565162951535312, 1.000000000000000000, 0.9510565162951535312, 1.000000000000000000, 0.9510565162951535312, 1.000000000000000000, 0.9510565162951535312, 1.000000000000000000, 0.9510565162951535312, 1.000000000000000000, 0.9510565162951535312, 1.000000000000000000, 0.9510565162951535312, 1.000000000000000000, 0.9510565162951535312, 1.000000000000000000, 0.9510565162951535312, 1.000000000000000000, 0.9510565162951535312, 1.000000000000000000, 0.9510565162951535312, 1.000000000000000000, 0.9510565162951535312, 1.000000000000000000, 0.9510565162951535312, 1.000000000000000000, 0.9510565162951535312, 1.000000000000000000, 0.9510565162951535312, 1.000000000000000000, 0.9510565162951535312, 1.000000000000000000, 0.9510565162951535312, 1.000000000000000000, 0.9510565162951535312, 1.000000000000000000, 0.9510565162951535312, 1.000000000000000000, 0.9510565162951535312, 1.000000000000000000, 0.9510565162951535312, 1.000000000000000000, 0.9510565162951535312, 1.000000000000000000, 0.9510565162951535312, 1.000000000000000000, 1.000000000000000000, 1.000000000000000000),
 ( 0.3333333333333333703, 0.3170188387650512141, 0.3333333333333333703, 0.3170188387650512141, 0.3333333333333333703, 0.3170188387650512141, 0.3333333333333333703, 0.3170188387650512141, 0.3333333333333333703, 0.3170188387650512141, 0.3333333333333333703, 0.3170188387650512141, 0.3333333333333333703, 0.3170188387650512141, 0.3333333333333333703, 0.3170188387650512141, 0.3333333333333333703, 0.3170188387650512141, 0.3333333333333333703, 0.3170188387650512141, 0.3333333333333333703, 0.3170188387650512141, 0.3333333333333333703, 0.3170188387650512141, 0.3333333333333333703, 0.3170188387650512141, 0.3333333333333333703, 0.3170188387650512141, 0.3333333333333333703, 0.3170188387650512141, 0.3333333333333333703, 0.3170188387650512141, 0.3333333333333333703, 0.3170188387650512141, 0.3333333333333333703, 0.3170188387650512141, 0.3333333333333333703, 0.3170188387650512141, 0.3333333333333333703, 0.3170188387650512141, 0.3333333333333333703, 0.3170188387650512141, 0.3333333333333333703, 0.3170188387650512141, 0.3333333333333333703, 0.3170188387650512141, 0.3333333333333333703, 0.3170188387650512141, 0.3333333333333333703, 0.3170188387650512141, 0.3333333333333333703, 0.3170188387650512141, 0.3333333333333333703, 0.3170188387650512141, 0.3333333333333333703, 0.3170188387650512141, 0.3333333333333333703, 0.3170188387650512141, 0.3333333333333333703, 0.3170188387650512141, 0.3333333333333333703, 0.3170188387650512141, 0.3333333333333333703, 0.3170188387650512141, 0.3333333333333333703, 0.3170188387650512141, 0.3333333333333333703, 0.3170188387650512141, 0.3333333333333333703, 0.3170188387650512141, 0.3333333333333333703, 0.3170188387650512141, 0.3333333333333333703, 0.3170188387650512141, 0.3333333333333333703, 0.3170188387650512141, 0.3333333333333333703, 0.3170188387650512141, 0.3333333333333333703, 0.3170188387650512141, 0.3333333333333333703, 0.3170188387650512141, 0.3333333333333333703, 0.3170188387650512141, 0.3333333333333333703, 0.3170188387650512141, 0.3333333333333333703, 0.3170188387650512141, 0.3333333333333333703, 0.3170188387650512141, 0.3333333333333333703, 0.3170188387650512141, 0.3333333333333333703, 0.3170188387650512141, 0.3333333333333333703, 0.3170188387650512141, 0.3333333333333333703, 0.3170188387650512141, 0.3333333333333333703, 0.3170188387650512141, 0.3333333333333333703, 0.3170188387650512141, 0.3333333333333333703, 0.3170188387650512141, 0.3333333333333333703, 0.3170188387650512141, 0.3333333333333333703, 0.3170188387650512141, 0.3333333333333333703, 0.3170188387650512141, 0.3333333333333333703, 0.3170188387650512141, 0.3333333333333333703, 0.3170188387650512141, 0.3333333333333333703, 0.3170188387650512141, 0.3333333333333333703, 0.3170188387650512141, 0.3333333333333333703, 0.3170188387650512141, 0.3333333333333333703, 0.3170188387650512141, 0.3333333333333333703, 0.3170188387650512141, 0.3333333333333333703, 0.3170188387650512141, 0.3333333333333333703, 0.3170188387650512141, 0.3333333333333333703, 0.3170188387650512141, 0.3333333333333333703, 0.3170188387650512141, 0.3333333333333333703, 0.3170188387650512141, 0.3333333333333333703, 0.3170188387650512141, 0.3333333333333333703, 0.3170188387650512141, 0.3333333333333333703, 0.3170188387650512141, 0.3333333333333333703, 0.3170188387650512141, 0.3333333333333333703, 0.3170188387650512141, 0.3333333333333333703, 0.3170188387650512141, 0.3333333333333333703, 0.3170188387650512141, 0.3333333333333333703, 0.3170188387650512141, 0.3333333333333333703, 0.3170188387650512141, 0.3333333333333333703, 0.3170188387650512141, 0.3333333333333333703, 0.3170188387650512141, 0.3333333333333333703, 0.3170188387650512141, 0.3333333333333333703, 0.3170188387650512141, 0.3333333333333333703, 0.3170188387650512141, 0.3333333333333333703, 0.3170188387650512141, 0.3333333333333333703, 0.3170188387650512141, 0.3333333333333333703, 0.3170188387650512141, 0.3333333333333333703, 0.3170188387650512141, 0.3333333333333333703, 0.3170188387650512141, 0.3333333333333333703, 0.3170188387650512141, 0.3333333333333333703, 0.3170188387650512141, 0.3333333333333333703, 0.3170188387650512141, 0.3333333333333333703, 0.3170188387650512141, 0.3333333333333333703, 0.3170188387650512141, 0.3333333333333333703, 0.3170188387650512141, 0.3333333333333333703, 0.3170188387650512141, 0.3333333333333333703, 0.3170188387650512141, 0.3333333333333333703, 0.3170188387650512141, 0.3333333333333333703, 0.3170188387650512141, 0.3333333333333333703, 0.3170188387650512141, 0.3333333333333333703, 0.3170188387650512141, 0.3333333333333333703, 0.3170188387650512141, 0.3333333333333333703, 0.3170188387650512141, 0.3333333333333333703, 0.3170188387650512141, 0.3333333333333333703, 0.3170188387650512141, 0.3333333333333333703, 0.3170188387650512141, 0.3333333333333333703, 0.3170188387650512141, 0.3333333333333333703, 0.3170188387650512141, 0.3333333333333333703, 0.3170188387650512141, 0.3333333333333333703, 0.3170188387650512141, 0.3333333333333333703, 0.3170188387650512141, 0.3333333333333333703, 0.3170188387650512141, 0.3333333333333333703, 0.3170188387650512141, 0.3333333333333333703, 0.3170188387650512141, 0.3333333333333333703, 0.3170188387650512141, 0.3333333333333333703, 0.3170188387650512141, 0.3333333333333333703, 0.3170188387650512141, 0.3333333333333333703, 0.3170188387650512141, 0.3333333333333333703, 0.3170188387650512141, 0.3333333333333333703, 0.3170188387650512141, 0.3333333333333333703, 0.3170188387650512141, 0.3333333333333333703, 0.3170188387650512141, 0.3333333333333333703, 0.3170188387650512141, 0.3333333333333333703, 0.3170188387650512141, 0.3333333333333333703, 0.3170188387650512141, 0.3333333333333333703, 0.3170188387650512141, 0.3333333333333333703, 0.3170188387650512141, 0.3333333333333333703, 0.3170188387650512141, 0.3333333333333333703, 0.3170188387650512141, 0.3333333333333333703, 0.3170188387650512141, 0.3333333333333333703, 0.3170188387650512141, 0.3333333333333333703, 0.3170188387650512141, 0.3333333333333333703, 0.3170188387650512141, 0.3333333333333333703, 0.3170188387650512141, 0.3333333333333333703, 0.3170188387650512141, 0.3333333333333333703, 0.3170188387650512141, 0.3333333333333333703, 0.3170188387650512141, 0.3333333333333333703, 0.3170188387650512141, 0.3333333333333333703, 0.3170188387650512141, 0.3333333333333333703, 0.3170188387650512141, 0.3333333333333333703, 0.3170188387650512141, 0.3333333333333333703, 0.3170188387650512141, 0.3333333333333333703, 0.3170188387650512141, 0.3333333333333333703, 0.3170188387650512141, 0.3333333333333333703, 0.3170188387650512141, 0.3333333333333333703, 0.3170188387650512141, 0.3333333333333333703, 0.3170188387650512141, 0.3333333333333333703, 0.3170188387650512141, 0.3333333333333333703, 0.3170188387650512141, 0.3333333333333333703, 0.3170188387650512141, 0.3333333333333333703, 0.3170188387650512141, 0.3333333333333333703, 0.3170188387650512141, 0.3333333333333333703, 0.3170188387650512141, 0.3333333333333333703, 0.3170188387650512141, 0.3333333333333333703, 0.3170188387650512141, 0.3333333333333333703, 0.3170188387650512141, 0.3333333333333333703, 0.3170188387650512141, 0.3333333333333333703, 0.3170188387650512141, 0.3333333333333333703, 0.3170188387650512141, 0.3333333333333333703, 0.3170188387650512141, 0.3333333333333333703, 0.3170188387650512141, 0.3333333333333333703, 0.3170188387650512141, 0.3333333333333333703, 0.3170188387650512141, 0.3333333333333333703, 0.3170188387650512141, 0.3333333333333333703, 0.3170188387650512141, 0.3333333333333333703, 0.3170188387650512141, 0.3333333333333333703, 0.3170188387650512141, 0.3333333333333333703, 0.3170188387650512141, 0.3333333333333333703, 0.3170188387650512141, 0.3333333333333333703, 0.3170188387650512141, 0.3333333333333333703, 0.3170188387650512141, 0.3333333333333333703, 0.3170188387650512141, 0.3333333333333333703, 0.3170188387650512141, 0.3333333333333333703, 0.3170188387650512141, 0.3333333333333333703, 0.3170188387650512141, 0.3333333333333333703, 0.3170188387650512141, 0.3333333333333333703, 0.3170188387650512141, 0.3333333333333333703, 0.3170188387650512141, 0.3333333333333333703, 0.3170188387650512141, 0.3333333333333333703, 0.3170188387650512141, 0.3333333333333333703, 0.3170188387650512141, 0.3333333333333333703, 0.3170188387650512141, 0.3333333333333333703, 0.3170188387650512141, 0.3333333333333333703, 0.3170188387650512141, 0.3333333333333333703, 0.3170188387650512141, 0.3333333333333333703, 0.3170188387650512141, 0.3333333333333333703, 0.3170188387650512141, 0.3333333333333333703, 0.3170188387650512141, 0.3333333333333333703, 0.3170188387650512141, 0.3333333333333333703, 0.3170188387650512141, 0.3333333333333333703, 0.3170188387650512141, 0.3333333333333333703, 0.3170188387650512141, 0.3333333333333333703, 0.3170188387650512141, 0.3333333333333333703, 0.3170188387650512141, 0.3333333333333333703, 0.3170188387650512141, 0.3333333333333333703, 0.3170188387650512141, 0.3333333333333333703, 0.3170188387650512141, 0.3333333333333333703, 0.3170188387650512141, 0.3333333333333333703, 0.3170188387650512141, 0.3333333333333333703, 0.3170188387650512141, 0.3333333333333333703, 0.3170188387650512141, 0.3333333333333333703, 0.3170188387650512141, 0.3333333333333333703, 0.3170188387650512141, 0.3333333333333333703, 0.3170188387650512141, 0.3333333333333333703, 0.3170188387650512141, 0.3333333333333333703, 0.3170188387650512141, 0.3333333333333333703, 0.3170188387650512141, 0.3333333333333333703, 0.3170188387650512141, 0.3333333333333333703, 0.3170188387650512141, 0.3333333333333333703, 0.3170188387650512141, 0.3333333333333333703, 0.3170188387650512141, 0.3333333333333333703, 0.3170188387650512141, 0.3333333333333333703, 0.3170188387650512141, 0.3333333333333333703, 0.3170188387650512141, 0.3333333333333333703, 0.3170188387650512141, 0.3333333333333333703, 0.3170188387650512141, 0.3333333333333333703, 0.3170188387650512141, 0.3333333333333333703, 0.3170188387650512141, 0.3333333333333333703, 0.3170188387650512141, 0.3333333333333333703, 0.3170188387650512141, 0.3333333333333333703, 0.3170188387650512141, 0.3333333333333333703, 0.3170188387650512141, 0.3333333333333333703, 0.3170188387650512141, 0.3333333333333333703, 0.3170188387650512141, 0.3333333333333333703, 0.3170188387650512141, 0.3333333333333333703, 0.3170188387650512141, 0.3333333333333333703, 0.3170188387650512141, 0.3333333333333333703, 0.3170188387650512141, 0.3333333333333333703, 0.3170188387650512141, 0.3333333333333333703, 0.3170188387650512141, 0.3333333333333333703, 0.3170188387650512141, 0.3333333333333333703, 0.3170188387650512141, 0.3333333333333333703, 0.3170188387650512141, 0.3333333333333333703, 0.3170188387650512141, 0.3333333333333333703, 0.3170188387650512141, 0.3333333333333333703, 0.3170188387650512141, 0.3333333333333333703, 0.3170188387650512141, 0.3333333333333333703, 0.3170188387650512141, 0.3333333333333333703, 0.3170188387650512141, 0.3333333333333333703, 0.3170188387650512141, 0.3333333333333333703, 0.3170188387650512141, 0.3333333333333333703, 0.3170188387650512141, 0.3333333333333333703, 0.3170188387650512141, 0.3333333333333333703, 0.3170188387650512141, 0.3333333333333333703, 0.3170188387650512141, 0.3333333333333333703, 0.3170188387650512141, 0.3333333333333333703, 0.3170188387650512141, 0.3333333333333333703, 0.3170188387650512141, 0.3333333333333333703, 0.3170188387650512141, 0.3333333333333333703, 0.3170188387650512141, 0.3333333333333333703, 0.3170188387650512141, 0.3333333333333333703, 0.3170188387650512141, 0.3333333333333333703, 0.3170188387650512141, 0.3333333333333333703, 0.3170188387650512141, 0.3333333333333333703, 0.3170188387650512141, 0.3333333333333333703, 0.3170188387650512141, 0.3333333333333333703, 0.3170188387650512141, 0.3333333333333333703, 0.3170188387650512141, 0.3333333333333333703, 0.3170188387650512141, 0.3333333333333333703, 0.3170188387650512141, 0.3333333333333333703, 0.3170188387650512141, 0.3333333333333333703, 0.3170188387650512141, 0.3333333333333333703, 0.3170188387650512141, 0.3333333333333333703, 0.3170188387650512141, 0.3333333333333333703, 0.3170188387650512141, 0.3333333333333333703, 0.3170188387650512141, 0.3333333333333333703, 0.3170188387650512141, 0.3333333333333333703, 0.3170188387650512141, 0.3333333333333333703, 0.3170188387650512141, 0.3333333333333333703, 0.3170188387650512141, 0.3333333333333333703, 0.3170188387650512141, 0.3333333333333333703, 0.3170188387650512141, 0.3333333333333333703, 0.3170188387650512141, 0.3333333333333333703, 0.3170188387650512141, 0.3333333333333333703, 0.3170188387650512141, 0.3333333333333333703, 0.3170188387650512141, 0.3333333333333333703, 0.3170188387650512141, 0.3333333333333333703, 0.3170188387650512141, 0.3333333333333333703, 0.3170188387650512141, 0.3333333333333333703, 0.3170188387650512141, 0.3333333333333333703, 0.3170188387650512141, 0.3333333333333333703, 0.3170188387650512141, 0.3333333333333333703, 0.3170188387650512141, 0.3333333333333333703, 0.3170188387650512141, 0.3333333333333333703, 0.3170188387650512141, 0.3333333333333333703, 0.3170188387650512141, 0.3333333333333333703, 0.3170188387650512141, 0.3333333333333333703, 0.3170188387650512141, 0.3333333333333333703, 0.3170188387650512141, 0.3333333333333333703, 0.3170188387650512141, 0.3333333333333333703, 0.3170188387650512141, 0.3333333333333333703, 0.3170188387650512141, 0.3333333333333333703, 0.3170188387650512141, 0.3333333333333333703, 0.3170188387650512141, 0.3333333333333333703, 0.3170188387650512141, 0.3333333333333333703, 0.3170188387650512141, 0.3333333333333333703, 0.3170188387650512141, 0.3333333333333333703, 0.3170188387650512141, 0.3333333333333333703, 0.3170188387650512141, 0.3333333333333333703, 0.3170188387650512141, 0.3333333333333333703, 0.3170188387650512141, 0.3333333333333333703, 0.3170188387650512141, 0.3333333333333333703, 0.3170188387650512141, 0.3333333333333333703, 0.3170188387650512141, 0.3333333333333333703, 0.3170188387650512141, 0.3333333333333333703, 0.3170188387650512141, 0.3333333333333333703, 0.3170188387650512141, 0.3333333333333333703, 0.3170188387650512141, 0.3333333333333333703, 0.3170188387650512141, 0.3333333333333333703, 0.3170188387650512141, 0.3333333333333333703, 0.3170188387650512141, 0.3333333333333333703, 0.3170188387650512141, 0.3333333333333333703, 0.3170188387650512141, 0.3333333333333333703, 0.3170188387650512141, 0.3333333333333333703, 0.3170188387650512141, 0.3333333333333333703, 0.3170188387650512141, 0.3333333333333333703, 0.3170188387650512141, 0.3333333333333333703, 0.3170188387650512141, 0.3333333333333333703, 0.3170188387650512141, 0.3333333333333333703, 0.3170188387650512141, 0.3333333333333333703, 0.3170188387650512141, 0.3333333333333333703, 0.3170188387650512141, 0.3333333333333333703, 0.3170188387650512141, 0.3333333333333333703, 0.3170188387650512141, 0.3333333333333333703, 0.3170188387650512141, 0.3333333333333333703, 0.3170188387650512141, 0.3333333333333333703, 0.3170188387650512141, 0.3333333333333333703, 0.3170188387650512141, 0.3333333333333333703, 0.3170188387650512141, 0.3333333333333333703, 0.3170188387650512141, 0.3333333333333333703, 0.3170188387650512141, 0.3333333333333333703, 0.3170188387650512141, 0.3333333333333333703, 0.3170188387650512141, 0.3333333333333333703, 0.3170188387650512141, 0.3333333333333333703, 0.3170188387650512141, 0.3333333333333333703, 0.3170188387650512141, 0.3333333333333333703, 0.3170188387650512141, 0.3333333333333333703, 0.3170188387650512141, 0.3333333333333333703, 0.3170188387650512141, 0.3333333333333333703, 0.3170188387650512141, 0.3333333333333333703, 0.3170188387650512141, 0.3333333333333333703, 0.3170188387650512141, 0.3333333333333333703, 0.3170188387650512141, 0.3333333333333333703, 0.3170188387650512141, 0.3333333333333333703, 0.3170188387650512141, 0.3333333333333333703, 0.3170188387650512141, 0.3333333333333333703, 0.3170188387650512141, 0.3333333333333333703, 0.3170188387650512141, 0.3333333333333333703, 0.3333333333333333703, 0.3333333333333333703),
 ( 0.3333333333333333703, 0.3170188387650512141, 0.3333333333333333703, 0.3170188387650512141, 0.3333333333333333703, 0.3170188387650512141, 0.3333333333333333703, 0.3170188387650512141, 0.3333333333333333703, 0.3170188387650512141, 0.3333333333333333703, 0.3170188387650512141, 0.3333333333333333703, 0.3170188387650512141, 0.3333333333333333703, 0.3170188387650512141, 0.3333333333333333703, 0.3170188387650512141, 0.3333333333333333703, 0.3170188387650512141, 0.3333333333333333703, 0.3170188387650512141, 0.3333333333333333703, 0.3170188387650512141, 0.3333333333333333703, 0.3170188387650512141, 0.3333333333333333703, 0.3170188387650512141, 0.3333333333333333703, 0.3170188387650512141, 0.3333333333333333703, 0.3170188387650512141, 0.3333333333333333703, 0.3170188387650512141, 0.3333333333333333703, 0.3170188387650512141, 0.3333333333333333703, 0.3170188387650512141, 0.3333333333333333703, 0.3170188387650512141, 0.3333333333333333703, 0.3170188387650512141, 0.3333333333333333703, 0.3170188387650512141, 0.3333333333333333703, 0.3170188387650512141, 0.3333333333333333703, 0.3170188387650512141, 0.3333333333333333703, 0.3170188387650512141, 0.3333333333333333703, 0.3170188387650512141, 0.3333333333333333703, 0.3170188387650512141, 0.3333333333333333703, 0.3170188387650512141, 0.3333333333333333703, 0.3170188387650512141, 0.3333333333333333703, 0.3170188387650512141, 0.3333333333333333703, 0.3170188387650512141, 0.3333333333333333703, 0.3170188387650512141, 0.3333333333333333703, 0.3170188387650512141, 0.3333333333333333703, 0.3170188387650512141, 0.3333333333333333703, 0.3170188387650512141, 0.3333333333333333703, 0.3170188387650512141, 0.3333333333333333703, 0.3170188387650512141, 0.3333333333333333703, 0.3170188387650512141, 0.3333333333333333703, 0.3170188387650512141, 0.3333333333333333703, 0.3170188387650512141, 0.3333333333333333703, 0.3170188387650512141, 0.3333333333333333703, 0.3170188387650512141, 0.3333333333333333703, 0.3170188387650512141, 0.3333333333333333703, 0.3170188387650512141, 0.3333333333333333703, 0.3170188387650512141, 0.3333333333333333703, 0.3170188387650512141, 0.3333333333333333703, 0.3170188387650512141, 0.3333333333333333703, 0.3170188387650512141, 0.3333333333333333703, 0.3170188387650512141, 0.3333333333333333703, 0.3170188387650512141, 0.3333333333333333703, 0.3170188387650512141, 0.3333333333333333703, 0.3170188387650512141, 0.3333333333333333703, 0.3170188387650512141, 0.3333333333333333703, 0.3170188387650512141, 0.3333333333333333703, 0.3170188387650512141, 0.3333333333333333703, 0.3170188387650512141, 0.3333333333333333703, 0.3170188387650512141, 0.3333333333333333703, 0.3170188387650512141, 0.3333333333333333703, 0.3170188387650512141, 0.3333333333333333703, 0.3170188387650512141, 0.3333333333333333703, 0.3170188387650512141, 0.3333333333333333703, 0.3170188387650512141, 0.3333333333333333703, 0.3170188387650512141, 0.3333333333333333703, 0.3170188387650512141, 0.3333333333333333703, 0.3170188387650512141, 0.3333333333333333703, 0.3170188387650512141, 0.3333333333333333703, 0.3170188387650512141, 0.3333333333333333703, 0.3170188387650512141, 0.3333333333333333703, 0.3170188387650512141, 0.3333333333333333703, 0.3170188387650512141, 0.3333333333333333703, 0.3170188387650512141, 0.3333333333333333703, 0.3170188387650512141, 0.3333333333333333703, 0.3170188387650512141, 0.3333333333333333703, 0.3170188387650512141, 0.3333333333333333703, 0.3170188387650512141, 0.3333333333333333703, 0.3170188387650512141, 0.3333333333333333703, 0.3170188387650512141, 0.3333333333333333703, 0.3170188387650512141, 0.3333333333333333703, 0.3170188387650512141, 0.3333333333333333703, 0.3170188387650512141, 0.3333333333333333703, 0.3170188387650512141, 0.3333333333333333703, 0.3170188387650512141, 0.3333333333333333703, 0.3170188387650512141, 0.3333333333333333703, 0.3170188387650512141, 0.3333333333333333703, 0.3170188387650512141, 0.3333333333333333703, 0.3170188387650512141, 0.3333333333333333703, 0.3170188387650512141, 0.3333333333333333703, 0.3170188387650512141, 0.3333333333333333703, 0.3170188387650512141, 0.3333333333333333703, 0.3170188387650512141, 0.3333333333333333703, 0.3170188387650512141, 0.3333333333333333703, 0.3170188387650512141, 0.3333333333333333703, 0.3170188387650512141, 0.3333333333333333703, 0.3170188387650512141, 0.3333333333333333703, 0.3170188387650512141, 0.3333333333333333703, 0.3170188387650512141, 0.3333333333333333703, 0.3170188387650512141, 0.3333333333333333703, 0.3170188387650512141, 0.3333333333333333703, 0.3170188387650512141, 0.3333333333333333703, 0.3170188387650512141, 0.3333333333333333703, 0.3170188387650512141, 0.3333333333333333703, 0.3170188387650512141, 0.3333333333333333703, 0.3170188387650512141, 0.3333333333333333703, 0.3170188387650512141, 0.3333333333333333703, 0.3170188387650512141, 0.3333333333333333703, 0.3170188387650512141, 0.3333333333333333703, 0.3170188387650512141, 0.3333333333333333703, 0.3170188387650512141, 0.3333333333333333703, 0.3170188387650512141, 0.3333333333333333703, 0.3170188387650512141, 0.3333333333333333703, 0.3170188387650512141, 0.3333333333333333703, 0.3170188387650512141, 0.3333333333333333703, 0.3170188387650512141, 0.3333333333333333703, 0.3170188387650512141, 0.3333333333333333703, 0.3170188387650512141, 0.3333333333333333703, 0.3170188387650512141, 0.3333333333333333703, 0.3170188387650512141, 0.3333333333333333703, 0.3170188387650512141, 0.3333333333333333703, 0.3170188387650512141, 0.3333333333333333703, 0.3170188387650512141, 0.3333333333333333703, 0.3170188387650512141, 0.3333333333333333703, 0.3170188387650512141, 0.3333333333333333703, 0.3170188387650512141, 0.3333333333333333703, 0.3170188387650512141, 0.3333333333333333703, 0.3170188387650512141, 0.3333333333333333703, 0.3170188387650512141, 0.3333333333333333703, 0.3170188387650512141, 0.3333333333333333703, 0.3170188387650512141, 0.3333333333333333703, 0.3170188387650512141, 0.3333333333333333703, 0.3170188387650512141, 0.3333333333333333703, 0.3170188387650512141, 0.3333333333333333703, 0.3170188387650512141, 0.3333333333333333703, 0.3170188387650512141, 0.3333333333333333703, 0.3170188387650512141, 0.3333333333333333703, 0.3170188387650512141, 0.3333333333333333703, 0.3170188387650512141, 0.3333333333333333703, 0.3170188387650512141, 0.3333333333333333703, 0.3170188387650512141, 0.3333333333333333703, 0.3170188387650512141, 0.3333333333333333703, 0.3170188387650512141, 0.3333333333333333703, 0.3170188387650512141, 0.3333333333333333703, 0.3170188387650512141, 0.3333333333333333703, 0.3170188387650512141, 0.3333333333333333703, 0.3170188387650512141, 0.3333333333333333703, 0.3170188387650512141, 0.3333333333333333703, 0.3170188387650512141, 0.3333333333333333703, 0.3170188387650512141, 0.3333333333333333703, 0.3170188387650512141, 0.3333333333333333703, 0.3170188387650512141, 0.3333333333333333703, 0.3170188387650512141, 0.3333333333333333703, 0.3170188387650512141, 0.3333333333333333703, 0.3170188387650512141, 0.3333333333333333703, 0.3170188387650512141, 0.3333333333333333703, 0.3170188387650512141, 0.3333333333333333703, 0.3170188387650512141, 0.3333333333333333703, 0.3170188387650512141, 0.3333333333333333703, 0.3170188387650512141, 0.3333333333333333703, 0.3170188387650512141, 0.3333333333333333703, 0.3170188387650512141, 0.3333333333333333703, 0.3170188387650512141, 0.3333333333333333703, 0.3170188387650512141, 0.3333333333333333703, 0.3170188387650512141, 0.3333333333333333703, 0.3170188387650512141, 0.3333333333333333703, 0.3170188387650512141, 0.3333333333333333703, 0.3170188387650512141, 0.3333333333333333703, 0.3170188387650512141, 0.3333333333333333703, 0.3170188387650512141, 0.3333333333333333703, 0.3170188387650512141, 0.3333333333333333703, 0.3170188387650512141, 0.3333333333333333703, 0.3170188387650512141, 0.3333333333333333703, 0.3170188387650512141, 0.3333333333333333703, 0.3170188387650512141, 0.3333333333333333703, 0.3170188387650512141, 0.3333333333333333703, 0.3170188387650512141, 0.3333333333333333703, 0.3170188387650512141, 0.3333333333333333703, 0.3170188387650512141, 0.3333333333333333703, 0.3170188387650512141, 0.3333333333333333703, 0.3170188387650512141, 0.3333333333333333703, 0.3170188387650512141, 0.3333333333333333703, 0.3170188387650512141, 0.3333333333333333703, 0.3170188387650512141, 0.3333333333333333703, 0.3170188387650512141, 0.3333333333333333703, 0.3170188387650512141, 0.3333333333333333703, 0.3170188387650512141, 0.3333333333333333703, 0.3170188387650512141, 0.3333333333333333703, 0.3170188387650512141, 0.3333333333333333703, 0.3170188387650512141, 0.3333333333333333703, 0.3170188387650512141, 0.3333333333333333703, 0.3170188387650512141, 0.3333333333333333703, 0.3170188387650512141, 0.3333333333333333703, 0.3170188387650512141, 0.3333333333333333703, 0.3170188387650512141, 0.3333333333333333703, 0.3170188387650512141, 0.3333333333333333703, 0.3170188387650512141, 0.3333333333333333703, 0.3170188387650512141, 0.3333333333333333703, 0.3170188387650512141, 0.3333333333333333703, 0.3170188387650512141, 0.3333333333333333703, 0.3170188387650512141, 0.3333333333333333703, 0.3170188387650512141, 0.3333333333333333703, 0.3170188387650512141, 0.3333333333333333703, 0.3170188387650512141, 0.3333333333333333703, 0.3170188387650512141, 0.3333333333333333703, 0.3170188387650512141, 0.3333333333333333703, 0.3170188387650512141, 0.3333333333333333703, 0.3170188387650512141, 0.3333333333333333703, 0.3170188387650512141, 0.3333333333333333703, 0.3170188387650512141, 0.3333333333333333703, 0.3170188387650512141, 0.3333333333333333703, 0.3170188387650512141, 0.3333333333333333703, 0.3170188387650512141, 0.3333333333333333703, 0.3170188387650512141, 0.3333333333333333703, 0.3170188387650512141, 0.3333333333333333703, 0.3170188387650512141, 0.3333333333333333703, 0.3170188387650512141, 0.3333333333333333703, 0.3170188387650512141, 0.3333333333333333703, 0.3170188387650512141, 0.3333333333333333703, 0.3170188387650512141, 0.3333333333333333703, 0.3170188387650512141, 0.3333333333333333703, 0.3170188387650512141, 0.3333333333333333703, 0.3170188387650512141, 0.3333333333333333703, 0.3170188387650512141, 0.3333333333333333703, 0.3170188387650512141, 0.3333333333333333703, 0.3170188387650512141, 0.3333333333333333703, 0.3170188387650512141, 0.3333333333333333703, 0.3170188387650512141, 0.3333333333333333703, 0.3170188387650512141, 0.3333333333333333703, 0.3170188387650512141, 0.3333333333333333703, 0.3170188387650512141, 0.3333333333333333703, 0.3170188387650512141, 0.3333333333333333703, 0.3170188387650512141, 0.3333333333333333703, 0.3170188387650512141, 0.3333333333333333703, 0.3170188387650512141, 0.3333333333333333703, 0.3170188387650512141, 0.3333333333333333703, 0.3170188387650512141, 0.3333333333333333703, 0.3170188387650512141, 0.3333333333333333703, 0.3170188387650512141, 0.3333333333333333703, 0.3170188387650512141, 0.3333333333333333703, 0.3170188387650512141, 0.3333333333333333703, 0.3170188387650512141, 0.3333333333333333703, 0.3170188387650512141, 0.3333333333333333703, 0.3170188387650512141, 0.3333333333333333703, 0.3170188387650512141, 0.3333333333333333703, 0.3170188387650512141, 0.3333333333333333703, 0.3170188387650512141, 0.3333333333333333703, 0.3170188387650512141, 0.3333333333333333703, 0.3170188387650512141, 0.3333333333333333703, 0.3170188387650512141, 0.3333333333333333703, 0.3170188387650512141, 0.3333333333333333703, 0.3170188387650512141, 0.3333333333333333703, 0.3170188387650512141, 0.3333333333333333703, 0.3170188387650512141, 0.3333333333333333703, 0.3170188387650512141, 0.3333333333333333703, 0.3170188387650512141, 0.3333333333333333703, 0.3170188387650512141, 0.3333333333333333703, 0.3170188387650512141, 0.3333333333333333703, 0.3170188387650512141, 0.3333333333333333703, 0.3170188387650512141, 0.3333333333333333703, 0.3170188387650512141, 0.3333333333333333703, 0.3170188387650512141, 0.3333333333333333703, 0.3170188387650512141, 0.3333333333333333703, 0.3170188387650512141, 0.3333333333333333703, 0.3170188387650512141, 0.3333333333333333703, 0.3170188387650512141, 0.3333333333333333703, 0.3170188387650512141, 0.3333333333333333703, 0.3170188387650512141, 0.3333333333333333703, 0.3170188387650512141, 0.3333333333333333703, 0.3170188387650512141, 0.3333333333333333703, 0.3170188387650512141, 0.3333333333333333703, 0.3170188387650512141, 0.3333333333333333703, 0.3170188387650512141, 0.3333333333333333703, 0.3170188387650512141, 0.3333333333333333703, 0.3170188387650512141, 0.3333333333333333703, 0.3170188387650512141, 0.3333333333333333703, 0.3170188387650512141, 0.3333333333333333703, 0.3170188387650512141, 0.3333333333333333703, 0.3170188387650512141, 0.3333333333333333703, 0.3170188387650512141, 0.3333333333333333703, 0.3170188387650512141, 0.3333333333333333703, 0.3170188387650512141, 0.3333333333333333703, 0.3170188387650512141, 0.3333333333333333703, 0.3170188387650512141, 0.3333333333333333703, 0.3170188387650512141, 0.3333333333333333703, 0.3170188387650512141, 0.3333333333333333703, 0.3170188387650512141, 0.3333333333333333703, 0.3170188387650512141, 0.3333333333333333703, 0.3170188387650512141, 0.3333333333333333703, 0.3170188387650512141, 0.3333333333333333703, 0.3170188387650512141, 0.3333333333333333703, 0.3170188387650512141, 0.3333333333333333703, 0.3170188387650512141, 0.3333333333333333703, 0.3170188387650512141, 0.3333333333333333703, 0.3170188387650512141, 0.3333333333333333703, 0.3170188387650512141, 0.3333333333333333703, 0.3170188387650512141, 0.3333333333333333703, 0.3170188387650512141, 0.3333333333333333703, 0.3170188387650512141, 0.3333333333333333703, 0.3170188387650512141, 0.3333333333333333703, 0.3170188387650512141, 0.3333333333333333703, 0.3170188387650512141, 0.3333333333333333703, 0.3170188387650512141, 0.3333333333333333703, 0.3170188387650512141, 0.3333333333333333703, 0.3170188387650512141, 0.3333333333333333703, 0.3170188387650512141, 0.3333333333333333703, 0.3170188387650512141, 0.3333333333333333703, 0.3170188387650512141, 0.3333333333333333703, 0.3170188387650512141, 0.3333333333333333703, 0.3170188387650512141, 0.3333333333333333703, 0.3170188387650512141, 0.3333333333333333703, 0.3170188387650512141, 0.3333333333333333703, 0.3170188387650512141, 0.3333333333333333703, 0.3170188387650512141, 0.3333333333333333703, 0.3170188387650512141, 0.3333333333333333703, 0.3170188387650512141, 0.3333333333333333703, 0.3170188387650512141, 0.3333333333333333703, 0.3170188387650512141, 0.3333333333333333703, 0.3170188387650512141, 0.3333333333333333703, 0.3170188387650512141, 0.3333333333333333703, 0.3170188387650512141, 0.3333333333333333703, 0.3170188387650512141, 0.3333333333333333703, 0.3170188387650512141, 0.3333333333333333703, 0.3170188387650512141, 0.3333333333333333703, 0.3170188387650512141, 0.3333333333333333703, 0.3170188387650512141, 0.3333333333333333703, 0.3170188387650512141, 0.3333333333333333703, 0.3170188387650512141, 0.3333333333333333703, 0.3170188387650512141, 0.3333333333333333703, 0.3170188387650512141, 0.3333333333333333703, 0.3170188387650512141, 0.3333333333333333703, 0.3170188387650512141, 0.3333333333333333703, 0.3170188387650512141, 0.3333333333333333703, 0.3170188387650512141, 0.3333333333333333703, 0.3170188387650512141, 0.3333333333333333703, 0.3170188387650512141, 0.3333333333333333703, 0.3170188387650512141, 0.3333333333333333703, 0.3170188387650512141, 0.3333333333333333703, 0.3170188387650512141, 0.3333333333333333703, 0.3170188387650512141, 0.3333333333333333703, 0.3170188387650512141, 0.3333333333333333703, 0.3170188387650512141, 0.3333333333333333703, 0.3170188387650512141, 0.3333333333333333703, 0.3170188387650512141, 0.3333333333333333703, 0.3170188387650512141, 0.3333333333333333703, 0.3170188387650512141, 0.3333333333333333703, 0.3170188387650512141, 0.3333333333333333703, 0.3170188387650512141, 0.3333333333333333703, 0.3333333333333333703, 0.3333333333333333703),
 ( 1.000000000000000000, 0.9510565162951535312, 1.000000000000000000, 0.9510565162951535312, 1.000000000000000000, 0.9510565162951535312, 1.000000000000000000, 0.9510565162951535312, 1.000000000000000000, 0.9510565162951535312, 1.000000000000000000, 0.9510565162951535312, 1.000000000000000000, 0.9510565162951535312, 1.000000000000000000, 0.9510565162951535312, 1.000000000000000000, 0.9510565162951535312, 1.000000000000000000, 0.9510565162951535312, 1.000000000000000000, 0.9510565162951535312, 1.000000000000000000, 0.9510565162951535312, 1.000000000000000000, 0.9510565162951535312, 1.000000000000000000, 0.9510565162951535312, 1.000000000000000000, 0.9510565162951535312, 1.000000000000000000, 0.9510565162951535312, 1.000000000000000000, 0.9510565162951535312, 1.000000000000000000, 0.9510565162951535312, 1.000000000000000000, 0.9510565162951535312, 1.000000000000000000, 0.9510565162951535312, 1.000000000000000000, 0.9510565162951535312, 1.000000000000000000, 0.9510565162951535312, 1.000000000000000000, 0.9510565162951535312, 1.000000000000000000, 0.9510565162951535312, 1.000000000000000000, 0.9510565162951535312, 1.000000000000000000, 0.9510565162951535312, 1.000000000000000000, 0.9510565162951535312, 1.000000000000000000, 0.9510565162951535312, 1.000000000000000000, 0.9510565162951535312, 1.000000000000000000, 0.9510565162951535312, 1.000000000000000000, 0.9510565162951535312, 1.000000000000000000, 0.9510565162951535312, 1.000000000000000000, 0.9510565162951535312, 1.000000000000000000, 0.9510565162951535312, 1.000000000000000000, 0.9510565162951535312, 1.000000000000000000, 0.9510565162951535312, 1.000000000000000000, 0.9510565162951535312, 1.000000000000000000, 0.9510565162951535312, 1.000000000000000000, 0.9510565162951535312, 1.000000000000000000, 0.9510565162951535312, 1.000000000000000000, 0.9510565162951535312, 1.000000000000000000, 0.9510565162951535312, 1.000000000000000000, 0.9510565162951535312, 1.000000000000000000, 0.9510565162951535312, 1.000000000000000000, 0.9510565162951535312, 1.000000000000000000, 0.9510565162951535312, 1.000000000000000000, 0.9510565162951535312, 1.000000000000000000, 0.9510565162951535312, 1.000000000000000000, 0.9510565162951535312, 1.000000000000000000, 0.9510565162951535312, 1.000000000000000000, 0.9510565162951535312, 1.000000000000000000, 0.9510565162951535312, 1.000000000000000000, 0.9510565162951535312, 1.000000000000000000, 0.9510565162951535312, 1.000000000000000000, 0.9510565162951535312, 1.000000000000000000, 0.9510565162951535312, 1.000000000000000000, 0.9510565162951535312, 1.000000000000000000, 0.9510565162951535312, 1.000000000000000000, 0.9510565162951535312, 1.000000000000000000, 0.9510565162951535312, 1.000000000000000000, 0.9510565162951535312, 1.000000000000000000, 0.9510565162951535312, 1.000000000000000000, 0.9510565162951535312, 1.000000000000000000, 0.9510565162951535312, 1.000000000000000000, 0.9510565162951535312, 1.000000000000000000, 0.9510565162951535312, 1.000000000000000000, 0.9510565162951535312, 1.000000000000000000, 0.9510565162951535312, 1.000000000000000000, 0.9510565162951535312, 1.000000000000000000, 0.9510565162951535312, 1.000000000000000000, 0.9510565162951535312, 1.000000000000000000, 0.9510565162951535312, 1.000000000000000000, 0.9510565162951535312, 1.000000000000000000, 0.9510565162951535312, 1.000000000000000000, 0.9510565162951535312, 1.000000000000000000, 0.9510565162951535312, 1.000000000000000000, 0.9510565162951535312, 1.000000000000000000, 0.9510565162951535312, 1.000000000000000000, 0.9510565162951535312, 1.000000000000000000, 0.9510565162951535312, 1.000000000000000000, 0.9510565162951535312, 1.000000000000000000, 0.9510565162951535312, 1.000000000000000000, 0.9510565162951535312, 1.000000000000000000, 0.9510565162951535312, 1.000000000000000000, 0.9510565162951535312, 1.000000000000000000, 0.9510565162951535312, 1.000000000000000000, 0.9510565162951535312, 1.000000000000000000, 0.9510565162951535312, 1.000000000000000000, 0.9510565162951535312, 1.000000000000000000, 0.9510565162951535312, 1.000000000000000000, 0.9510565162951535312, 1.000000000000000000, 0.9510565162951535312, 1.000000000000000000, 0.9510565162951535312, 1.000000000000000000, 0.9510565162951535312, 1.000000000000000000, 0.9510565162951535312, 1.000000000000000000, 0.9510565162951535312, 1.000000000000000000, 0.9510565162951535312, 1.000000000000000000, 0.9510565162951535312, 1.000000000000000000, 0.9510565162951535312, 1.000000000000000000, 0.9510565162951535312, 1.000000000000000000, 0.9510565162951535312, 1.000000000000000000, 0.9510565162951535312, 1.000000000000000000, 0.9510565162951535312, 1.000000000000000000, 0.9510565162951535312, 1.000000000000000000, 0.9510565162951535312, 1.000000000000000000, 0.9510565162951535312, 1.000000000000000000, 0.9510565162951535312, 1.000000000000000000, 0.9510565162951535312, 1.000000000000000000, 0.9510565162951535312, 1.000000000000000000, 0.9510565162951535312, 1.000000000000000000, 0.9510565162951535312, 1.000000000000000000, 0.9510565162951535312, 1.000000000000000000, 0.9510565162951535312, 1.000000000000000000, 0.9510565162951535312, 1.000000000000000000, 0.9510565162951535312, 1.000000000000000000, 0.9510565162951535312, 1.000000000000000000, 0.9510565162951535312, 1.000000000000000000, 0.9510565162951535312, 1.000000000000000000, 0.9510565162951535312, 1.000000000000000000, 0.9510565162951535312, 1.000000000000000000, 0.9510565162951535312, 1.000000000000000000, 0.9510565162951535312, 1.000000000000000000, 0.9510565162951535312, 1.000000000000000000, 0.9510565162951535312, 1.000000000000000000, 0.9510565162951535312, 1.000000000000000000, 0.9510565162951535312, 1.000000000000000000, 0.9510565162951535312, 1.000000000000000000, 0.9510565162951535312, 1.000000000000000000, 0.9510565162951535312, 1.000000000000000000, 0.9510565162951535312, 1.000000000000000000, 0.9510565162951535312, 1.000000000000000000, 0.9510565162951535312, 1.000000000000000000, 0.9510565162951535312, 1.000000000000000000, 0.9510565162951535312, 1.000000000000000000, 0.9510565162951535312, 1.000000000000000000, 0.9510565162951535312, 1.000000000000000000, 0.9510565162951535312, 1.000000000000000000, 0.9510565162951535312, 1.000000000000000000, 0.9510565162951535312, 1.000000000000000000, 0.9510565162951535312, 1.000000000000000000, 0.9510565162951535312, 1.000000000000000000, 0.9510565162951535312, 1.000000000000000000, 0.9510565162951535312, 1.000000000000000000, 0.9510565162951535312, 1.000000000000000000, 0.9510565162951535312, 1.000000000000000000, 0.9510565162951535312, 1.000000000000000000, 0.9510565162951535312, 1.000000000000000000, 0.9510565162951535312, 1.000000000000000000, 0.9510565162951535312, 1.000000000000000000, 0.9510565162951535312, 1.000000000000000000, 0.9510565162951535312, 1.000000000000000000, 0.9510565162951535312, 1.000000000000000000, 0.9510565162951535312, 1.000000000000000000, 0.9510565162951535312, 1.000000000000000000, 0.9510565162951535312, 1.000000000000000000, 0.9510565162951535312, 1.000000000000000000, 0.9510565162951535312, 1.000000000000000000, 0.9510565162951535312, 1.000000000000000000, 0.9510565162951535312, 1.000000000000000000, 0.9510565162951535312, 1.000000000000000000, 0.9510565162951535312, 1.000000000000000000, 0.9510565162951535312, 1.000000000000000000, 0.9510565162951535312, 1.000000000000000000, 0.9510565162951535312, 1.000000000000000000, 0.9510565162951535312, 1.000000000000000000, 0.9510565162951535312, 1.000000000000000000, 0.9510565162951535312, 1.000000000000000000, 0.9510565162951535312, 1.000000000000000000, 0.9510565162951535312, 1.000000000000000000, 0.9510565162951535312, 1.000000000000000000, 0.9510565162951535312, 1.000000000000000000, 0.9510565162951535312, 1.000000000000000000, 0.9510565162951535312, 1.000000000000000000, 0.9510565162951535312, 1.000000000000000000, 0.9510565162951535312, 1.000000000000000000, 0.9510565162951535312, 1.000000000000000000, 0.9510565162951535312, 1.000000000000000000, 0.9510565162951535312, 1.000000000000000000, 0.9510565162951535312, 1.000000000000000000, 0.9510565162951535312, 1.000000000000000000, 0.9510565162951535312, 1.000000000000000000, 0.9510565162951535312, 1.000000000000000000, 0.9510565162951535312, 1.000000000000000000, 0.9510565162951535312, 1.000000000000000000, 0.9510565162951535312, 1.000000000000000000, 0.9510565162951535312, 1.000000000000000000, 0.9510565162951535312, 1.000000000000000000, 0.9510565162951535312, 1.000000000000000000, 0.9510565162951535312, 1.000000000000000000, 0.9510565162951535312, 1.000000000000000000, 0.9510565162951535312, 1.000000000000000000, 0.9510565162951535312, 1.000000000000000000, 0.9510565162951535312, 1.000000000000000000, 0.9510565162951535312, 1.000000000000000000, 0.9510565162951535312, 1.000000000000000000, 0.9510565162951535312, 1.000000000000000000, 0.9510565162951535312, 1.000000000000000000, 0.9510565162951535312, 1.000000000000000000, 0.9510565162951535312, 1.000000000000000000, 0.9510565162951535312, 1.000000000000000000, 0.9510565162951535312, 1.000000000000000000, 0.9510565162951535312, 1.000000000000000000, 0.9510565162951535312, 1.000000000000000000, 0.9510565162951535312, 1.000000000000000000, 0.9510565162951535312, 1.000000000000000000, 0.9510565162951535312, 1.000000000000000000, 0.9510565162951535312, 1.000000000000000000, 0.9510565162951535312, 1.000000000000000000, 0.9510565162951535312, 1.000000000000000000, 0.9510565162951535312, 1.000000000000000000, 0.9510565162951535312, 1.000000000000000000, 0.9510565162951535312, 1.000000000000000000, 0.9510565162951535312, 1.000000000000000000, 0.9510565162951535312, 1.000000000000000000, 0.9510565162951535312, 1.000000000000000000, 0.9510565162951535312, 1.000000000000000000, 0.9510565162951535312, 1.000000000000000000, 0.9510565162951535312, 1.000000000000000000, 0.9510565162951535312, 1.000000000000000000, 0.9510565162951535312, 1.000000000000000000, 0.9510565162951535312, 1.000000000000000000, 0.9510565162951535312, 1.000000000000000000, 0.9510565162951535312, 1.000000000000000000, 0.9510565162951535312, 1.000000000000000000, 0.9510565162951535312, 1.000000000000000000, 0.9510565162951535312, 1.000000000000000000, 0.9510565162951535312, 1.000000000000000000, 0.9510565162951535312, 1.000000000000000000, 0.9510565162951535312, 1.000000000000000000, 0.9510565162951535312, 1.000000000000000000, 0.9510565162951535312, 1.000000000000000000, 0.9510565162951535312, 1.000000000000000000, 0.9510565162951535312, 1.000000000000000000, 0.9510565162951535312, 1.000000000000000000, 0.9510565162951535312, 1.000000000000000000, 0.9510565162951535312, 1.000000000000000000, 0.9510565162951535312, 1.000000000000000000, 0.9510565162951535312, 1.000000000000000000, 0.9510565162951535312, 1.000000000000000000, 0.9510565162951535312, 1.000000000000000000, 0.9510565162951535312, 1.000000000000000000, 0.9510565162951535312, 1.000000000000000000, 0.9510565162951535312, 1.000000000000000000, 0.9510565162951535312, 1.000000000000000000, 0.9510565162951535312, 1.000000000000000000, 0.9510565162951535312, 1.000000000000000000, 0.9510565162951535312, 1.000000000000000000, 0.9510565162951535312, 1.000000000000000000, 0.9510565162951535312, 1.000000000000000000, 0.9510565162951535312, 1.000000000000000000, 0.9510565162951535312, 1.000000000000000000, 0.9510565162951535312, 1.000000000000000000, 0.9510565162951535312, 1.000000000000000000, 0.9510565162951535312, 1.000000000000000000, 0.9510565162951535312, 1.000000000000000000, 0.9510565162951535312, 1.000000000000000000, 0.9510565162951535312, 1.000000000000000000, 0.9510565162951535312, 1.000000000000000000, 0.9510565162951535312, 1.000000000000000000, 0.9510565162951535312, 1.000000000000000000, 0.9510565162951535312, 1.000000000000000000, 0.9510565162951535312, 1.000000000000000000, 0.9510565162951535312, 1.000000000000000000, 0.9510565162951535312, 1.000000000000000000, 0.9510565162951535312, 1.000000000000000000, 0.9510565162951535312, 1.000000000000000000, 0.9510565162951535312, 1.000000000000000000, 0.9510565162951535312, 1.000000000000000000, 0.9510565162951535312, 1.000000000000000000, 0.9510565162951535312, 1.000000000000000000, 0.9510565162951535312, 1.000000000000000000, 0.9510565162951535312, 1.000000000000000000, 0.9510565162951535312, 1.000000000000000000, 0.9510565162951535312, 1.000000000000000000, 0.9510565162951535312, 1.000000000000000000, 0.9510565162951535312, 1.000000000000000000, 0.9510565162951535312, 1.000000000000000000, 0.9510565162951535312, 1.000000000000000000, 0.9510565162951535312, 1.000000000000000000, 0.9510565162951535312, 1.000000000000000000, 0.9510565162951535312, 1.000000000000000000, 0.9510565162951535312, 1.000000000000000000, 0.9510565162951535312, 1.000000000000000000, 0.9510565162951535312, 1.000000000000000000, 0.9510565162951535312, 1.000000000000000000, 0.9510565162951535312, 1.000000000000000000, 0.9510565162951535312, 1.000000000000000000, 0.9510565162951535312, 1.000000000000000000, 0.9510565162951535312, 1.000000000000000000, 0.9510565162951535312, 1.000000000000000000, 0.9510565162951535312, 1.000000000000000000, 0.9510565162951535312, 1.000000000000000000, 0.9510565162951535312, 1.000000000000000000, 0.9510565162951535312, 1.000000000000000000, 0.9510565162951535312, 1.000000000000000000, 0.9510565162951535312, 1.000000000000000000, 0.9510565162951535312, 1.000000000000000000, 0.9510565162951535312, 1.000000000000000000, 0.9510565162951535312, 1.000000000000000000, 0.9510565162951535312, 1.000000000000000000, 0.9510565162951535312, 1.000000000000000000, 0.9510565162951535312, 1.000000000000000000, 0.9510565162951535312, 1.000000000000000000, 0.9510565162951535312, 1.000000000000000000, 0.9510565162951535312, 1.000000000000000000, 0.9510565162951535312, 1.000000000000000000, 0.9510565162951535312, 1.000000000000000000, 0.9510565162951535312, 1.000000000000000000, 0.9510565162951535312, 1.000000000000000000, 0.9510565162951535312, 1.000000000000000000, 0.9510565162951535312, 1.000000000000000000, 0.9510565162951535312, 1.000000000000000000, 0.9510565162951535312, 1.000000000000000000, 0.9510565162951535312, 1.000000000000000000, 0.9510565162951535312, 1.000000000000000000, 0.9510565162951535312, 1.000000000000000000, 0.9510565162951535312, 1.000000000000000000, 0.9510565162951535312, 1.000000000000000000, 0.9510565162951535312, 1.000000000000000000, 0.9510565162951535312, 1.000000000000000000, 0.9510565162951535312, 1.000000000000000000, 0.9510565162951535312, 1.000000000000000000, 0.9510565162951535312, 1.000000000000000000, 0.9510565162951535312, 1.000000000000000000, 0.9510565162951535312, 1.000000000000000000, 0.9510565162951535312, 1.000000000000000000, 0.9510565162951535312, 1.000000000000000000, 0.9510565162951535312, 1.000000000000000000, 0.9510565162951535312, 1.000000000000000000, 0.9510565162951535312, 1.000000000000000000, 0.9510565162951535312, 1.000000000000000000, 0.9510565162951535312, 1.000000000000000000, 0.9510565162951535312, 1.000000000000000000, 0.9510565162951535312, 1.000000000000000000, 0.9510565162951535312, 1.000000000000000000, 0.9510565162951535312, 1.000000000000000000, 0.9510565162951535312, 1.000000000000000000, 0.9510565162951535312, 1.000000000000000000, 0.9510565162951535312, 1.000000000000000000, 0.9510565162951535312, 1.000000000000000000, 0.9510565162951535312, 1.000000000000000000, 0.9510565162951535312, 1.000000000000000000, 0.9510565162951535312, 1.000000000000000000, 0.9510565162951535312, 1.000000000000000000, 0.9510565162951535312, 1.000000000000000000, 1.000000000000000000, 1.000000000000000000),
 ( 0.3333333333333333703, 0.3170188387650512141, 0.3333333333333333703, 0.3170188387650512141, 0.3333333333333333703, 0.3170188387650512141, 0.3333333333333333703, 0.3170188387650512141, 0.3333333333333333703, 0.3170188387650512141, 0.3333333333333333703, 0.3170188387650512141, 0.3333333333333333703, 0.3170188387650512141, 0.3333333333333333703, 0.3170188387650512141, 0.3333333333333333703, 0.3170188387650512141, 0.3333333333333333703, 0.3170188387650512141, 0.3333333333333333703, 0.3170188387650512141, 0.3333333333333333703, 0.3170188387650512141, 0.3333333333333333703, 0.3170188387650512141, 0.3333333333333333703, 0.3170188387650512141, 0.3333333333333333703, 0.3170188387650512141, 0.3333333333333333703, 0.3170188387650512141, 0.3333333333333333703, 0.3170188387650512141, 0.3333333333333333703, 0.3170188387650512141, 0.3333333333333333703, 0.3170188387650512141, 0.3333333333333333703, 0.3170188387650512141, 0.3333333333333333703, 0.3170188387650512141, 0.3333333333333333703, 0.3170188387650512141, 0.3333333333333333703, 0.3170188387650512141, 0.3333333333333333703, 0.3170188387650512141, 0.3333333333333333703, 0.3170188387650512141, 0.3333333333333333703, 0.3170188387650512141, 0.3333333333333333703, 0.3170188387650512141, 0.3333333333333333703, 0.3170188387650512141, 0.3333333333333333703, 0.3170188387650512141, 0.3333333333333333703, 0.3170188387650512141, 0.3333333333333333703, 0.3170188387650512141, 0.3333333333333333703, 0.3170188387650512141, 0.3333333333333333703, 0.3170188387650512141, 0.3333333333333333703, 0.3170188387650512141, 0.3333333333333333703, 0.3170188387650512141, 0.3333333333333333703, 0.3170188387650512141, 0.3333333333333333703, 0.3170188387650512141, 0.3333333333333333703, 0.3170188387650512141, 0.3333333333333333703, 0.3170188387650512141, 0.3333333333333333703, 0.3170188387650512141, 0.3333333333333333703, 0.3170188387650512141, 0.3333333333333333703, 0.3170188387650512141, 0.3333333333333333703, 0.3170188387650512141, 0.3333333333333333703, 0.3170188387650512141, 0.3333333333333333703, 0.3170188387650512141, 0.3333333333333333703, 0.3170188387650512141, 0.3333333333333333703, 0.3170188387650512141, 0.3333333333333333703, 0.3170188387650512141, 0.3333333333333333703, 0.3170188387650512141, 0.3333333333333333703, 0.3170188387650512141, 0.3333333333333333703, 0.3170188387650512141, 0.3333333333333333703, 0.3170188387650512141, 0.3333333333333333703, 0.3170188387650512141, 0.3333333333333333703, 0.3170188387650512141, 0.3333333333333333703, 0.3170188387650512141, 0.3333333333333333703, 0.3170188387650512141, 0.3333333333333333703, 0.3170188387650512141, 0.3333333333333333703, 0.3170188387650512141, 0.3333333333333333703, 0.3170188387650512141, 0.3333333333333333703, 0.3170188387650512141, 0.3333333333333333703, 0.3170188387650512141, 0.3333333333333333703, 0.3170188387650512141, 0.3333333333333333703, 0.3170188387650512141, 0.3333333333333333703, 0.3170188387650512141, 0.3333333333333333703, 0.3170188387650512141, 0.3333333333333333703, 0.3170188387650512141, 0.3333333333333333703, 0.3170188387650512141, 0.3333333333333333703, 0.3170188387650512141, 0.3333333333333333703, 0.3170188387650512141, 0.3333333333333333703, 0.3170188387650512141, 0.3333333333333333703, 0.3170188387650512141, 0.3333333333333333703, 0.3170188387650512141, 0.3333333333333333703, 0.3170188387650512141, 0.3333333333333333703, 0.3170188387650512141, 0.3333333333333333703, 0.3170188387650512141, 0.3333333333333333703, 0.3170188387650512141, 0.3333333333333333703, 0.3170188387650512141, 0.3333333333333333703, 0.3170188387650512141, 0.3333333333333333703, 0.3170188387650512141, 0.3333333333333333703, 0.3170188387650512141, 0.3333333333333333703, 0.3170188387650512141, 0.3333333333333333703, 0.3170188387650512141, 0.3333333333333333703, 0.3170188387650512141, 0.3333333333333333703, 0.3170188387650512141, 0.3333333333333333703, 0.3170188387650512141, 0.3333333333333333703, 0.3170188387650512141, 0.3333333333333333703, 0.3170188387650512141, 0.3333333333333333703, 0.3170188387650512141, 0.3333333333333333703, 0.3170188387650512141, 0.3333333333333333703, 0.3170188387650512141, 0.3333333333333333703, 0.3170188387650512141, 0.3333333333333333703, 0.3170188387650512141, 0.3333333333333333703, 0.3170188387650512141, 0.3333333333333333703, 0.3170188387650512141, 0.3333333333333333703, 0.3170188387650512141, 0.3333333333333333703, 0.3170188387650512141, 0.3333333333333333703, 0.3170188387650512141, 0.3333333333333333703, 0.3170188387650512141, 0.3333333333333333703, 0.3170188387650512141, 0.3333333333333333703, 0.3170188387650512141, 0.3333333333333333703, 0.3170188387650512141, 0.3333333333333333703, 0.3170188387650512141, 0.3333333333333333703, 0.3170188387650512141, 0.3333333333333333703, 0.3170188387650512141, 0.3333333333333333703, 0.3170188387650512141, 0.3333333333333333703, 0.3170188387650512141, 0.3333333333333333703, 0.3170188387650512141, 0.3333333333333333703, 0.3170188387650512141, 0.3333333333333333703, 0.3170188387650512141, 0.3333333333333333703, 0.3170188387650512141, 0.3333333333333333703, 0.3170188387650512141, 0.3333333333333333703, 0.3170188387650512141, 0.3333333333333333703, 0.3170188387650512141, 0.3333333333333333703, 0.3170188387650512141, 0.3333333333333333703, 0.3170188387650512141, 0.3333333333333333703, 0.3170188387650512141, 0.3333333333333333703, 0.3170188387650512141, 0.3333333333333333703, 0.3170188387650512141, 0.3333333333333333703, 0.3170188387650512141, 0.3333333333333333703, 0.3170188387650512141, 0.3333333333333333703, 0.3170188387650512141, 0.3333333333333333703, 0.3170188387650512141, 0.3333333333333333703, 0.3170188387650512141, 0.3333333333333333703, 0.3170188387650512141, 0.3333333333333333703, 0.3170188387650512141, 0.3333333333333333703, 0.3170188387650512141, 0.3333333333333333703, 0.3170188387650512141, 0.3333333333333333703, 0.3170188387650512141, 0.3333333333333333703, 0.3170188387650512141, 0.3333333333333333703, 0.3170188387650512141, 0.3333333333333333703, 0.3170188387650512141, 0.3333333333333333703, 0.3170188387650512141, 0.3333333333333333703, 0.3170188387650512141, 0.3333333333333333703, 0.3170188387650512141, 0.3333333333333333703, 0.3170188387650512141, 0.3333333333333333703, 0.3170188387650512141, 0.3333333333333333703, 0.3170188387650512141, 0.3333333333333333703, 0.3170188387650512141, 0.3333333333333333703, 0.3170188387650512141, 0.3333333333333333703, 0.3170188387650512141, 0.3333333333333333703, 0.3170188387650512141, 0.3333333333333333703, 0.3170188387650512141, 0.3333333333333333703, 0.3170188387650512141, 0.3333333333333333703, 0.3170188387650512141, 0.3333333333333333703, 0.3170188387650512141, 0.3333333333333333703, 0.3170188387650512141, 0.3333333333333333703, 0.3170188387650512141, 0.3333333333333333703, 0.3170188387650512141, 0.3333333333333333703, 0.3170188387650512141, 0.3333333333333333703, 0.3170188387650512141, 0.3333333333333333703, 0.3170188387650512141, 0.3333333333333333703, 0.3170188387650512141, 0.3333333333333333703, 0.3170188387650512141, 0.3333333333333333703, 0.3170188387650512141, 0.3333333333333333703, 0.3170188387650512141, 0.3333333333333333703, 0.3170188387650512141, 0.3333333333333333703, 0.3170188387650512141, 0.3333333333333333703, 0.3170188387650512141, 0.3333333333333333703, 0.3170188387650512141, 0.3333333333333333703, 0.3170188387650512141, 0.3333333333333333703, 0.3170188387650512141, 0.3333333333333333703, 0.3170188387650512141, 0.3333333333333333703, 0.3170188387650512141, 0.3333333333333333703, 0.3170188387650512141, 0.3333333333333333703, 0.3170188387650512141, 0.3333333333333333703, 0.3170188387650512141, 0.3333333333333333703, 0.3170188387650512141, 0.3333333333333333703, 0.3170188387650512141, 0.3333333333333333703, 0.3170188387650512141, 0.3333333333333333703, 0.3170188387650512141, 0.3333333333333333703, 0.3170188387650512141, 0.3333333333333333703, 0.3170188387650512141, 0.3333333333333333703, 0.3170188387650512141, 0.3333333333333333703, 0.3170188387650512141, 0.3333333333333333703, 0.3170188387650512141, 0.3333333333333333703, 0.3170188387650512141, 0.3333333333333333703, 0.3170188387650512141, 0.3333333333333333703, 0.3170188387650512141, 0.3333333333333333703, 0.3170188387650512141, 0.3333333333333333703, 0.3170188387650512141, 0.3333333333333333703, 0.3170188387650512141, 0.3333333333333333703, 0.3170188387650512141, 0.3333333333333333703, 0.3170188387650512141, 0.3333333333333333703, 0.3170188387650512141, 0.3333333333333333703, 0.3170188387650512141, 0.3333333333333333703, 0.3170188387650512141, 0.3333333333333333703, 0.3170188387650512141, 0.3333333333333333703, 0.3170188387650512141, 0.3333333333333333703, 0.3170188387650512141, 0.3333333333333333703, 0.3170188387650512141, 0.3333333333333333703, 0.3170188387650512141, 0.3333333333333333703, 0.3170188387650512141, 0.3333333333333333703, 0.3170188387650512141, 0.3333333333333333703, 0.3170188387650512141, 0.3333333333333333703, 0.3170188387650512141, 0.3333333333333333703, 0.3170188387650512141, 0.3333333333333333703, 0.3170188387650512141, 0.3333333333333333703, 0.3170188387650512141, 0.3333333333333333703, 0.3170188387650512141, 0.3333333333333333703, 0.3170188387650512141, 0.3333333333333333703, 0.3170188387650512141, 0.3333333333333333703, 0.3170188387650512141, 0.3333333333333333703, 0.3170188387650512141, 0.3333333333333333703, 0.3170188387650512141, 0.3333333333333333703, 0.3170188387650512141, 0.3333333333333333703, 0.3170188387650512141, 0.3333333333333333703, 0.3170188387650512141, 0.3333333333333333703, 0.3170188387650512141, 0.3333333333333333703, 0.3170188387650512141, 0.3333333333333333703, 0.3170188387650512141, 0.3333333333333333703, 0.3170188387650512141, 0.3333333333333333703, 0.3170188387650512141, 0.3333333333333333703, 0.3170188387650512141, 0.3333333333333333703, 0.3170188387650512141, 0.3333333333333333703, 0.3170188387650512141, 0.3333333333333333703, 0.3170188387650512141, 0.3333333333333333703, 0.3170188387650512141, 0.3333333333333333703, 0.3170188387650512141, 0.3333333333333333703, 0.3170188387650512141, 0.3333333333333333703, 0.3170188387650512141, 0.3333333333333333703, 0.3170188387650512141, 0.3333333333333333703, 0.3170188387650512141, 0.3333333333333333703, 0.3170188387650512141, 0.3333333333333333703, 0.3170188387650512141, 0.3333333333333333703, 0.3170188387650512141, 0.3333333333333333703, 0.3170188387650512141, 0.3333333333333333703, 0.3170188387650512141, 0.3333333333333333703, 0.3170188387650512141, 0.3333333333333333703, 0.3170188387650512141, 0.3333333333333333703, 0.3170188387650512141, 0.3333333333333333703, 0.3170188387650512141, 0.3333333333333333703, 0.3170188387650512141, 0.3333333333333333703, 0.3170188387650512141, 0.3333333333333333703, 0.3170188387650512141, 0.3333333333333333703, 0.3170188387650512141, 0.3333333333333333703, 0.3170188387650512141, 0.3333333333333333703, 0.3170188387650512141, 0.3333333333333333703, 0.3170188387650512141, 0.3333333333333333703, 0.3170188387650512141, 0.3333333333333333703, 0.3170188387650512141, 0.3333333333333333703, 0.3170188387650512141, 0.3333333333333333703, 0.3170188387650512141, 0.3333333333333333703, 0.3170188387650512141, 0.3333333333333333703, 0.3170188387650512141, 0.3333333333333333703, 0.3170188387650512141, 0.3333333333333333703, 0.3170188387650512141, 0.3333333333333333703, 0.3170188387650512141, 0.3333333333333333703, 0.3170188387650512141, 0.3333333333333333703, 0.3170188387650512141, 0.3333333333333333703, 0.3170188387650512141, 0.3333333333333333703, 0.3170188387650512141, 0.3333333333333333703, 0.3170188387650512141, 0.3333333333333333703, 0.3170188387650512141, 0.3333333333333333703, 0.3170188387650512141, 0.3333333333333333703, 0.3170188387650512141, 0.3333333333333333703, 0.3170188387650512141, 0.3333333333333333703, 0.3170188387650512141, 0.3333333333333333703, 0.3170188387650512141, 0.3333333333333333703, 0.3170188387650512141, 0.3333333333333333703, 0.3170188387650512141, 0.3333333333333333703, 0.3170188387650512141, 0.3333333333333333703, 0.3170188387650512141, 0.3333333333333333703, 0.3170188387650512141, 0.3333333333333333703, 0.3170188387650512141, 0.3333333333333333703, 0.3170188387650512141, 0.3333333333333333703, 0.3170188387650512141, 0.3333333333333333703, 0.3170188387650512141, 0.3333333333333333703, 0.3170188387650512141, 0.3333333333333333703, 0.3170188387650512141, 0.3333333333333333703, 0.3170188387650512141, 0.3333333333333333703, 0.3170188387650512141, 0.3333333333333333703, 0.3170188387650512141, 0.3333333333333333703, 0.3170188387650512141, 0.3333333333333333703, 0.3170188387650512141, 0.3333333333333333703, 0.3170188387650512141, 0.3333333333333333703, 0.3170188387650512141, 0.3333333333333333703, 0.3170188387650512141, 0.3333333333333333703, 0.3170188387650512141, 0.3333333333333333703, 0.3170188387650512141, 0.3333333333333333703, 0.3170188387650512141, 0.3333333333333333703, 0.3170188387650512141, 0.3333333333333333703, 0.3170188387650512141, 0.3333333333333333703, 0.3170188387650512141, 0.3333333333333333703, 0.3170188387650512141, 0.3333333333333333703, 0.3170188387650512141, 0.3333333333333333703, 0.3170188387650512141, 0.3333333333333333703, 0.3170188387650512141, 0.3333333333333333703, 0.3170188387650512141, 0.3333333333333333703, 0.3170188387650512141, 0.3333333333333333703, 0.3170188387650512141, 0.3333333333333333703, 0.3170188387650512141, 0.3333333333333333703, 0.3170188387650512141, 0.3333333333333333703, 0.3170188387650512141, 0.3333333333333333703, 0.3170188387650512141, 0.3333333333333333703, 0.3170188387650512141, 0.3333333333333333703, 0.3170188387650512141, 0.3333333333333333703, 0.3170188387650512141, 0.3333333333333333703, 0.3170188387650512141, 0.3333333333333333703, 0.3170188387650512141, 0.3333333333333333703, 0.3170188387650512141, 0.3333333333333333703, 0.3170188387650512141, 0.3333333333333333703, 0.3170188387650512141, 0.3333333333333333703, 0.3170188387650512141, 0.3333333333333333703, 0.3170188387650512141, 0.3333333333333333703, 0.3170188387650512141, 0.3333333333333333703, 0.3170188387650512141, 0.3333333333333333703, 0.3170188387650512141, 0.3333333333333333703, 0.3170188387650512141, 0.3333333333333333703, 0.3170188387650512141, 0.3333333333333333703, 0.3170188387650512141, 0.3333333333333333703, 0.3170188387650512141, 0.3333333333333333703, 0.3170188387650512141, 0.3333333333333333703, 0.3170188387650512141, 0.3333333333333333703, 0.3170188387650512141, 0.3333333333333333703, 0.3170188387650512141, 0.3333333333333333703, 0.3170188387650512141, 0.3333333333333333703, 0.3170188387650512141, 0.3333333333333333703, 0.3170188387650512141, 0.3333333333333333703, 0.3170188387650512141, 0.3333333333333333703, 0.3170188387650512141, 0.3333333333333333703, 0.3170188387650512141, 0.3333333333333333703, 0.3170188387650512141, 0.3333333333333333703, 0.3170188387650512141, 0.3333333333333333703, 0.3170188387650512141, 0.3333333333333333703, 0.3170188387650512141, 0.3333333333333333703, 0.3170188387650512141, 0.3333333333333333703, 0.3170188387650512141, 0.3333333333333333703, 0.3170188387650512141, 0.3333333333333333703, 0.3170188387650512141, 0.3333333333333333703, 0.3170188387650512141, 0.3333333333333333703, 0.3170188387650512141, 0.3333333333333333703, 0.3170188387650512141, 0.3333333333333333703, 0.3170188387650512141, 0.3333333333333333703, 0.3170188387650512141, 0.3333333333333333703, 0.3170188387650512141, 0.3333333333333333703, 0.3170188387650512141, 0.3333333333333333703, 0.3170188387650512141, 0.3333333333333333703, 0.3170188387650512141, 0.3333333333333333703, 0.3170188387650512141, 0.3333333333333333703, 0.3170188387650512141, 0.3333333333333333703, 0.3170188387650512141, 0.3333333333333333703, 0.3170188387650512141, 0.3333333333333333703, 0.3170188387650512141, 0.3333333333333333703, 0.3170188387650512141, 0.3333333333333333703, 0.3170188387650512141, 0.3333333333333333703, 0.3333333333333333703, 0.3333333333333333703),
 ( 0.3333333333333333703, 0.3170188387650512141, 0.3333333333333333703, 0.3170188387650512141, 0.3333333333333333703, 0.3170188387650512141, 0.3333333333333333703, 0.3170188387650512141, 0.3333333333333333703, 0.3170188387650512141, 0.3333333333333333703, 0.3170188387650512141, 0.3333333333333333703, 0.3170188387650512141, 0.3333333333333333703, 0.3170188387650512141, 0.3333333333333333703, 0.3170188387650512141, 0.3333333333333333703, 0.3170188387650512141, 0.3333333333333333703, 0.3170188387650512141, 0.3333333333333333703, 0.3170188387650512141, 0.3333333333333333703, 0.3170188387650512141, 0.3333333333333333703, 0.3170188387650512141, 0.3333333333333333703, 0.3170188387650512141, 0.3333333333333333703, 0.3170188387650512141, 0.3333333333333333703, 0.3170188387650512141, 0.3333333333333333703, 0.3170188387650512141, 0.3333333333333333703, 0.3170188387650512141, 0.3333333333333333703, 0.3170188387650512141, 0.3333333333333333703, 0.3170188387650512141, 0.3333333333333333703, 0.3170188387650512141, 0.3333333333333333703, 0.3170188387650512141, 0.3333333333333333703, 0.3170188387650512141, 0.3333333333333333703, 0.3170188387650512141, 0.3333333333333333703, 0.3170188387650512141, 0.3333333333333333703, 0.3170188387650512141, 0.3333333333333333703, 0.3170188387650512141, 0.3333333333333333703, 0.3170188387650512141, 0.3333333333333333703, 0.3170188387650512141, 0.3333333333333333703, 0.3170188387650512141, 0.3333333333333333703, 0.3170188387650512141, 0.3333333333333333703, 0.3170188387650512141, 0.3333333333333333703, 0.3170188387650512141, 0.3333333333333333703, 0.3170188387650512141, 0.3333333333333333703, 0.3170188387650512141, 0.3333333333333333703, 0.3170188387650512141, 0.3333333333333333703, 0.3170188387650512141, 0.3333333333333333703, 0.3170188387650512141, 0.3333333333333333703, 0.3170188387650512141, 0.3333333333333333703, 0.3170188387650512141, 0.3333333333333333703, 0.3170188387650512141, 0.3333333333333333703, 0.3170188387650512141, 0.3333333333333333703, 0.3170188387650512141, 0.3333333333333333703, 0.3170188387650512141, 0.3333333333333333703, 0.3170188387650512141, 0.3333333333333333703, 0.3170188387650512141, 0.3333333333333333703, 0.3170188387650512141, 0.3333333333333333703, 0.3170188387650512141, 0.3333333333333333703, 0.3170188387650512141, 0.3333333333333333703, 0.3170188387650512141, 0.3333333333333333703, 0.3170188387650512141, 0.3333333333333333703, 0.3170188387650512141, 0.3333333333333333703, 0.3170188387650512141, 0.3333333333333333703, 0.3170188387650512141, 0.3333333333333333703, 0.3170188387650512141, 0.3333333333333333703, 0.3170188387650512141, 0.3333333333333333703, 0.3170188387650512141, 0.3333333333333333703, 0.3170188387650512141, 0.3333333333333333703, 0.3170188387650512141, 0.3333333333333333703, 0.3170188387650512141, 0.3333333333333333703, 0.3170188387650512141, 0.3333333333333333703, 0.3170188387650512141, 0.3333333333333333703, 0.3170188387650512141, 0.3333333333333333703, 0.3170188387650512141, 0.3333333333333333703, 0.3170188387650512141, 0.3333333333333333703, 0.3170188387650512141, 0.3333333333333333703, 0.3170188387650512141, 0.3333333333333333703, 0.3170188387650512141, 0.3333333333333333703, 0.3170188387650512141, 0.3333333333333333703, 0.3170188387650512141, 0.3333333333333333703, 0.3170188387650512141, 0.3333333333333333703, 0.3170188387650512141, 0.3333333333333333703, 0.3170188387650512141, 0.3333333333333333703, 0.3170188387650512141, 0.3333333333333333703, 0.3170188387650512141, 0.3333333333333333703, 0.3170188387650512141, 0.3333333333333333703, 0.3170188387650512141, 0.3333333333333333703, 0.3170188387650512141, 0.3333333333333333703, 0.3170188387650512141, 0.3333333333333333703, 0.3170188387650512141, 0.3333333333333333703, 0.3170188387650512141, 0.3333333333333333703, 0.3170188387650512141, 0.3333333333333333703, 0.3170188387650512141, 0.3333333333333333703, 0.3170188387650512141, 0.3333333333333333703, 0.3170188387650512141, 0.3333333333333333703, 0.3170188387650512141, 0.3333333333333333703, 0.3170188387650512141, 0.3333333333333333703, 0.3170188387650512141, 0.3333333333333333703, 0.3170188387650512141, 0.3333333333333333703, 0.3170188387650512141, 0.3333333333333333703, 0.3170188387650512141, 0.3333333333333333703, 0.3170188387650512141, 0.3333333333333333703, 0.3170188387650512141, 0.3333333333333333703, 0.3170188387650512141, 0.3333333333333333703, 0.3170188387650512141, 0.3333333333333333703, 0.3170188387650512141, 0.3333333333333333703, 0.3170188387650512141, 0.3333333333333333703, 0.3170188387650512141, 0.3333333333333333703, 0.3170188387650512141, 0.3333333333333333703, 0.3170188387650512141, 0.3333333333333333703, 0.3170188387650512141, 0.3333333333333333703, 0.3170188387650512141, 0.3333333333333333703, 0.3170188387650512141, 0.3333333333333333703, 0.3170188387650512141, 0.3333333333333333703, 0.3170188387650512141, 0.3333333333333333703, 0.3170188387650512141, 0.3333333333333333703, 0.3170188387650512141, 0.3333333333333333703, 0.3170188387650512141, 0.3333333333333333703, 0.3170188387650512141, 0.3333333333333333703, 0.3170188387650512141, 0.3333333333333333703, 0.3170188387650512141, 0.3333333333333333703, 0.3170188387650512141, 0.3333333333333333703, 0.3170188387650512141, 0.3333333333333333703, 0.3170188387650512141, 0.3333333333333333703, 0.3170188387650512141, 0.3333333333333333703, 0.3170188387650512141, 0.3333333333333333703, 0.3170188387650512141, 0.3333333333333333703, 0.3170188387650512141, 0.3333333333333333703, 0.3170188387650512141, 0.3333333333333333703, 0.3170188387650512141, 0.3333333333333333703, 0.3170188387650512141, 0.3333333333333333703, 0.3170188387650512141, 0.3333333333333333703, 0.3170188387650512141, 0.3333333333333333703, 0.3170188387650512141, 0.3333333333333333703, 0.3170188387650512141, 0.3333333333333333703, 0.3170188387650512141, 0.3333333333333333703, 0.3170188387650512141, 0.3333333333333333703, 0.3170188387650512141, 0.3333333333333333703, 0.3170188387650512141, 0.3333333333333333703, 0.3170188387650512141, 0.3333333333333333703, 0.3170188387650512141, 0.3333333333333333703, 0.3170188387650512141, 0.3333333333333333703, 0.3170188387650512141, 0.3333333333333333703, 0.3170188387650512141, 0.3333333333333333703, 0.3170188387650512141, 0.3333333333333333703, 0.3170188387650512141, 0.3333333333333333703, 0.3170188387650512141, 0.3333333333333333703, 0.3170188387650512141, 0.3333333333333333703, 0.3170188387650512141, 0.3333333333333333703, 0.3170188387650512141, 0.3333333333333333703, 0.3170188387650512141, 0.3333333333333333703, 0.3170188387650512141, 0.3333333333333333703, 0.3170188387650512141, 0.3333333333333333703, 0.3170188387650512141, 0.3333333333333333703, 0.3170188387650512141, 0.3333333333333333703, 0.3170188387650512141, 0.3333333333333333703, 0.3170188387650512141, 0.3333333333333333703, 0.3170188387650512141, 0.3333333333333333703, 0.3170188387650512141, 0.3333333333333333703, 0.3170188387650512141, 0.3333333333333333703, 0.3170188387650512141, 0.3333333333333333703, 0.3170188387650512141, 0.3333333333333333703, 0.3170188387650512141, 0.3333333333333333703, 0.3170188387650512141, 0.3333333333333333703, 0.3170188387650512141, 0.3333333333333333703, 0.3170188387650512141, 0.3333333333333333703, 0.3170188387650512141, 0.3333333333333333703, 0.3170188387650512141, 0.3333333333333333703, 0.3170188387650512141, 0.3333333333333333703, 0.3170188387650512141, 0.3333333333333333703, 0.3170188387650512141, 0.3333333333333333703, 0.3170188387650512141, 0.3333333333333333703, 0.3170188387650512141, 0.3333333333333333703, 0.3170188387650512141, 0.3333333333333333703, 0.3170188387650512141, 0.3333333333333333703, 0.3170188387650512141, 0.3333333333333333703, 0.3170188387650512141, 0.3333333333333333703, 0.3170188387650512141, 0.3333333333333333703, 0.3170188387650512141, 0.3333333333333333703, 0.3170188387650512141, 0.3333333333333333703, 0.3170188387650512141, 0.3333333333333333703, 0.3170188387650512141, 0.3333333333333333703, 0.3170188387650512141, 0.3333333333333333703, 0.3170188387650512141, 0.3333333333333333703, 0.3170188387650512141, 0.3333333333333333703, 0.3170188387650512141, 0.3333333333333333703, 0.3170188387650512141, 0.3333333333333333703, 0.3170188387650512141, 0.3333333333333333703, 0.3170188387650512141, 0.3333333333333333703, 0.3170188387650512141, 0.3333333333333333703, 0.3170188387650512141, 0.3333333333333333703, 0.3170188387650512141, 0.3333333333333333703, 0.3170188387650512141, 0.3333333333333333703, 0.3170188387650512141, 0.3333333333333333703, 0.3170188387650512141, 0.3333333333333333703, 0.3170188387650512141, 0.3333333333333333703, 0.3170188387650512141, 0.3333333333333333703, 0.3170188387650512141, 0.3333333333333333703, 0.3170188387650512141, 0.3333333333333333703, 0.3170188387650512141, 0.3333333333333333703, 0.3170188387650512141, 0.3333333333333333703, 0.3170188387650512141, 0.3333333333333333703, 0.3170188387650512141, 0.3333333333333333703, 0.3170188387650512141, 0.3333333333333333703, 0.3170188387650512141, 0.3333333333333333703, 0.3170188387650512141, 0.3333333333333333703, 0.3170188387650512141, 0.3333333333333333703, 0.3170188387650512141, 0.3333333333333333703, 0.3170188387650512141, 0.3333333333333333703, 0.3170188387650512141, 0.3333333333333333703, 0.3170188387650512141, 0.3333333333333333703, 0.3170188387650512141, 0.3333333333333333703, 0.3170188387650512141, 0.3333333333333333703, 0.3170188387650512141, 0.3333333333333333703, 0.3170188387650512141, 0.3333333333333333703, 0.3170188387650512141, 0.3333333333333333703, 0.3170188387650512141, 0.3333333333333333703, 0.3170188387650512141, 0.3333333333333333703, 0.3170188387650512141, 0.3333333333333333703, 0.3170188387650512141, 0.3333333333333333703, 0.3170188387650512141, 0.3333333333333333703, 0.3170188387650512141, 0.3333333333333333703, 0.3170188387650512141, 0.3333333333333333703, 0.3170188387650512141, 0.3333333333333333703, 0.3170188387650512141, 0.3333333333333333703, 0.3170188387650512141, 0.3333333333333333703, 0.3170188387650512141, 0.3333333333333333703, 0.3170188387650512141, 0.3333333333333333703, 0.3170188387650512141, 0.3333333333333333703, 0.3170188387650512141, 0.3333333333333333703, 0.3170188387650512141, 0.3333333333333333703, 0.3170188387650512141, 0.3333333333333333703, 0.3170188387650512141, 0.3333333333333333703, 0.3170188387650512141, 0.3333333333333333703, 0.3170188387650512141, 0.3333333333333333703, 0.3170188387650512141, 0.3333333333333333703, 0.3170188387650512141, 0.3333333333333333703, 0.3170188387650512141, 0.3333333333333333703, 0.3170188387650512141, 0.3333333333333333703, 0.3170188387650512141, 0.3333333333333333703, 0.3170188387650512141, 0.3333333333333333703, 0.3170188387650512141, 0.3333333333333333703, 0.3170188387650512141, 0.3333333333333333703, 0.3170188387650512141, 0.3333333333333333703, 0.3170188387650512141, 0.3333333333333333703, 0.3170188387650512141, 0.3333333333333333703, 0.3170188387650512141, 0.3333333333333333703, 0.3170188387650512141, 0.3333333333333333703, 0.3170188387650512141, 0.3333333333333333703, 0.3170188387650512141, 0.3333333333333333703, 0.3170188387650512141, 0.3333333333333333703, 0.3170188387650512141, 0.3333333333333333703, 0.3170188387650512141, 0.3333333333333333703, 0.3170188387650512141, 0.3333333333333333703, 0.3170188387650512141, 0.3333333333333333703, 0.3170188387650512141, 0.3333333333333333703, 0.3170188387650512141, 0.3333333333333333703, 0.3170188387650512141, 0.3333333333333333703, 0.3170188387650512141, 0.3333333333333333703, 0.3170188387650512141, 0.3333333333333333703, 0.3170188387650512141, 0.3333333333333333703, 0.3170188387650512141, 0.3333333333333333703, 0.3170188387650512141, 0.3333333333333333703, 0.3170188387650512141, 0.3333333333333333703, 0.3170188387650512141, 0.3333333333333333703, 0.3170188387650512141, 0.3333333333333333703, 0.3170188387650512141, 0.3333333333333333703, 0.3170188387650512141, 0.3333333333333333703, 0.3170188387650512141, 0.3333333333333333703, 0.3170188387650512141, 0.3333333333333333703, 0.3170188387650512141, 0.3333333333333333703, 0.3170188387650512141, 0.3333333333333333703, 0.3170188387650512141, 0.3333333333333333703, 0.3170188387650512141, 0.3333333333333333703, 0.3170188387650512141, 0.3333333333333333703, 0.3170188387650512141, 0.3333333333333333703, 0.3170188387650512141, 0.3333333333333333703, 0.3170188387650512141, 0.3333333333333333703, 0.3170188387650512141, 0.3333333333333333703, 0.3170188387650512141, 0.3333333333333333703, 0.3170188387650512141, 0.3333333333333333703, 0.3170188387650512141, 0.3333333333333333703, 0.3170188387650512141, 0.3333333333333333703, 0.3170188387650512141, 0.3333333333333333703, 0.3170188387650512141, 0.3333333333333333703, 0.3170188387650512141, 0.3333333333333333703, 0.3170188387650512141, 0.3333333333333333703, 0.3170188387650512141, 0.3333333333333333703, 0.3170188387650512141, 0.3333333333333333703, 0.3170188387650512141, 0.3333333333333333703, 0.3170188387650512141, 0.3333333333333333703, 0.3170188387650512141, 0.3333333333333333703, 0.3170188387650512141, 0.3333333333333333703, 0.3170188387650512141, 0.3333333333333333703, 0.3170188387650512141, 0.3333333333333333703, 0.3170188387650512141, 0.3333333333333333703, 0.3170188387650512141, 0.3333333333333333703, 0.3170188387650512141, 0.3333333333333333703, 0.3170188387650512141, 0.3333333333333333703, 0.3170188387650512141, 0.3333333333333333703, 0.3170188387650512141, 0.3333333333333333703, 0.3170188387650512141, 0.3333333333333333703, 0.3170188387650512141, 0.3333333333333333703, 0.3170188387650512141, 0.3333333333333333703, 0.3170188387650512141, 0.3333333333333333703, 0.3170188387650512141, 0.3333333333333333703, 0.3170188387650512141, 0.3333333333333333703, 0.3170188387650512141, 0.3333333333333333703, 0.3170188387650512141, 0.3333333333333333703, 0.3170188387650512141, 0.3333333333333333703, 0.3170188387650512141, 0.3333333333333333703, 0.3170188387650512141, 0.3333333333333333703, 0.3170188387650512141, 0.3333333333333333703, 0.3170188387650512141, 0.3333333333333333703, 0.3170188387650512141, 0.3333333333333333703, 0.3170188387650512141, 0.3333333333333333703, 0.3170188387650512141, 0.3333333333333333703, 0.3170188387650512141, 0.3333333333333333703, 0.3170188387650512141, 0.3333333333333333703, 0.3170188387650512141, 0.3333333333333333703, 0.3170188387650512141, 0.3333333333333333703, 0.3170188387650512141, 0.3333333333333333703, 0.3170188387650512141, 0.3333333333333333703, 0.3170188387650512141, 0.3333333333333333703, 0.3170188387650512141, 0.3333333333333333703, 0.3170188387650512141, 0.3333333333333333703, 0.3170188387650512141, 0.3333333333333333703, 0.3170188387650512141, 0.3333333333333333703, 0.3170188387650512141, 0.3333333333333333703, 0.3170188387650512141, 0.3333333333333333703, 0.3170188387650512141, 0.3333333333333333703, 0.3170188387650512141, 0.3333333333333333703, 0.3170188387650512141, 0.3333333333333333703, 0.3170188387650512141, 0.3333333333333333703, 0.3170188387650512141, 0.3333333333333333703, 0.3170188387650512141, 0.3333333333333333703, 0.3170188387650512141, 0.3333333333333333703, 0.3170188387650512141, 0.3333333333333333703, 0.3170188387650512141, 0.3333333333333333703, 0.3170188387650512141, 0.3333333333333333703, 0.3170188387650512141, 0.3333333333333333703, 0.3170188387650512141, 0.3333333333333333703, 0.3170188387650512141, 0.3333333333333333703, 0.3170188387650512141, 0.3333333333333333703, 0.3170188387650512141, 0.3333333333333333703, 0.3170188387650512141, 0.3333333333333333703, 0.3170188387650512141, 0.3333333333333333703, 0.3170188387650512141, 0.3333333333333333703, 0.3170188387650512141, 0.3333333333333333703, 0.3170188387650512141, 0.3333333333333333703, 0.3170188387650512141, 0.3333333333333333703, 0.3170188387650512141, 0.3333333333333333703, 0.3170188387650512141, 0.3333333333333333703, 0.3170188387650512141, 0.3333333333333333703, 0.3333333333333333703, 0.3333333333333333703),
 ( 1.000000000000000000, 0.9510565162951535312, 1.000000000000000000, 0.9510565162951535312, 1.000000000000000000, 0.9510565162951535312, 1.000000000000000000, 0.9510565162951535312, 1.000000000000000000, 0.9510565162951535312, 1.000000000000000000, 0.9510565162951535312, 1.000000000000000000, 0.9510565162951535312, 1.000000000000000000, 0.9510565162951535312, 1.000000000000000000, 0.9510565162951535312, 1.000000000000000000, 0.9510565162951535312, 1.000000000000000000, 0.9510565162951535312, 1.000000000000000000, 0.9510565162951535312, 1.000000000000000000, 0.9510565162951535312, 1.000000000000000000, 0.9510565162951535312, 1.000000000000000000, 0.9510565162951535312, 1.000000000000000000, 0.9510565162951535312, 1.000000000000000000, 0.9510565162951535312, 1.000000000000000000, 0.9510565162951535312, 1.000000000000000000, 0.9510565162951535312, 1.000000000000000000, 0.9510565162951535312, 1.000000000000000000, 0.9510565162951535312, 1.000000000000000000, 0.9510565162951535312, 1.000000000000000000, 0.9510565162951535312, 1.000000000000000000, 0.9510565162951535312, 1.000000000000000000, 0.9510565162951535312, 1.000000000000000000, 0.9510565162951535312, 1.000000000000000000, 0.9510565162951535312, 1.000000000000000000, 0.9510565162951535312, 1.000000000000000000, 0.9510565162951535312, 1.000000000000000000, 0.9510565162951535312, 1.000000000000000000, 0.9510565162951535312, 1.000000000000000000, 0.9510565162951535312, 1.000000000000000000, 0.9510565162951535312, 1.000000000000000000, 0.9510565162951535312, 1.000000000000000000, 0.9510565162951535312, 1.000000000000000000, 0.9510565162951535312, 1.000000000000000000, 0.9510565162951535312, 1.000000000000000000, 0.9510565162951535312, 1.000000000000000000, 0.9510565162951535312, 1.000000000000000000, 0.9510565162951535312, 1.000000000000000000, 0.9510565162951535312, 1.000000000000000000, 0.9510565162951535312, 1.000000000000000000, 0.9510565162951535312, 1.000000000000000000, 0.9510565162951535312, 1.000000000000000000, 0.9510565162951535312, 1.000000000000000000, 0.9510565162951535312, 1.000000000000000000, 0.9510565162951535312, 1.000000000000000000, 0.9510565162951535312, 1.000000000000000000, 0.9510565162951535312, 1.000000000000000000, 0.9510565162951535312, 1.000000000000000000, 0.9510565162951535312, 1.000000000000000000, 0.9510565162951535312, 1.000000000000000000, 0.9510565162951535312, 1.000000000000000000, 0.9510565162951535312, 1.000000000000000000, 0.9510565162951535312, 1.000000000000000000, 0.9510565162951535312, 1.000000000000000000, 0.9510565162951535312, 1.000000000000000000, 0.9510565162951535312, 1.000000000000000000, 0.9510565162951535312, 1.000000000000000000, 0.9510565162951535312, 1.000000000000000000, 0.9510565162951535312, 1.000000000000000000, 0.9510565162951535312, 1.000000000000000000, 0.9510565162951535312, 1.000000000000000000, 0.9510565162951535312, 1.000000000000000000, 0.9510565162951535312, 1.000000000000000000, 0.9510565162951535312, 1.000000000000000000, 0.9510565162951535312, 1.000000000000000000, 0.9510565162951535312, 1.000000000000000000, 0.9510565162951535312, 1.000000000000000000, 0.9510565162951535312, 1.000000000000000000, 0.9510565162951535312, 1.000000000000000000, 0.9510565162951535312, 1.000000000000000000, 0.9510565162951535312, 1.000000000000000000, 0.9510565162951535312, 1.000000000000000000, 0.9510565162951535312, 1.000000000000000000, 0.9510565162951535312, 1.000000000000000000, 0.9510565162951535312, 1.000000000000000000, 0.9510565162951535312, 1.000000000000000000, 0.9510565162951535312, 1.000000000000000000, 0.9510565162951535312, 1.000000000000000000, 0.9510565162951535312, 1.000000000000000000, 0.9510565162951535312, 1.000000000000000000, 0.9510565162951535312, 1.000000000000000000, 0.9510565162951535312, 1.000000000000000000, 0.9510565162951535312, 1.000000000000000000, 0.9510565162951535312, 1.000000000000000000, 0.9510565162951535312, 1.000000000000000000, 0.9510565162951535312, 1.000000000000000000, 0.9510565162951535312, 1.000000000000000000, 0.9510565162951535312, 1.000000000000000000, 0.9510565162951535312, 1.000000000000000000, 0.9510565162951535312, 1.000000000000000000, 0.9510565162951535312, 1.000000000000000000, 0.9510565162951535312, 1.000000000000000000, 0.9510565162951535312, 1.000000000000000000, 0.9510565162951535312, 1.000000000000000000, 0.9510565162951535312, 1.000000000000000000, 0.9510565162951535312, 1.000000000000000000, 0.9510565162951535312, 1.000000000000000000, 0.9510565162951535312, 1.000000000000000000, 0.9510565162951535312, 1.000000000000000000, 0.9510565162951535312, 1.000000000000000000, 0.9510565162951535312, 1.000000000000000000, 0.9510565162951535312, 1.000000000000000000, 0.9510565162951535312, 1.000000000000000000, 0.9510565162951535312, 1.000000000000000000, 0.9510565162951535312, 1.000000000000000000, 0.9510565162951535312, 1.000000000000000000, 0.9510565162951535312, 1.000000000000000000, 0.9510565162951535312, 1.000000000000000000, 0.9510565162951535312, 1.000000000000000000, 0.9510565162951535312, 1.000000000000000000, 0.9510565162951535312, 1.000000000000000000, 0.9510565162951535312, 1.000000000000000000, 0.9510565162951535312, 1.000000000000000000, 0.9510565162951535312, 1.000000000000000000, 0.9510565162951535312, 1.000000000000000000, 0.9510565162951535312, 1.000000000000000000, 0.9510565162951535312, 1.000000000000000000, 0.9510565162951535312, 1.000000000000000000, 0.9510565162951535312, 1.000000000000000000, 0.9510565162951535312, 1.000000000000000000, 0.9510565162951535312, 1.000000000000000000, 0.9510565162951535312, 1.000000000000000000, 0.9510565162951535312, 1.000000000000000000, 0.9510565162951535312, 1.000000000000000000, 0.9510565162951535312, 1.000000000000000000, 0.9510565162951535312, 1.000000000000000000, 0.9510565162951535312, 1.000000000000000000, 0.9510565162951535312, 1.000000000000000000, 0.9510565162951535312, 1.000000000000000000, 0.9510565162951535312, 1.000000000000000000, 0.9510565162951535312, 1.000000000000000000, 0.9510565162951535312, 1.000000000000000000, 0.9510565162951535312, 1.000000000000000000, 0.9510565162951535312, 1.000000000000000000, 0.9510565162951535312, 1.000000000000000000, 0.9510565162951535312, 1.000000000000000000, 0.9510565162951535312, 1.000000000000000000, 0.9510565162951535312, 1.000000000000000000, 0.9510565162951535312, 1.000000000000000000, 0.9510565162951535312, 1.000000000000000000, 0.9510565162951535312, 1.000000000000000000, 0.9510565162951535312, 1.000000000000000000, 0.9510565162951535312, 1.000000000000000000, 0.9510565162951535312, 1.000000000000000000, 0.9510565162951535312, 1.000000000000000000, 0.9510565162951535312, 1.000000000000000000, 0.9510565162951535312, 1.000000000000000000, 0.9510565162951535312, 1.000000000000000000, 0.9510565162951535312, 1.000000000000000000, 0.9510565162951535312, 1.000000000000000000, 0.9510565162951535312, 1.000000000000000000, 0.9510565162951535312, 1.000000000000000000, 0.9510565162951535312, 1.000000000000000000, 0.9510565162951535312, 1.000000000000000000, 0.9510565162951535312, 1.000000000000000000, 0.9510565162951535312, 1.000000000000000000, 0.9510565162951535312, 1.000000000000000000, 0.9510565162951535312, 1.000000000000000000, 0.9510565162951535312, 1.000000000000000000, 0.9510565162951535312, 1.000000000000000000, 0.9510565162951535312, 1.000000000000000000, 0.9510565162951535312, 1.000000000000000000, 0.9510565162951535312, 1.000000000000000000, 0.9510565162951535312, 1.000000000000000000, 0.9510565162951535312, 1.000000000000000000, 0.9510565162951535312, 1.000000000000000000, 0.9510565162951535312, 1.000000000000000000, 0.9510565162951535312, 1.000000000000000000, 0.9510565162951535312, 1.000000000000000000, 0.9510565162951535312, 1.000000000000000000, 0.9510565162951535312, 1.000000000000000000, 0.9510565162951535312, 1.000000000000000000, 0.9510565162951535312, 1.000000000000000000, 0.9510565162951535312, 1.000000000000000000, 0.9510565162951535312, 1.000000000000000000, 0.9510565162951535312, 1.000000000000000000, 0.9510565162951535312, 1.000000000000000000, 0.9510565162951535312, 1.000000000000000000, 0.9510565162951535312, 1.000000000000000000, 0.9510565162951535312, 1.000000000000000000, 0.9510565162951535312, 1.000000000000000000, 0.9510565162951535312, 1.000000000000000000, 0.9510565162951535312, 1.000000000000000000, 0.9510565162951535312, 1.000000000000000000, 0.9510565162951535312, 1.000000000000000000, 0.9510565162951535312, 1.000000000000000000, 0.9510565162951535312, 1.000000000000000000, 0.9510565162951535312, 1.000000000000000000, 0.9510565162951535312, 1.000000000000000000, 0.9510565162951535312, 1.000000000000000000, 0.9510565162951535312, 1.000000000000000000, 0.9510565162951535312, 1.000000000000000000, 0.9510565162951535312, 1.000000000000000000, 0.9510565162951535312, 1.000000000000000000, 0.9510565162951535312, 1.000000000000000000, 0.9510565162951535312, 1.000000000000000000, 0.9510565162951535312, 1.000000000000000000, 0.9510565162951535312, 1.000000000000000000, 0.9510565162951535312, 1.000000000000000000, 0.9510565162951535312, 1.000000000000000000, 0.9510565162951535312, 1.000000000000000000, 0.9510565162951535312, 1.000000000000000000, 0.9510565162951535312, 1.000000000000000000, 0.9510565162951535312, 1.000000000000000000, 0.9510565162951535312, 1.000000000000000000, 0.9510565162951535312, 1.000000000000000000, 0.9510565162951535312, 1.000000000000000000, 0.9510565162951535312, 1.000000000000000000, 0.9510565162951535312, 1.000000000000000000, 0.9510565162951535312, 1.000000000000000000, 0.9510565162951535312, 1.000000000000000000, 0.9510565162951535312, 1.000000000000000000, 0.9510565162951535312, 1.000000000000000000, 0.9510565162951535312, 1.000000000000000000, 0.9510565162951535312, 1.000000000000000000, 0.9510565162951535312, 1.000000000000000000, 0.9510565162951535312, 1.000000000000000000, 0.9510565162951535312, 1.000000000000000000, 0.9510565162951535312, 1.000000000000000000, 0.9510565162951535312, 1.000000000000000000, 0.9510565162951535312, 1.000000000000000000, 0.9510565162951535312, 1.000000000000000000, 0.9510565162951535312, 1.000000000000000000, 0.9510565162951535312, 1.000000000000000000, 0.9510565162951535312, 1.000000000000000000, 0.9510565162951535312, 1.000000000000000000, 0.9510565162951535312, 1.000000000000000000, 0.9510565162951535312, 1.000000000000000000, 0.9510565162951535312, 1.000000000000000000, 0.9510565162951535312, 1.000000000000000000, 0.9510565162951535312, 1.000000000000000000, 0.9510565162951535312, 1.000000000000000000, 0.9510565162951535312, 1.000000000000000000, 0.9510565162951535312, 1.000000000000000000, 0.9510565162951535312, 1.000000000000000000, 0.9510565162951535312, 1.000000000000000000, 0.9510565162951535312, 1.000000000000000000, 0.9510565162951535312, 1.000000000000000000, 0.9510565162951535312, 1.000000000000000000, 0.9510565162951535312, 1.000000000000000000, 0.9510565162951535312, 1.000000000000000000, 0.9510565162951535312, 1.000000000000000000, 0.9510565162951535312, 1.000000000000000000, 0.9510565162951535312, 1.000000000000000000, 0.9510565162951535312, 1.000000000000000000, 0.9510565162951535312, 1.000000000000000000, 0.9510565162951535312, 1.000000000000000000, 0.9510565162951535312, 1.000000000000000000, 0.9510565162951535312, 1.000000000000000000, 0.9510565162951535312, 1.000000000000000000, 0.9510565162951535312, 1.000000000000000000, 0.9510565162951535312, 1.000000000000000000, 0.9510565162951535312, 1.000000000000000000, 0.9510565162951535312, 1.000000000000000000, 0.9510565162951535312, 1.000000000000000000, 0.9510565162951535312, 1.000000000000000000, 0.9510565162951535312, 1.000000000000000000, 0.9510565162951535312, 1.000000000000000000, 0.9510565162951535312, 1.000000000000000000, 0.9510565162951535312, 1.000000000000000000, 0.9510565162951535312, 1.000000000000000000, 0.9510565162951535312, 1.000000000000000000, 0.9510565162951535312, 1.000000000000000000, 0.9510565162951535312, 1.000000000000000000, 0.9510565162951535312, 1.000000000000000000, 0.9510565162951535312, 1.000000000000000000, 0.9510565162951535312, 1.000000000000000000, 0.9510565162951535312, 1.000000000000000000, 0.9510565162951535312, 1.000000000000000000, 0.9510565162951535312, 1.000000000000000000, 0.9510565162951535312, 1.000000000000000000, 0.9510565162951535312, 1.000000000000000000, 0.9510565162951535312, 1.000000000000000000, 0.9510565162951535312, 1.000000000000000000, 0.9510565162951535312, 1.000000000000000000, 0.9510565162951535312, 1.000000000000000000, 0.9510565162951535312, 1.000000000000000000, 0.9510565162951535312, 1.000000000000000000, 0.9510565162951535312, 1.000000000000000000, 0.9510565162951535312, 1.000000000000000000, 0.9510565162951535312, 1.000000000000000000, 0.9510565162951535312, 1.000000000000000000, 0.9510565162951535312, 1.000000000000000000, 0.9510565162951535312, 1.000000000000000000, 0.9510565162951535312, 1.000000000000000000, 0.9510565162951535312, 1.000000000000000000, 0.9510565162951535312, 1.000000000000000000, 0.9510565162951535312, 1.000000000000000000, 0.9510565162951535312, 1.000000000000000000, 0.9510565162951535312, 1.000000000000000000, 0.9510565162951535312, 1.000000000000000000, 0.9510565162951535312, 1.000000000000000000, 0.9510565162951535312, 1.000000000000000000, 0.9510565162951535312, 1.000000000000000000, 0.9510565162951535312, 1.000000000000000000, 0.9510565162951535312, 1.000000000000000000, 0.9510565162951535312, 1.000000000000000000, 0.9510565162951535312, 1.000000000000000000, 0.9510565162951535312, 1.000000000000000000, 0.9510565162951535312, 1.000000000000000000, 0.9510565162951535312, 1.000000000000000000, 0.9510565162951535312, 1.000000000000000000, 0.9510565162951535312, 1.000000000000000000, 0.9510565162951535312, 1.000000000000000000, 0.9510565162951535312, 1.000000000000000000, 0.9510565162951535312, 1.000000000000000000, 0.9510565162951535312, 1.000000000000000000, 0.9510565162951535312, 1.000000000000000000, 0.9510565162951535312, 1.000000000000000000, 0.9510565162951535312, 1.000000000000000000, 0.9510565162951535312, 1.000000000000000000, 0.9510565162951535312, 1.000000000000000000, 0.9510565162951535312, 1.000000000000000000, 0.9510565162951535312, 1.000000000000000000, 0.9510565162951535312, 1.000000000000000000, 0.9510565162951535312, 1.000000000000000000, 0.9510565162951535312, 1.000000000000000000, 0.9510565162951535312, 1.000000000000000000, 0.9510565162951535312, 1.000000000000000000, 0.9510565162951535312, 1.000000000000000000, 0.9510565162951535312, 1.000000000000000000, 0.9510565162951535312, 1.000000000000000000, 0.9510565162951535312, 1.000000000000000000, 0.9510565162951535312, 1.000000000000000000, 0.9510565162951535312, 1.000000000000000000, 0.9510565162951535312, 1.000000000000000000, 0.9510565162951535312, 1.000000000000000000, 0.9510565162951535312, 1.000000000000000000, 0.9510565162951535312, 1.000000000000000000, 0.9510565162951535312, 1.000000000000000000, 0.9510565162951535312, 1.000000000000000000, 0.9510565162951535312, 1.000000000000000000, 0.9510565162951535312, 1.000000000000000000, 0.9510565162951535312, 1.000000000000000000, 0.9510565162951535312, 1.000000000000000000, 0.9510565162951535312, 1.000000000000000000, 0.9510565162951535312, 1.000000000000000000, 0.9510565162951535312, 1.000000000000000000, 0.9510565162951535312, 1.000000000000000000, 0.9510565162951535312, 1.000000000000000000, 0.9510565162951535312, 1.000000000000000000, 0.9510565162951535312, 1.000000000000000000, 0.9510565162951535312, 1.000000000000000000, 1.000000000000000000, 1.000000000000000000) ) ) 
 REPRESENTATION_ITEM ( '' )  SURFACE ( )  );
#30713=CARTESIAN_POINT ( 'NONE',  ( 6.500168698208244500, 202.3363017425938324, 22.29886208192143826 ) ) ;
#30717=CARTESIAN_POINT ( 'NONE',  ( 6.444103211791042618, 202.2591342207267644, -0.6988620819214341751 ) ) ;
#30718=CARTESIAN_POINT ( 'NONE',  ( -11.98450388067341876, 203.0532714938636047, 86.34886208192143897 ) ) ;
#30723=CARTESIAN_POINT ( 'NONE',  ( -6.139770520408369237, 215.5359834540460042, 0.9511379180785658471 ) ) ;
#30724=CARTESIAN_POINT ( 'NONE',  ( -3.044812012439970683, 197.4746971517856196, 73.89886208192143613 ) ) ;
#30727=CARTESIAN_POINT ( 'NONE',  ( 6.220909254589536808, 215.4770327129947702, 13.55113791807856849 ) ) ;
#30730=CARTESIAN_POINT ( 'NONE',  ( 6.220909254589536808, 215.4770327129947702, 88.55113791807853829 ) ) ;
#30732=CARTESIAN_POINT ( 'NONE',  ( 3.135527875058820690, 216.4958274776887492, 73.40113791807857524 ) ) ;
#30735=CARTESIAN_POINT ( 'NONE',  ( -9.736236675708031640, 214.0148392665760753, 89.79886208192142760 ) ) ;
#30736=EDGE_CURVE ( 'NONE', #18219, #19921, #22258, .T. ) ;
#30738=CARTESIAN_POINT ( 'NONE',  ( 6.220909254589536808, 215.4770327129947987, 25.55113791807857027 ) ) ;
#30742=CARTESIAN_POINT ( 'NONE',  ( -7.456977232089304408, 196.8216656703010301, 99.05113791807858092 ) ) ;
#30745=CARTESIAN_POINT ( 'NONE',  ( -10.01549611932659545, 210.2015048109875011, 83.64886208192145034 ) ) ;
#30746=CARTESIAN_POINT ( 'NONE',  ( -11.98450388067341876, 203.0532714938636047, 20.34886208192143542 ) ) ;
#30748=CARTESIAN_POINT ( 'NONE',  ( -8.062137200540920645, 212.9164362838581894, 30.80113791807856671 ) ) ;
#30750=CARTESIAN_POINT ( 'NONE',  ( 6.220909254589681581, 198.5229672870052582, 100.4488620819214475 ) ) ;
#30754=CARTESIAN_POINT ( 'NONE',  ( 4.984841277089891776, 200.2242689037093726, 82.44886208192144750 ) ) ;
#30759=CARTESIAN_POINT ( 'NONE',  ( -2.426778023690262742, 214.6231898156240163, 64.10113791807857808 ) ) ;
#30764=CARTESIAN_POINT ( 'NONE',  ( -4.984841277089726574, 200.2242689037092305, 78.05113791807858092 ) ) ;
#30767=CARTESIAN_POINT ( 'NONE',  ( 2.426778023690075337, 214.6231898156240447, 66.39886208192143613 ) ) ;
#30774=CARTESIAN_POINT ( 'NONE',  ( -12.01549611932652972, 203.1486557965464499, 69.35113791807857808 ) ) ;
#30776=CARTESIAN_POINT ( 'NONE',  ( -9.736236675707914401, 199.9851607334237542, 12.20113791807856707 ) ) ;
#30777=CARTESIAN_POINT ( 'NONE',  ( 8.118202686958039038, 212.8392687619912635, 88.70113791807857240 ) ) ;
#30779=CARTESIAN_POINT ( 'NONE',  ( 11.98450388067341876, 210.9467285061363953, 42.84886208192143187 ) ) ;
#30780=CARTESIAN_POINT ( 'NONE',  ( 8.118202686958138514, 201.1607312380088501, 61.29886208192143471 ) ) ;
#30782=CARTESIAN_POINT ( 'NONE',  ( 0.05014649552807549926, 219.6175466908591716, 94.25113791807859798 ) ) ;
#30784=CARTESIAN_POINT ( 'NONE',  ( -8.118202686958039038, 201.1607312380087080, 3.201137918078566180 ) ) ;
#30785=CARTESIAN_POINT ( 'NONE',  ( -9.984503880673420539, 203.7031108863293980, 71.34886208192142476 ) ) ;
#30788=CARTESIAN_POINT ( 'NONE',  ( -12.01549611932659722, 210.8513442034533227, 68.64886208192142192 ) ) ;
#30789=CARTESIAN_POINT ( 'NONE',  ( -0.05014649552810635652, 196.4853777576173002, 92.75113791807858377 ) ) ;
#30792=CARTESIAN_POINT ( 'NONE',  ( 0.05014649552828262524, 198.5883022060938572, 52.74886208192144466 ) ) ;
#30801=CARTESIAN_POINT ( 'NONE',  ( -8.062137200540822946, 201.0835637161416400, 50.19886208192144039 ) ) ;
#30807=CARTESIAN_POINT ( 'NONE',  ( -4.984841277089891776, 213.7757310962905990, 23.94886208192143684 ) ) ;
#30808=CARTESIAN_POINT ( 'NONE',  ( -6.139770520408369237, 215.5359834540460042, 66.95113791807858661 ) ) ;
#30810=CARTESIAN_POINT ( 'NONE',  ( -6.220909254589537696, 198.5229672870051161, 54.05113791807856671 ) ) ;
#30811=CARTESIAN_POINT ( 'NONE',  ( 10.01549611932653860, 210.2015048109876716, 25.85113791807856742 ) ) ;
#30812=CARTESIAN_POINT ( 'NONE',  ( -0.05014649552807731031, 198.5883022060938572, 2.751137918078566003 ) ) ;
#30816=CARTESIAN_POINT ( 'NONE',  ( -3.662846001190052991, 218.4274158808045740, 34.10113791807857098 ) ) ;
#30818=CARTESIAN_POINT ( 'NONE',  ( -3.044812012440131443, 216.5253028482142952, 85.10113791807857808 ) ) ;
#30819=CARTESIAN_POINT ( 'NONE',  ( 3.044812012440130555, 197.4746971517856764, 47.60113791807857098 ) ) ;
#30821=CARTESIAN_POINT ( 'NONE',  ( 3.662846001189864698, 218.4274158808046593, 12.39886208192143613 ) ) ;
#30822=CARTESIAN_POINT ( 'NONE',  ( -0.05014649552828402690, 217.5146222423826714, 30.24886208192143755 ) ) ;
#30825=CARTESIAN_POINT ( 'NONE',  ( -0.05014649552807705357, 194.3824533091408000, 59.75113791807856245 ) ) ;
#30826=CARTESIAN_POINT ( 'NONE',  ( -4.903702542908602524, 213.8346818373418898, 81.95113791807858661 ) ) ;
#30828=CARTESIAN_POINT ( 'NONE',  ( -9.984503880673420539, 203.7031108863293980, 41.34886208192143897 ) ) ;
#30833=CARTESIAN_POINT ( 'NONE',  ( 12.00000000000000711, 207.0476921513415220, 45.99886208192143755 ) ) ;
#30834=ORIENTED_EDGE ( 'NONE', *, *, #1654, .F. ) ;
#30842=CARTESIAN_POINT ( 'NONE',  ( 6.444103211791042618, 202.2591342207267644, 35.30113791807856671 ) ) ;
#30843=EDGE_CURVE ( 'NONE', #13603, #6436, #6706, .T. ) ;
#30845=CARTESIAN_POINT ( 'NONE',  ( 6.139770520408223575, 215.5359834540460611, 15.54886208192143293 ) ) ;
#30848=CARTESIAN_POINT ( 'NONE',  ( 6.500168698208129925, 211.6636982574063381, 58.70113791807857240 ) ) ;
#30851=CARTESIAN_POINT ( 'NONE',  ( 6.220909254589681581, 198.5229672870052582, 100.4488620819214475 ) ) ;
#30853=CARTESIAN_POINT ( 'NONE',  ( -6.220909254589537696, 198.5229672870051161, 39.05113791807856671 ) ) ;
#30855=CARTESIAN_POINT ( 'NONE',  ( -6.220909254589537696, 198.5229672870051161, 30.05113791807856671 ) ) ;
#30863=CARTESIAN_POINT ( 'NONE',  ( -7.456977232089304408, 196.8216656703010301, 3.051137918078566269 ) ) ;
#30866=CARTESIAN_POINT ( 'NONE',  ( 8.118202686958039038, 212.8392687619912635, 46.70113791807857240 ) ) ;
#30874=CARTESIAN_POINT ( 'NONE',  ( -0.05014649552807705357, 194.3824533091408000, 29.75113791807856956 ) ) ;
#30876=CARTESIAN_POINT ( 'NONE',  ( 0.05014649552828275708, 196.4853777576173002, 13.74886208192143400 ) ) ;
#30879=CARTESIAN_POINT ( 'NONE',  ( 3.044812012440130555, 197.4746971517856764, 11.60113791807856742 ) ) ;
#30880=CARTESIAN_POINT ( 'NONE',  ( 6.139770520408368348, 198.4640165459539674, 74.45113791807857240 ) ) ;
#30883=CARTESIAN_POINT ( 'NONE',  ( 2.426778023690075337, 214.6231898156240447, 33.39886208192144323 ) ) ;
#30887=CARTESIAN_POINT ( 'NONE',  ( 7.984503880673485376, 204.3529502787953902, 8.151137918078566358 ) ) ;
#30888=CARTESIAN_POINT ( 'NONE',  ( -3.662846001189865142, 195.5725841191952838, 85.89886208192143613 ) ) ;
#30894=CARTESIAN_POINT ( 'NONE',  ( 6.139770520408368348, 198.4640165459539674, 5.451137918078567068 ) ) ;
#30895=CARTESIAN_POINT ( 'NONE',  ( -9.984503880673420539, 203.7031108863293980, 74.34886208192143897 ) ) ;
#30898=CARTESIAN_POINT ( 'NONE',  ( -8.062137200540920645, 212.9164362838581894, 9.801137918078566713 ) ) ;
#30901=CARTESIAN_POINT ( 'NONE',  ( 10.01549611932653860, 210.2015048109876716, 94.85113791807857808 ) ) ;
#30903=CARTESIAN_POINT ( 'NONE',  ( -6.139770520408369237, 215.5359834540460042, 75.95113791807857240 ) ) ;
#30907=CARTESIAN_POINT ( 'NONE',  ( -3.662846001189865142, 195.5725841191952838, 88.89886208192143613 ) ) ;
#30913=CARTESIAN_POINT ( 'NONE',  ( 11.98450388067348271, 203.0532714938637753, 95.15113791807856103 ) ) ;
#30918=CARTESIAN_POINT ( 'NONE',  ( 10.00000000000000711, 207.0476921513415220, 87.99886208192144466 ) ) ;
#30919=CARTESIAN_POINT ( 'NONE',  ( 3.662846001189864698, 218.4274158808046593, 27.39886208192143613 ) ) ;
#30921=CARTESIAN_POINT ( 'NONE',  ( -3.044812012440131443, 216.5253028482142952, 40.10113791807857098 ) ) ;
#30923=CARTESIAN_POINT ( 'NONE',  ( -6.220909254589682469, 215.4770327129946850, 101.9488620819214333 ) ) ;
#30925=EDGE_LOOP ( 'NONE', ( #18263, #5307, #1963, #28778 ) ) ;
#30926=CARTESIAN_POINT ( 'NONE',  ( 8.000000000000008882, 207.0476921513415220, 78.99886208192144466 ) ) ;
#30934=CARTESIAN_POINT ( 'NONE',  ( -0.05014649552807731031, 198.5883022060938572, 56.75113791807857666 ) ) ;
#30937=CARTESIAN_POINT ( 'NONE',  ( -7.984503880673488041, 209.6470497212046098, 84.65113791807856103 ) ) ;
#30939=AXIS2_PLACEMENT_3D ( 'NONE', #15973, #31644, #11196 ) ;
#30941=CARTESIAN_POINT ( 'NONE',  ( 2.517493886309087436, 199.4062855549015865, 64.59886208192142476 ) ) ;
#30942=CARTESIAN_POINT ( 'NONE',  ( -9.984503880673475606, 210.2968891136704315, 3.651137918078565470 ) ) ;
#30947=CARTESIAN_POINT ( 'NONE',  ( -12.00000000000000711, 207.0476921513413515, 66.50113791807856956 ) ) ;
#30952=CARTESIAN_POINT ( 'NONE',  ( -12.00000000000000711, 207.0476921513413515, 12.50113791807856600 ) ) ;
#30953=CARTESIAN_POINT ( 'NONE',  ( 10.01549611932653860, 210.2015048109876716, 88.85113791807857808 ) ) ;
#30956=CARTESIAN_POINT ( 'NONE',  ( 7.456977232089471386, 196.8216656703012006, 55.44886208192143329 ) ) ;
#30957=CARTESIAN_POINT ( 'NONE',  ( -6.139770520408224463, 198.4640165459539105, 56.04886208192142760 ) ) ;
#30959=CARTESIAN_POINT ( 'NONE',  ( 7.456977232089302632, 217.1783343296989131, 94.55113791807855250 ) ) ;
#30961=CARTESIAN_POINT ( 'NONE',  ( 8.062137200540920645, 201.0835637161417822, -0.6988620819214342861 ) ) ;
#30962=CARTESIAN_POINT ( 'NONE',  ( 6.139770520408223575, 215.5359834540460611, 69.54886208192142760 ) ) ;
#30965=CARTESIAN_POINT ( 'NONE',  ( -9.736236675708031640, 214.0148392665760753, 77.79886208192142760 ) ) ;
#30966=CARTESIAN_POINT ( 'NONE',  ( 0.05014649552810505201, 217.5146222423826714, 88.25113791807858377 ) ) ;
#30969=CARTESIAN_POINT ( 'NONE',  ( -0.05014649552828365914, 215.4116977939061144, 54.24886208192144466 ) ) ;
#30978=CARTESIAN_POINT ( 'NONE',  ( 9.984503880673420539, 210.2968891136705167, 51.84886208192143897 ) ) ;
#30985=CARTESIAN_POINT ( 'NONE',  ( -4.903702542908436435, 200.1653181626580249, 32.04886208192144181 ) ) ;
#30986=CARTESIAN_POINT ( 'NONE',  ( -8.062137200540920645, 212.9164362838581894, 66.80113791807858092 ) ) ;
#30988=CARTESIAN_POINT ( 'NONE',  ( 8.118202686958039038, 212.8392687619912635, 58.70113791807857240 ) ) ;
#30989=CARTESIAN_POINT ( 'NONE',  ( 6.139770520408368348, 198.4640165459539674, 29.45113791807856529 ) ) ;
#30990=CARTESIAN_POINT ( 'NONE',  ( -6.444103211791042618, 211.7408657792732356, 15.80113791807856849 ) ) ;
#30994=CARTESIAN_POINT ( 'NONE',  ( 0.05014649552807549926, 219.6175466908591716, 34.25113791807857666 ) ) ;
#30997=CARTESIAN_POINT ( 'NONE',  ( 8.118202686958039038, 212.8392687619912635, 82.70113791807857240 ) ) ;
#30998=CARTESIAN_POINT ( 'NONE',  ( -6.220909254589537696, 198.5229672870051445, 57.05113791807857382 ) ) ;
#31000=CARTESIAN_POINT ( 'NONE',  ( -3.753561863808878130, 218.3979405102790281, 24.09886208192143897 ) ) ;
#31001=CARTESIAN_POINT ( 'NONE',  ( 6.220909254589680693, 198.5229672870052582, 31.44886208192142973 ) ) ;
#31004=CARTESIAN_POINT ( 'NONE',  ( 9.680171189290831535, 199.9079932115568852, 65.30113791807858092 ) ) ;
#31006=CARTESIAN_POINT ( 'NONE',  ( 8.000000000000008882, 206.9523078486586485, 80.00113791807856956 ) ) ;
#31008=CARTESIAN_POINT ( 'NONE',  ( 8.118202686958138514, 201.1607312380088501, 43.29886208192143471 ) ) ;
#31011=CARTESIAN_POINT ( 'NONE',  ( -12.01549611932659722, 210.8513442034533227, 53.64886208192142902 ) ) ;
#31012=VERTEX_POINT ( 'NONE', #12826 ) ;
#31017=CARTESIAN_POINT ( 'NONE',  ( -8.015496119326531499, 204.4483345814780364, 42.35113791807857098 ) ) ;
#31018=CARTESIAN_POINT ( 'NONE',  ( -8.118202686958138514, 212.8392687619910930, 26.79886208192143826 ) ) ;
#31024=CARTESIAN_POINT ( 'NONE',  ( -8.000000000000008882, 206.9523078486584780, 2.498862081921435330 ) ) ;
#31025=CARTESIAN_POINT ( 'NONE',  ( -0.05014649552810635652, 196.4853777576173002, 44.75113791807858377 ) ) ;
#31028=CARTESIAN_POINT ( 'NONE',  ( -8.118202686958039038, 201.1607312380087080, 27.20113791807856884 ) ) ;
#31029=CARTESIAN_POINT ( 'NONE',  ( 9.984503880673420539, 210.2968891136705736, 102.8488620819214390 ) ) ;
#31030=CARTESIAN_POINT ( 'NONE',  ( -8.000000000000008882, 206.9523078486584780, 83.49886208192144466 ) ) ;
#31034=CARTESIAN_POINT ( 'NONE',  ( 0.05014649552807549926, 219.6175466908591716, 10.25113791807856600 ) ) ;
#31037=CARTESIAN_POINT ( 'NONE',  ( -6.139770520408369237, 215.5359834540460042, 60.95113791807857950 ) ) ;
#31043=CARTESIAN_POINT ( 'NONE',  ( 3.662846001190051659, 195.5725841191953691, 38.60113791807855677 ) ) ;
#31046=CARTESIAN_POINT ( 'NONE',  ( -9.984503880673420539, 203.7031108863293980, 11.34886208192143187 ) ) ;
#31049=CARTESIAN_POINT ( 'NONE',  ( 10.00000000000000711, 206.9523078486586201, 8.001137918078566003 ) ) ;
#31050=CARTESIAN_POINT ( 'NONE',  ( 8.118202686958039038, 212.8392687619912635, 67.70113791807858661 ) ) ;
#31052=CARTESIAN_POINT ( 'NONE',  ( 2.426778023690075337, 214.6231898156240447, 30.39886208192143613 ) ) ;
#31056=CARTESIAN_POINT ( 'NONE',  ( -2.426778023690262742, 214.6231898156240163, 10.10113791807856742 ) ) ;
#31057=CARTESIAN_POINT ( 'NONE',  ( 7.375838497908012492, 217.2372850707501186, 99.54886208192144181 ) ) ;
#31062=CARTESIAN_POINT ( 'NONE',  ( -9.984503880673473830, 210.2968891136704315, 6.651137918078564581 ) ) ;
#31064=CARTESIAN_POINT ( 'NONE',  ( 10.00000000000000711, 207.0476921513415220, 75.99886208192144466 ) ) ;
#31067=CARTESIAN_POINT ( 'NONE',  ( -0.05014649552810635652, 196.4853777576173002, 14.75113791807856245 ) ) ;
#31071=CARTESIAN_POINT ( 'NONE',  ( -8.062137200540920645, 212.9164362838581894, 99.80113791807858092 ) ) ;
#31073=CARTESIAN_POINT ( 'NONE',  ( -3.135527875058821579, 197.5041725223112223, 86.90113791807857524 ) ) ;
#31077=CARTESIAN_POINT ( 'NONE',  ( 7.456977232089471386, 196.8216656703012006, 100.4488620819214475 ) ) ;
#31082=CARTESIAN_POINT ( 'NONE',  ( 3.753561863808689836, 218.3979405102790565, 100.4011379180785895 ) ) ;
#31085=CARTESIAN_POINT ( 'NONE',  ( 3.044812012439969795, 216.5253028482143520, 84.39886208192143613 ) ) ;
#31087=CARTESIAN_POINT ( 'NONE',  ( -0.05014649552828442242, 219.6175466908591716, 21.24886208192143755 ) ) ;
#31089=CARTESIAN_POINT ( 'NONE',  ( 3.135527875058820690, 216.4958274776887492, 40.40113791807857524 ) ) ;
#31091=CARTESIAN_POINT ( 'NONE',  ( -4.903702542908436435, 200.1653181626580249, 5.048862081921433820 ) ) ;
#31094=CARTESIAN_POINT ( 'NONE',  ( 4.984841277089891776, 200.2242689037093726, 85.44886208192144750 ) ) ;
#31096=CARTESIAN_POINT ( 'NONE',  ( 0.05014649552807626948, 215.4116977939061144, 34.25113791807857666 ) ) ;
#31098=ORIENTED_EDGE ( 'NONE', *, *, #15338, .F. ) ;
#31101=CARTESIAN_POINT ( 'NONE',  ( 8.015496119326531499, 209.5516654185219636, 85.85113791807857808 ) ) ;
#31105=CARTESIAN_POINT ( 'NONE',  ( -4.903702542908436435, 200.1653181626580249, 59.04886208192144181 ) ) ;
#31106=DIRECTION ( 'NONE',  ( -0.1461455375466716444, 0.9854922318508084755, -0.08629335326029916042 ) ) ;
#31109=CARTESIAN_POINT ( 'NONE',  ( -6.139770520408368348, 215.5359834540460042, 3.951137918078565736 ) ) ;
#31113=CARTESIAN_POINT ( 'NONE',  ( 11.98450388067348271, 203.0532714938637753, 68.15113791807856103 ) ) ;
#31115=CARTESIAN_POINT ( 'NONE',  ( 11.98450388067348271, 203.0532714938637753, 8.151137918078566358 ) ) ;
#31116=CARTESIAN_POINT ( 'NONE',  ( -9.984503880673475606, 210.2968891136704315, 87.65113791807856103 ) ) ;
#31117=CARTESIAN_POINT ( 'NONE',  ( 3.753561863808876797, 195.6020594897209719, 49.59886208192143897 ) ) ;
#31118=CARTESIAN_POINT ( 'NONE',  ( -10.01549611932659545, 210.2015048109875011, 53.64886208192142902 ) ) ;
#31119=CARTESIAN_POINT ( 'NONE',  ( -3.662846001190052991, 218.4274158808045740, 100.1011379180785781 ) ) ;
#31121=CARTESIAN_POINT ( 'NONE',  ( -6.220909254589537696, 198.5229672870051161, 12.05113791807856671 ) ) ;
#31122=CARTESIAN_POINT ( 'NONE',  ( -8.118202686958138514, 212.8392687619910930, 83.79886208192144181 ) ) ;
#31124=CARTESIAN_POINT ( 'NONE',  ( 7.375838497908012492, 217.2372850707501186, 78.54886208192142760 ) ) ;
#31125=CARTESIAN_POINT ( 'NONE',  ( 9.984503880673470277, 203.7031108863295401, 95.15113791807854682 ) ) ;
#31128=CARTESIAN_POINT ( 'NONE',  ( 2.517493886309087436, 199.4062855549015865, 52.59886208192143897 ) ) ;
#31135=CARTESIAN_POINT ( 'NONE',  ( 8.062137200540822946, 212.9164362838583315, 48.69886208192144039 ) ) ;
#31139=CARTESIAN_POINT ( 'NONE',  ( -0.05014649552828365914, 215.4116977939061144, 36.24886208192143755 ) ) ;
#31140=CARTESIAN_POINT ( 'NONE',  ( -9.984503880673473830, 210.2968891136704315, 72.65113791807857524 ) ) ;
#31142=CARTESIAN_POINT ( 'NONE',  ( 3.135527875058820690, 216.4958274776887492, 58.40113791807857524 ) ) ;
#31144=CARTESIAN_POINT ( 'NONE',  ( -10.01549611932653860, 203.7984951890123284, 24.35113791807855677 ) ) ;
#31145=CARTESIAN_POINT ( 'NONE',  ( -4.984841277089726574, 200.2242689037092305, 15.05113791807856849 ) ) ;
#31149=CARTESIAN_POINT ( 'NONE',  ( -3.662846001190052991, 218.4274158808045740, 43.10113791807857098 ) ) ;
#31151=CARTESIAN_POINT ( 'NONE',  ( -10.01549611932653860, 203.7984951890123284, 84.35113791807856387 ) ) ;
#31153=CARTESIAN_POINT ( 'NONE',  ( -8.118202686958039038, 201.1607312380087080, 54.20113791807857240 ) ) ;
#31155=CARTESIAN_POINT ( 'NONE',  ( -7.456977232089471386, 217.1783343296987709, 23.94886208192143684 ) ) ;
#31156=CARTESIAN_POINT ( 'NONE',  ( 9.984503880673420539, 210.2968891136705736, 27.84886208192143187 ) ) ;
#31158=CARTESIAN_POINT ( 'NONE',  ( -12.00000000000000711, 207.0476921513413515, 72.50113791807856956 ) ) ;
#31159=CARTESIAN_POINT ( 'NONE',  ( 7.984503880673485376, 204.3529502787953902, 86.15113791807856103 ) ) ;
#31161=CARTESIAN_POINT ( 'NONE',  ( -8.062137200540822946, 201.0835637161416400, 41.19886208192144039 ) ) ;
#31164=CARTESIAN_POINT ( 'NONE',  ( 12.00000000000000711, 207.0476921513415220, 54.99886208192144466 ) ) ;
#31165=ORIENTED_EDGE ( 'NONE', *, *, #4518, .T. ) ;
#31170=CARTESIAN_POINT ( 'NONE',  ( -4.984841277089726574, 200.2242689037092305, 39.05113791807855961 ) ) ;
#31172=APPLICATION_CONTEXT ( 'automotive_design' ) ;
#31173=CARTESIAN_POINT ( 'NONE',  ( -8.062137200540822946, 201.0835637161416400, 26.19886208192143684 ) ) ;
#31176=DIRECTION ( 'NONE',  ( 0.5559124511712782990, 1.006869472843640094E-17, 0.8312408475482547798 ) ) ;
#31180=CARTESIAN_POINT ( 'NONE',  ( -2.426778023690076225, 199.3768101843759553, 4.898862081921435241 ) ) ;
#31183=CARTESIAN_POINT ( 'NONE',  ( -6.220909254589537696, 198.5229672870051161, 45.05113791807855961 ) ) ;
#31185=CARTESIAN_POINT ( 'NONE',  ( 6.139770520408368348, 198.4640165459539674, 26.45113791807856884 ) ) ;
#31186=CARTESIAN_POINT ( 'NONE',  ( 10.00000000000000711, 207.0476921513415220, 102.9988620819214447 ) ) ;
#31190=CARTESIAN_POINT ( 'NONE',  ( 8.000000000000008882, 207.0476921513415220, 96.99886208192143044 ) ) ;
#31194=CARTESIAN_POINT ( 'NONE',  ( 7.375838497908181246, 196.7627149292499666, 5.451137918078566180 ) ) ;
#31197=CARTESIAN_POINT ( 'NONE',  ( 10.00000000000000711, 206.9523078486586201, 56.00113791807856956 ) ) ;
#31205=CARTESIAN_POINT ( 'NONE',  ( -11.98450388067348804, 210.9467285061362247, 36.65113791807856103 ) ) ;
#31207=CARTESIAN_POINT ( 'NONE',  ( 9.984503880673420539, 210.2968891136705167, 9.848862081921435419 ) ) ;
#31212=CARTESIAN_POINT ( 'NONE',  ( -8.118202686958039038, 201.1607312380087080, 12.20113791807856707 ) ) ;
#31213=CARTESIAN_POINT ( 'NONE',  ( -9.984503880673473830, 210.2968891136704315, 72.65113791807857524 ) ) ;
#31216=CARTESIAN_POINT ( 'NONE',  ( 2.517493886309087436, 199.4062855549015865, 34.59886208192143897 ) ) ;
#31220=CARTESIAN_POINT ( 'NONE',  ( 8.000000000000008882, 206.9523078486586485, 11.00113791807856600 ) ) ;
#31222=CARTESIAN_POINT ( 'NONE',  ( -12.01549611932659722, 210.8513442034533227, 98.64886208192146455 ) ) ;
#31227=CARTESIAN_POINT ( 'NONE',  ( 10.01549611932653860, 210.2015048109876716, 10.85113791807856387 ) ) ;
#31229=CARTESIAN_POINT ( 'NONE',  ( -8.062137200540822946, 201.0835637161416400, 83.19886208192143329 ) ) ;
#31233=CARTESIAN_POINT ( 'NONE',  ( 10.00000000000000711, 206.9523078486586201, 14.00113791807856600 ) ) ;
#31238=CARTESIAN_POINT ( 'NONE',  ( -8.062137200540920645, 212.9164362838581894, 81.80113791807858092 ) ) ;
#31242=CARTESIAN_POINT ( 'NONE',  ( 11.98450388067341876, 210.9467285061363953, 96.84886208192143897 ) ) ;
#31247=CARTESIAN_POINT ( 'NONE',  ( -9.680171189290831535, 214.0920067884431148, 93.80113791807858092 ) ) ;
#31250=CARTESIAN_POINT ( 'NONE',  ( -8.118202686958138514, 212.8392687619910930, 86.79886208192142760 ) ) ;
#31251=CARTESIAN_POINT ( 'NONE',  ( -0.05014649552828442242, 219.6175466908591716, 24.24886208192144110 ) ) ;
#31253=CARTESIAN_POINT ( 'NONE',  ( -6.139770520408369237, 215.5359834540460042, 45.95113791807857950 ) ) ;
#31255=CARTESIAN_POINT ( 'NONE',  ( -6.444103211790928043, 202.2591342207265939, 5.198862081921435063 ) ) ;
#31260=CARTESIAN_POINT ( 'NONE',  ( 6.444103211790928043, 211.7408657792734061, 90.69886208192143329 ) ) ;
#31261=VECTOR ( 'NONE', #22789, 1000.000000000000227 ) ;
#31265=CARTESIAN_POINT ( 'NONE',  ( 6.444103211791042618, 202.2591342207267644, 26.30113791807856316 ) ) ;
#31271=CARTESIAN_POINT ( 'NONE',  ( 2.517493886308900919, 214.5937144450984420, 91.40113791807857524 ) ) ;
#31276=CARTESIAN_POINT ( 'NONE',  ( -6.444103211790928043, 202.2591342207265939, 59.19886208192144750 ) ) ;
#31279=CARTESIAN_POINT ( 'NONE',  ( 10.01549611932653860, 210.2015048109876716, 4.851137918078564759 ) ) ;
#31283=CARTESIAN_POINT ( 'NONE',  ( -7.456977232089304408, 196.8216656703010301, 72.05113791807858092 ) ) ;
#31285=CARTESIAN_POINT ( 'NONE',  ( -9.736236675707914401, 199.9851607334237542, 6.201137918078565292 ) ) ;
#31286=CARTESIAN_POINT ( 'NONE',  ( 10.01549611932653860, 210.2015048109876716, 91.85113791807856387 ) ) ;
#31288=CARTESIAN_POINT ( 'NONE',  ( -0.05014649552828442242, 219.6175466908591716, 51.24886208192143755 ) ) ;
#31289=CARTESIAN_POINT ( 'NONE',  ( -3.044812012439970683, 197.4746971517856196, 61.89886208192143613 ) ) ;
#31290=CARTESIAN_POINT ( 'NONE',  ( 12.01549611932652972, 210.8513442034534933, 91.85113791807857808 ) ) ;
#31292=CARTESIAN_POINT ( 'NONE',  ( 6.220909254589536808, 215.4770327129947702, 10.55113791807856138 ) ) ;
#31293=CARTESIAN_POINT ( 'NONE',  ( 6.220909254589681581, 198.5229672870052582, 82.44886208192141908 ) ) ;
#31295=CARTESIAN_POINT ( 'NONE',  ( -9.680171189290716072, 199.9079932115567146, 80.19886208192143329 ) ) ;
#31296=CARTESIAN_POINT ( 'NONE',  ( -9.984503880673473830, 210.2968891136704315, 99.65113791807853261 ) ) ;
#31299=CARTESIAN_POINT ( 'NONE',  ( 2.517493886309087436, 199.4062855549015865, 61.59886208192145318 ) ) ;
#31306=CARTESIAN_POINT ( 'NONE',  ( -3.044812012439970683, 197.4746971517856196, 55.89886208192143613 ) ) ;
#31311=CARTESIAN_POINT ( 'NONE',  ( 8.000000000000008882, 207.0476921513415220, 36.99886208192143044 ) ) ;
#31312=CARTESIAN_POINT ( 'NONE',  ( 9.984503880673470277, 203.7031108863295401, 77.15113791807857524 ) ) ;
#31314=CARTESIAN_POINT ( 'NONE',  ( -3.044812012440131443, 216.5253028482142952, 61.10113791807857098 ) ) ;
#31315=CARTESIAN_POINT ( 'NONE',  ( 10.01549611932653860, 210.2015048109876716, 28.85113791807855677 ) ) ;
#31316=CARTESIAN_POINT ( 'NONE',  ( -4.903702542908602524, 213.8346818373418898, 18.95113791807856529 ) ) ;
#31320=CARTESIAN_POINT ( 'NONE',  ( 0.05014649552807549926, 219.6175466908591716, 43.25113791807856245 ) ) ;
#31322=CARTESIAN_POINT ( 'NONE',  ( -8.118202686958039038, 201.1607312380087080, 87.20113791807858661 ) ) ;
#31323=CARTESIAN_POINT ( 'NONE',  ( 9.984503880673473830, 203.7031108863295401, 56.15113791807856813 ) ) ;
#31324=CARTESIAN_POINT ( 'NONE',  ( -12.01549611932659722, 210.8513442034533227, 23.64886208192143968 ) ) ;
#31325=CARTESIAN_POINT ( 'NONE',  ( -6.220909254589682469, 215.4770327129947134, 23.94886208192143329 ) ) ;
#31327=CARTESIAN_POINT ( 'NONE',  ( -12.00000000000000711, 207.0476921513413515, 66.50113791807856956 ) ) ;
#31328=CARTESIAN_POINT ( 'NONE',  ( -0.05014649552807731031, 198.5883022060938572, 89.75113791807858377 ) ) ;
#31329=CARTESIAN_POINT ( 'NONE',  ( 6.220909254589681581, 198.5229672870052582, 52.44886208192143329 ) ) ;
#31332=CARTESIAN_POINT ( 'NONE',  ( -3.662846001189865142, 195.5725841191952838, 55.89886208192143613 ) ) ;
#31337=CARTESIAN_POINT ( 'NONE',  ( 4.984841277089725686, 213.7757310962907411, 40.55113791807856671 ) ) ;
#31341=CARTESIAN_POINT ( 'NONE',  ( 3.135527875058981895, 197.5041725223112792, 25.59886208192143897 ) ) ;
#31347=CARTESIAN_POINT ( 'NONE',  ( -2.517493886309087880, 214.5937144450984135, 9.098862081921435419 ) ) ;
#31348=CARTESIAN_POINT ( 'NONE',  ( -8.118202686958039038, 201.1607312380087080, 45.20113791807857240 ) ) ;
#31350=CARTESIAN_POINT ( 'NONE',  ( 3.135527875058820690, 216.4958274776887492, 31.40113791807857524 ) ) ;
#31351=CYLINDRICAL_SURFACE ( 'NONE', #23346, 0.9999999999999953371 ) ;
#31353=CARTESIAN_POINT ( 'NONE',  ( -2.517493886309087880, 214.5937144450984135, 93.09886208192145318 ) ) ;
#31357=CARTESIAN_POINT ( 'NONE',  ( 9.736236675707914401, 214.0148392665762458, 7.701137918078567068 ) ) ;
#31360=CARTESIAN_POINT ( 'NONE',  ( 3.135527875058820690, 216.4958274776887492, 58.40113791807857524 ) ) ;
#31361=CARTESIAN_POINT ( 'NONE',  ( -0.05014649552810635652, 196.4853777576173002, 26.75113791807856956 ) ) ;
#31366=CARTESIAN_POINT ( 'NONE',  ( 3.044812012439969795, 216.5253028482143520, 3.398862081921434797 ) ) ;
#31369=CARTESIAN_POINT ( 'NONE',  ( 12.00000000000000711, 206.9523078486586485, 38.00113791807857666 ) ) ;
#31370=CARTESIAN_POINT ( 'NONE',  ( -9.984503880673420539, 203.7031108863293980, 23.34886208192142831 ) ) ;
#31374=CARTESIAN_POINT ( 'NONE',  ( 6.139770520408368348, 198.4640165459539674, 71.45113791807857240 ) ) ;
#31376=CARTESIAN_POINT ( 'NONE',  ( -10.00000000000019362, 205.9534653805592654, 104.4507591396482127 ) ) ;
#31379=CARTESIAN_POINT ( 'NONE',  ( 6.444103211791042618, 202.2591342207267644, 17.30113791807856671 ) ) ;
#31382=CARTESIAN_POINT ( 'NONE',  ( -3.753561863808878130, 218.3979405102790281, 99.09886208192145318 ) ) ;
#31387=CARTESIAN_POINT ( 'NONE',  ( -6.139770520408369237, 215.5359834540460042, 3.951137918078566180 ) ) ;
#31389=CARTESIAN_POINT ( 'NONE',  ( 8.118202686958138514, 201.1607312380088501, 85.29886208192144181 ) ) ;
#31392=CARTESIAN_POINT ( 'NONE',  ( 3.135527875058820690, 216.4958274776887492, 10.40113791807856636 ) ) ;
#31397=CARTESIAN_POINT ( 'NONE',  ( -10.01549611932653860, 203.7984951890123284, 99.35113791807857808 ) ) ;
#31399=CARTESIAN_POINT ( 'NONE',  ( 3.044812012440130555, 197.4746971517856764, 80.60113791807857808 ) ) ;
#31402=CARTESIAN_POINT ( 'NONE',  ( 9.680171189290716072, 214.0920067884432854, 93.69886208192144750 ) ) ;
#31407=CARTESIAN_POINT ( 'NONE',  ( 7.375838497908012492, 217.2372850707501186, 3.548862081921434264 ) ) ;
#31413=CARTESIAN_POINT ( 'NONE',  ( -3.135527875058982783, 216.4958274776886924, 96.09886208192143897 ) ) ;
#31414=CARTESIAN_POINT ( 'NONE',  ( 11.98450388067341876, 210.9467285061363953, 18.84886208192143187 ) ) ;
#31416=CARTESIAN_POINT ( 'NONE',  ( 8.062137200540920645, 201.0835637161417822, 38.30113791807857382 ) ) ;
#31419=CARTESIAN_POINT ( 'NONE',  ( -10.00000000000000711, 206.9523078486584495, 104.4988620819214447 ) ) ;
#31423=CARTESIAN_POINT ( 'NONE',  ( 6.444103211790928043, 211.7408657792734061, 93.69886208192144750 ) ) ;
#31424=CARTESIAN_POINT ( 'NONE',  ( 7.984503880673485376, 204.3529502787953902, 32.15113791807857524 ) ) ;
#31431=CARTESIAN_POINT ( 'NONE',  ( 6.444103211791042618, 202.2591342207267644, 89.30113791807858092 ) ) ;
#31435=CARTESIAN_POINT ( 'NONE',  ( -8.015496119326597224, 209.5516654185217362, 59.64886208192145034 ) ) ;
#31446=CARTESIAN_POINT ( 'NONE',  ( -12.00000000000000711, 207.0476921513413515, 69.50113791807856956 ) ) ;
#31449=CARTESIAN_POINT ( 'NONE',  ( 6.220909254589536808, 215.4770327129947987, 85.55113791807856671 ) ) ;
#31451=CARTESIAN_POINT ( 'NONE',  ( -9.736236675708031640, 214.0148392665760753, 50.79886208192143471 ) ) ;
#31452=CARTESIAN_POINT ( 'NONE',  ( 8.062137200540822946, 212.9164362838583315, 63.69886208192143329 ) ) ;
#31453=CARTESIAN_POINT ( 'NONE',  ( 3.662846001190051659, 195.5725841191953691, 92.60113791807857808 ) ) ;
#31456=CARTESIAN_POINT ( 'NONE',  ( 10.00000000000000711, 206.9523078486586201, 14.00113791807856600 ) ) ;
#31458=CARTESIAN_POINT ( 'NONE',  ( -10.00000000000000711, 206.9523078486584495, 77.49886208192144466 ) ) ;
#31461=CARTESIAN_POINT ( 'NONE',  ( -10.00000000000000711, 207.0476921513413515, 96.50113791807856956 ) ) ;
#31463=CARTESIAN_POINT ( 'NONE',  ( -2.517493886309087880, 214.5937144450984135, 57.09886208192145318 ) ) ;
#31471=CARTESIAN_POINT ( 'NONE',  ( -2.517493886308901807, 199.4062855549015012, 56.90113791807858235 ) ) ;
#31472=( NAMED_UNIT ( * ) SI_UNIT ( $, .STERADIAN. ) SOLID_ANGLE_UNIT ( ) );
#31475=CARTESIAN_POINT ( 'NONE',  ( -0.05014649552828365914, 215.4116977939061144, 33.24886208192144466 ) ) ;
#31477=CARTESIAN_POINT ( 'NONE',  ( 3.135527875058820690, 216.4958274776887492, 76.40113791807857524 ) ) ;
#31479=CARTESIAN_POINT ( 'NONE',  ( 6.139770520408368348, 198.4640165459539674, 59.45113791807855819 ) ) ;
#31481=CIRCLE ( 'NONE', #32530, 0.9999999999999941158 ) ;
#31482=CARTESIAN_POINT ( 'NONE',  ( -8.118202686958039038, 201.1607312380087080, 30.20113791807856884 ) ) ;
#31483=CARTESIAN_POINT ( 'NONE',  ( 6.500168698208129925, 211.6636982574063381, 10.70113791807856529 ) ) ;
#31487=CARTESIAN_POINT ( 'NONE',  ( -0.05014649552807705357, 194.3824533091408000, 35.75113791807857666 ) ) ;
#31489=CARTESIAN_POINT ( 'NONE',  ( -0.05014649552810635652, 196.4853777576173002, 83.75113791807856956 ) ) ;
#31490=CARTESIAN_POINT ( 'NONE',  ( -8.062137200540920645, 212.9164362838581894, 60.80113791807857382 ) ) ;
#31492=CARTESIAN_POINT ( 'NONE',  ( 7.456977232089471386, 196.8216656703012006, 25.44886208192143684 ) ) ;
#31493=CARTESIAN_POINT ( 'NONE',  ( -10.01549611932659545, 210.2015048109875011, 26.64886208192143258 ) ) ;
#31495=CARTESIAN_POINT ( 'NONE',  ( 0.05014649552807549926, 219.6175466908591716, 64.25113791807856956 ) ) ;
#31496=CARTESIAN_POINT ( 'NONE',  ( 2.517493886308900919, 214.5937144450984420, 85.40113791807856103 ) ) ;
#31497=CARTESIAN_POINT ( 'NONE',  ( -0.05014649552828403384, 217.5146222423826714, 54.24886208192142334 ) ) ;
#31500=CARTESIAN_POINT ( 'NONE',  ( -9.736236675708031640, 214.0148392665760753, 56.79886208192143471 ) ) ;
#31506=CARTESIAN_POINT ( 'NONE',  ( 0.05014649552807626948, 215.4116977939061144, 40.25113791807856956 ) ) ;
#31508=CARTESIAN_POINT ( 'NONE',  ( 0.05014649552828275708, 196.4853777576173002, 19.74886208192143044 ) ) ;
#31514=CARTESIAN_POINT ( 'NONE',  ( 7.984503880673422316, 209.6470497212048372, 6.848862081921435419 ) ) ;
#31515=CARTESIAN_POINT ( 'NONE',  ( 3.044812012440130555, 197.4746971517856764, 50.60113791807857808 ) ) ;
#31516=CARTESIAN_POINT ( 'NONE',  ( -3.135527875058821579, 197.5041725223112223, 23.90113791807856813 ) ) ;
#31519=CARTESIAN_POINT ( 'NONE',  ( 0.05014649552828262524, 198.5883022060938572, 88.74886208192143044 ) ) ;
#31523=CARTESIAN_POINT ( 'NONE',  ( 12.01549611932652972, 210.8513442034534933, 10.85113791807856565 ) ) ;
#31527=CARTESIAN_POINT ( 'NONE',  ( 3.044812012440130555, 197.4746971517856764, 53.60113791807857098 ) ) ;
#31528=CARTESIAN_POINT ( 'NONE',  ( -10.01549611932653860, 203.7984951890123000, 30.35113791807856742 ) ) ;
#31533=CARTESIAN_POINT ( 'NONE',  ( -0.05014649552807705357, 194.3824533091408000, 41.75113791807856245 ) ) ;
#31536=CARTESIAN_POINT ( 'NONE',  ( 3.044812012439969795, 216.5253028482143520, 24.39886208192143613 ) ) ;
#31540=CARTESIAN_POINT ( 'NONE',  ( -8.062137200540920645, 212.9164362838581894, 69.80113791807856671 ) ) ;
#31544=CARTESIAN_POINT ( 'NONE',  ( -4.984841277089726574, 200.2242689037092305, 18.05113791807856316 ) ) ;
#31546=CARTESIAN_POINT ( 'NONE',  ( -3.662846001189865142, 195.5725841191952838, 100.8988620819214361 ) ) ;
#31551=CARTESIAN_POINT ( 'NONE',  ( -8.062137200540920645, 212.9164362838581894, 3.801137918078565825 ) ) ;
#31552=CARTESIAN_POINT ( 'NONE',  ( -3.135527875058982783, 216.4958274776886924, 84.09886208192143897 ) ) ;
#31555=CARTESIAN_POINT ( 'NONE',  ( -6.220909254589537696, 198.5229672870051161, 24.05113791807855961 ) ) ;
#31558=CARTESIAN_POINT ( 'NONE',  ( -3.135527875058821579, 197.5041725223112223, 98.90113791807857524 ) ) ;
#31560=CARTESIAN_POINT ( 'NONE',  ( -10.01549611932653860, 203.7984951890123284, 84.35113791807856387 ) ) ;
#31563=CARTESIAN_POINT ( 'NONE',  ( -9.680171189290716072, 199.9079932115567146, 98.19886208192144750 ) ) ;
#31565=ORIENTED_EDGE ( 'NONE', *, *, #18337, .F. ) ;
#31574=CARTESIAN_POINT ( 'NONE',  ( 8.118202686958138514, 201.1607312380088501, 97.29886208192144181 ) ) ;
#31575=CARTESIAN_POINT ( 'NONE',  ( 12.01549611932659367, 203.1486557965466773, 34.14886208192143613 ) ) ;
#31578=CARTESIAN_POINT ( 'NONE',  ( -6.139770520408369237, 215.5359834540460042, 42.95113791807856529 ) ) ;
#31580=CARTESIAN_POINT ( 'NONE',  ( -2.517493886309087880, 214.5937144450984135, 6.098862081921434530 ) ) ;
#31584=CARTESIAN_POINT ( 'NONE',  ( -7.984503880673422316, 204.3529502787951628, 89.34886208192143897 ) ) ;
#31585=CARTESIAN_POINT ( 'NONE',  ( 0.05014649552807626948, 215.4116977939061144, 31.25113791807856956 ) ) ;
#31587=EDGE_LOOP ( 'NONE', ( #16443, #10603, #28147, #23989, #5922, #12525 ) ) ;
#31591=CARTESIAN_POINT ( 'NONE',  ( -8.015496119326531499, 204.4483345814780364, 84.35113791807857808 ) ) ;
#31594=CARTESIAN_POINT ( 'NONE',  ( -8.000000000000008882, 206.9523078486584780, 71.49886208192144466 ) ) ;
#31599=CARTESIAN_POINT ( 'NONE',  ( 6.139770520408367460, 198.4640165459539389, 8.451137918078565292 ) ) ;
#31603=CARTESIAN_POINT ( 'NONE',  ( -7.375838497908182134, 217.2372850707499765, 81.95113791807858661 ) ) ;
#31605=CARTESIAN_POINT ( 'NONE',  ( -6.139770520408368348, 215.5359834540460042, 93.95113791807855819 ) ) ;
#31609=CARTESIAN_POINT ( 'NONE',  ( 0.05014649552828288198, 194.3824533091408000, 55.74886208192143755 ) ) ;
#31610=CARTESIAN_POINT ( 'NONE',  ( -10.01549611932659545, 210.2015048109875011, 68.64886208192143613 ) ) ;
#31612=CARTESIAN_POINT ( 'NONE',  ( 0.05014649552828288198, 194.3824533091408000, 7.748862081921433109 ) ) ;
#31614=CARTESIAN_POINT ( 'NONE',  ( -3.044812012440131443, 216.5253028482142952, 10.10113791807856565 ) ) ;
#31615=CARTESIAN_POINT ( 'NONE',  ( 3.044812012439969795, 216.5253028482143520, 75.39886208192143613 ) ) ;
#31621=CARTESIAN_POINT ( 'NONE',  ( 2.426778023690075337, 214.6231898156240447, 63.39886208192144323 ) ) ;
#31629=CARTESIAN_POINT ( 'NONE',  ( 0.05014649552807626948, 215.4116977939061144, 61.25113791807857666 ) ) ;
#31633=CARTESIAN_POINT ( 'NONE',  ( -7.984503880673422316, 204.3529502787951628, 35.34886208192144608 ) ) ;
#31634=CARTESIAN_POINT ( 'NONE',  ( 0.05014649552810505201, 217.5146222423826714, 79.25113791807856956 ) ) ;
#31636=CARTESIAN_POINT ( 'NONE',  ( -8.062137200540920645, 212.9164362838581894, 63.80113791807858092 ) ) ;
#31638=CARTESIAN_POINT ( 'NONE',  ( 8.015496119326531499, 209.5516654185219636, 10.85113791807856565 ) ) ;
#31643=CARTESIAN_POINT ( 'NONE',  ( 11.98450388067348271, 203.0532714938637753, 50.15113791807857524 ) ) ;
#31644=DIRECTION ( 'NONE',  ( 0.000000000000000000, 0.9988620819214357738, 0.04769215134144196705 ) ) ;
#31645=CARTESIAN_POINT ( 'NONE',  ( -3.135527875058821579, 197.5041725223112223, 98.90113791807857524 ) ) ;
#31646=CARTESIAN_POINT ( 'NONE',  ( 6.220909254589536808, 215.4770327129947987, 55.55113791807856671 ) ) ;
#31647=CARTESIAN_POINT ( 'NONE',  ( 9.680171189290716072, 214.0920067884432854, 24.69886208192143684 ) ) ;
#31648=CARTESIAN_POINT ( 'NONE',  ( -0.05014649552828402690, 217.5146222423826714, 36.24886208192143755 ) ) ;
#31651=CARTESIAN_POINT ( 'NONE',  ( -3.753561863808691168, 195.6020594897209435, 68.90113791807856103 ) ) ;
#31652=CARTESIAN_POINT ( 'NONE',  ( -6.500168698208129925, 202.3363017425936050, 87.20113791807858661 ) ) ;
#31653=CARTESIAN_POINT ( 'NONE',  ( 9.984503880673420539, 210.2968891136705167, 51.84886208192143897 ) ) ;
#31656=CARTESIAN_POINT ( 'NONE',  ( -7.375838497908014268, 196.7627149292498530, 53.04886208192142760 ) ) ;
#31665=CARTESIAN_POINT ( 'NONE',  ( -6.500168698208129925, 202.3363017425936050, 42.20113791807857240 ) ) ;
#31668=CARTESIAN_POINT ( 'NONE',  ( 9.984503880673420539, 210.2968891136705167, 33.84886208192143187 ) ) ;
#31673=CARTESIAN_POINT ( 'NONE',  ( 6.500168698208244500, 202.3363017425938324, 7.298862081921435596 ) ) ;
#31674=CARTESIAN_POINT ( 'NONE',  ( 8.062137200540920645, 201.0835637161417822, 47.30113791807857382 ) ) ;
#31676=CARTESIAN_POINT ( 'NONE',  ( 3.135527875058820690, 216.4958274776887492, 37.40113791807857524 ) ) ;
#31679=CARTESIAN_POINT ( 'NONE',  ( 6.500168698208244500, 202.3363017425938324, 94.29886208192142760 ) ) ;
#31683=CARTESIAN_POINT ( 'NONE',  ( -3.753561863808691168, 195.6020594897209435, 11.90113791807856813 ) ) ;
#31686=CARTESIAN_POINT ( 'NONE',  ( -3.044812012440131443, 216.5253028482142952, 67.10113791807857808 ) ) ;
#31687=CARTESIAN_POINT ( 'NONE',  ( -0.05014649552810635652, 196.4853777576173002, 29.75113791807856956 ) ) ;
#31690=CARTESIAN_POINT ( 'NONE',  ( 0.05014649552828275014, 196.4853777576173002, 13.74886208192143400 ) ) ;
#31693=CARTESIAN_POINT ( 'NONE',  ( 3.753561863808689836, 218.3979405102790565, 37.40113791807856813 ) ) ;
#31695=CARTESIAN_POINT ( 'NONE',  ( -8.062137200540822946, 201.0835637161416400, 26.19886208192143684 ) ) ;
#31699=CARTESIAN_POINT ( 'NONE',  ( 10.00000000000000711, 206.9523078486586201, 83.00113791807856956 ) ) ;
#31705=CARTESIAN_POINT ( 'NONE',  ( -2.517493886308901807, 199.4062855549015012, 11.90113791807856813 ) ) ;
#31708=CARTESIAN_POINT ( 'NONE',  ( -3.753561863808878130, 218.3979405102790281, 102.0988620819214532 ) ) ;
#31714=CARTESIAN_POINT ( 'NONE',  ( -6.139770520408224463, 198.4640165459539389, 80.04886208192139918 ) ) ;
#31716=CARTESIAN_POINT ( 'NONE',  ( 0.05014649552810505201, 217.5146222423826714, 22.25113791807856956 ) ) ;
#31722=CARTESIAN_POINT ( 'NONE',  ( 9.984503880673470277, 203.7031108863295401, 89.15113791807857524 ) ) ;
#31725=CARTESIAN_POINT ( 'NONE',  ( -0.05014649552828442242, 219.6175466908591716, 99.24886208192143044 ) ) ;
#31728=DIRECTION ( 'NONE',  ( -0.08583835255247916629, -0.09953364313786493278, -0.9913247858874408847 ) ) ;
#31735=CARTESIAN_POINT ( 'NONE',  ( 8.118202686958138514, 201.1607312380088501, 94.29886208192144181 ) ) ;
#31736=CARTESIAN_POINT ( 'NONE',  ( -0.05014649552828442242, 219.6175466908591716, 30.24886208192143755 ) ) ;
#31738=CARTESIAN_POINT ( 'NONE',  ( -3.044812012440131443, 216.5253028482142952, 49.10113791807857808 ) ) ;
#31740=CARTESIAN_POINT ( 'NONE',  ( -8.015496119326597224, 209.5516654185217362, 5.648862081921434353 ) ) ;
#31741=TOROIDAL_SURFACE ( 'NONE', #18138, 9.624472924841564136, 1.000000000000000444 ) ;
#31745=CARTESIAN_POINT ( 'NONE',  ( -0.05014649552828365914, 215.4116977939061144, 87.24886208192144466 ) ) ;
#31746=CARTESIAN_POINT ( 'NONE',  ( -2.517493886308901807, 199.4062855549015012, 26.90113791807856813 ) ) ;
#31753=CARTESIAN_POINT ( 'NONE',  ( -6.500168698208129925, 202.3363017425936050, 96.20113791807858661 ) ) ;
#31758=CARTESIAN_POINT ( 'NONE',  ( -2.517493886309087880, 214.5937144450984135, 75.09886208192142476 ) ) ;
#31762=CARTESIAN_POINT ( 'NONE',  ( 0.05014649552810506589, 217.5146222423826714, 7.251137918078566003 ) ) ;
#31767=CARTESIAN_POINT ( 'NONE',  ( 7.456977232089302632, 217.1783343296989131, 79.55113791807858092 ) ) ;
#31768=CARTESIAN_POINT ( 'NONE',  ( -10.01549611932653860, 203.7984951890123000, 99.35113791807857808 ) ) ;
#31771=CARTESIAN_POINT ( 'NONE',  ( 9.680171189290716072, 214.0920067884432854, 60.69886208192144039 ) ) ;
#31772=CARTESIAN_POINT ( 'NONE',  ( 3.135527875058981895, 197.5041725223112792, 67.59886208192143897 ) ) ;
#31774=CARTESIAN_POINT ( 'NONE',  ( 12.00000000000000711, 207.0476921513415220, 3.998862081921433997 ) ) ;
#31776=CARTESIAN_POINT ( 'NONE',  ( 8.062137200540920645, 201.0835637161417822, 14.30113791807856671 ) ) ;
#31778=CARTESIAN_POINT ( 'NONE',  ( -9.984503880673420539, 203.7031108863293980, 83.34886208192139634 ) ) ;
#31780=CARTESIAN_POINT ( 'NONE',  ( 10.00000000000000711, 206.9523078486586201, 101.0011379180785696 ) ) ;
#31783=CARTESIAN_POINT ( 'NONE',  ( 0.05014649552828262524, 198.5883022060938572, 64.74886208192143044 ) ) ;
#31789=CARTESIAN_POINT ( 'NONE',  ( 2.426778023690261410, 199.3768101843759837, 68.60113791807857808 ) ) ;
#31794=CARTESIAN_POINT ( 'NONE',  ( 6.444103211790928043, 211.7408657792734061, 48.69886208192144750 ) ) ;
#31795=CARTESIAN_POINT ( 'NONE',  ( 6.220909254589536808, 215.4770327129947702, 76.55113791807855250 ) ) ;
#31796=CARTESIAN_POINT ( 'NONE',  ( -10.00000000000000711, 207.0476921513413515, 66.50113791807856956 ) ) ;
#31798=PLANE ( 'NONE',  #15897 ) ;
#31799=CARTESIAN_POINT ( 'NONE',  ( 8.000000000000008882, 206.9523078486586485, 20.00113791807856956 ) ) ;
#31803=CARTESIAN_POINT ( 'NONE',  ( -9.680171189290831535, 214.0920067884431148, 45.80113791807856671 ) ) ;
#31805=CARTESIAN_POINT ( 'NONE',  ( 6.139770520408368348, 198.4640165459539674, 98.45113791807854398 ) ) ;
#31806=CARTESIAN_POINT ( 'NONE',  ( -0.05014649552810635652, 196.4853777576173002, 65.75113791807856956 ) ) ;
#31807=CARTESIAN_POINT ( 'NONE',  ( -11.98450388067341876, 203.0532714938636047, 29.34886208192143897 ) ) ;
#31808=CARTESIAN_POINT ( 'NONE',  ( -10.00000000000000711, 206.9523078486584495, 38.49886208192143755 ) ) ;
#31810=CARTESIAN_POINT ( 'NONE',  ( -7.456977232089304408, 196.8216656703010301, 81.05113791807856671 ) ) ;
#31811=CARTESIAN_POINT ( 'NONE',  ( -6.444103211791042618, 211.7408657792732356, 84.80113791807858092 ) ) ;
#31813=CARTESIAN_POINT ( 'NONE',  ( -8.118202686958138514, 212.8392687619910930, 47.79886208192143471 ) ) ;
#31816=CARTESIAN_POINT ( 'NONE',  ( 0.05014649552828288198, 194.3824533091408000, 58.74886208192142334 ) ) ;
#31818=CARTESIAN_POINT ( 'NONE',  ( 8.000000000000008882, 207.0476921513415220, 30.99886208192143400 ) ) ;
#31824=CARTESIAN_POINT ( 'NONE',  ( 2.426778023690261410, 199.3768101843759837, 53.60113791807856387 ) ) ;
#31826=CARTESIAN_POINT ( 'NONE',  ( 8.118202686958138514, 201.1607312380088501, 31.29886208192143826 ) ) ;
#31832=CARTESIAN_POINT ( 'NONE',  ( 2.426778023690075337, 214.6231898156240447, 18.39886208192143613 ) ) ;
#31833=CARTESIAN_POINT ( 'NONE',  ( 6.220909254589536808, 215.4770327129947702, 49.55113791807855250 ) ) ;
#31836=CARTESIAN_POINT ( 'NONE',  ( 3.044812012440130555, 197.4746971517856764, 32.60113791807857098 ) ) ;
#31838=CARTESIAN_POINT ( 'NONE',  ( -8.015496119326597224, 209.5516654185217362, 89.64886208192142192 ) ) ;
#31842=CARTESIAN_POINT ( 'NONE',  ( 7.456977232089302632, 217.1783343296989131, 19.55113791807856671 ) ) ;
#31846=CARTESIAN_POINT ( 'NONE',  ( -6.220909254589537696, 198.5229672870051161, 66.05113791807858092 ) ) ;
#31848=CARTESIAN_POINT ( 'NONE',  ( -3.044812012440131443, 216.5253028482142952, 37.10113791807857098 ) ) ;
#31851=CARTESIAN_POINT ( 'NONE',  ( -6.139770520408224463, 198.4640165459539105, 14.04886208192143471 ) ) ;
#31854=CARTESIAN_POINT ( 'NONE',  ( -3.662846001190052991, 218.4274158808045740, 52.10113791807857808 ) ) ;
#31857=CARTESIAN_POINT ( 'NONE',  ( 6.220909254589681581, 198.5229672870052582, 19.44886208192142618 ) ) ;
#31860=CARTESIAN_POINT ( 'NONE',  ( -6.139770520408369237, 215.5359834540460042, 78.95113791807858661 ) ) ;
#31864=DIRECTION ( 'NONE',  ( 0.3362851123284906207, 0.04491457122451913281, 0.9406885799869860731 ) ) ;
#31866=CARTESIAN_POINT ( 'NONE',  ( 2.517493886308900919, 214.5937144450984420, 19.40113791807856813 ) ) ;
#31868=CARTESIAN_POINT ( 'NONE',  ( -12.00000000000000711, 206.9523078486584780, 104.4988620819214304 ) ) ;
#31870=ORIENTED_EDGE ( 'NONE', *, *, #25823, .T. ) ;
#31875=CARTESIAN_POINT ( 'NONE',  ( -0.05014649552828403384, 217.5146222423826714, 84.24886208192143044 ) ) ;
#31877=CARTESIAN_POINT ( 'NONE',  ( 8.062137200540920645, 201.0835637161417822, 26.30113791807856671 ) ) ;
#31879=CARTESIAN_POINT ( 'NONE',  ( 0.05014649552828288198, 194.3824533091408000, 79.74886208192143044 ) ) ;
#31885=CARTESIAN_POINT ( 'NONE',  ( -9.984503880673473830, 210.2968891136704315, 96.65113791807857524 ) ) ;
#31888=CARTESIAN_POINT ( 'NONE',  ( -3.044812012440131443, 216.5253028482142952, 40.10113791807857098 ) ) ;
#31893=CARTESIAN_POINT ( 'NONE',  ( 3.753561863808689836, 218.3979405102790565, 10.40113791807856636 ) ) ;
#31897=CARTESIAN_POINT ( 'NONE',  ( 9.984503880673420539, 210.2968891136705736, 96.84886208192142476 ) ) ;
#31898=CARTESIAN_POINT ( 'NONE',  ( -11.98450388067341876, 203.0532714938636047, 29.34886208192143897 ) ) ;
#31900=CARTESIAN_POINT ( 'NONE',  ( -10.01549611932653860, 203.7984951890123284, 51.35113791807858519 ) ) ;
#31902=CARTESIAN_POINT ( 'NONE',  ( -7.984503880673422316, 204.3529502787951628, 11.34886208192143542 ) ) ;
#31906=CARTESIAN_POINT ( 'NONE',  ( -7.984503880673422316, 204.3529502787951628, 95.34886208192143897 ) ) ;
#31907=CARTESIAN_POINT ( 'NONE',  ( -4.903702542908602524, 213.8346818373418898, 42.95113791807857240 ) ) ;
#31912=CARTESIAN_POINT ( 'NONE',  ( 0.05014649552828275708, 196.4853777576173002, 55.74886208192143755 ) ) ;
#31915=CARTESIAN_POINT ( 'NONE',  ( 6.500168698208129925, 211.6636982574063381, 100.7011379180785866 ) ) ;
#31918=CARTESIAN_POINT ( 'NONE',  ( 8.000000000000008882, 207.0476921513415220, 69.99886208192144466 ) ) ;
#31923=CARTESIAN_POINT ( 'NONE',  ( -6.220909254589537696, 198.5229672870051445, 12.05113791807856671 ) ) ;
#31927=CARTESIAN_POINT ( 'NONE',  ( 12.00000000000000711, 206.9523078486586485, 74.00113791807856956 ) ) ;
#31928=CARTESIAN_POINT ( 'NONE',  ( 8.062137200540920645, 201.0835637161417822, 101.3011379180785809 ) ) ;
#31932=CARTESIAN_POINT ( 'NONE',  ( 8.062137200540822946, 212.9164362838583315, 3.698862081921434619 ) ) ;
#31933=CARTESIAN_POINT ( 'NONE',  ( -3.753561863808878130, 218.3979405102790281, 60.09886208192143897 ) ) ;
#31934=CARTESIAN_POINT ( 'NONE',  ( -9.984503880673420539, 203.7031108863293980, 62.34886208192143897 ) ) ;
#31935=CARTESIAN_POINT ( 'NONE',  ( -9.680171189290716072, 199.9079932115567146, 2.198862081921433731 ) ) ;
#31937=CARTESIAN_POINT ( 'NONE',  ( -3.135527875058821579, 197.5041725223112223, 20.90113791807856813 ) ) ;
#31938=CARTESIAN_POINT ( 'NONE',  ( 6.139770520408223575, 215.5359834540460611, 90.54886208192144181 ) ) ;
#31944=CARTESIAN_POINT ( 'NONE',  ( 4.903702542908435547, 213.8346818373419751, 60.54886208192144181 ) ) ;
#31951=CIRCLE ( 'NONE', #25984, 1.000000000000000888 ) ;
#31953=CARTESIAN_POINT ( 'NONE',  ( -0.05014649552807731031, 198.5883022060938572, 65.75113791807856956 ) ) ;
#31954=SURFACE_STYLE_FILL_AREA ( #6057 ) ;
#31958=CARTESIAN_POINT ( 'NONE',  ( 2.426778023690075337, 214.6231898156240447, 42.39886208192144323 ) ) ;
#31959=CARTESIAN_POINT ( 'NONE',  ( -8.118202686958039038, 201.1607312380087080, 78.20113791807857240 ) ) ;
#31960=CARTESIAN_POINT ( 'NONE',  ( -3.135527875058821579, 197.5041725223112223, 62.90113791807858235 ) ) ;
#31962=CARTESIAN_POINT ( 'NONE',  ( 8.015496119326531499, 209.5516654185219636, 22.85113791807856742 ) ) ;
#31966=CARTESIAN_POINT ( 'NONE',  ( -3.662846001190052991, 218.4274158808045740, 46.10113791807857098 ) ) ;
#31969=CARTESIAN_POINT ( 'NONE',  ( 0.05014649552810505201, 217.5146222423826714, 91.25113791807858377 ) ) ;
#31970=CARTESIAN_POINT ( 'NONE',  ( -3.135527875058821579, 197.5041725223112223, 71.90113791807857524 ) ) ;
#31972=AXIS2_PLACEMENT_3D ( 'NONE', #8623, #19182, #27013 ) ;
#31973=CARTESIAN_POINT ( 'NONE',  ( 9.680171189290716072, 214.0920067884432854, 33.69886208192142618 ) ) ;
#31974=CARTESIAN_POINT ( 'NONE',  ( 6.139770520408223575, 215.5359834540460611, 33.54886208192143471 ) ) ;
#31976=CARTESIAN_POINT ( 'NONE',  ( -7.456977232089304408, 196.8216656703010301, 75.05113791807858092 ) ) ;
#31977=CARTESIAN_POINT ( 'NONE',  ( -2.426778023690262742, 214.6231898156240163, 94.10113791807857808 ) ) ;
#31979=CARTESIAN_POINT ( 'NONE',  ( 6.220909254589681581, 198.5229672870052582, 49.44886208192144039 ) ) ;
#31984=CARTESIAN_POINT ( 'NONE',  ( 12.00000000000000711, 207.0476921513415220, 60.99886208192143044 ) ) ;
#31986=CARTESIAN_POINT ( 'NONE',  ( -7.984503880673422316, 204.3529502787951628, 32.34886208192143897 ) ) ;
#31992=CARTESIAN_POINT ( 'NONE',  ( -4.984841277089726574, 200.2242689037092305, 51.05113791807858092 ) ) ;
#31996=CARTESIAN_POINT ( 'NONE',  ( -3.135527875058982783, 216.4958274776886924, 30.09886208192143897 ) ) ;
#32002=CARTESIAN_POINT ( 'NONE',  ( -7.984503880673422316, 204.3529502787951628, 17.34886208192143187 ) ) ;
#32003=CARTESIAN_POINT ( 'NONE',  ( -6.139770520408369237, 215.5359834540460042, 51.95113791807857950 ) ) ;
#32006=CARTESIAN_POINT ( 'NONE',  ( -8.062137200540920645, 212.9164362838581894, 39.80113791807857382 ) ) ;
#32008=CIRCLE ( 'NONE', #17870, 0.9999999999999941158 ) ;
#32010=CARTESIAN_POINT ( 'NONE',  ( -8.050845014156799095, 215.4811768934071665, 104.9910338291041114 ) ) ;
#32013=CARTESIAN_POINT ( 'NONE',  ( -12.01549611932652972, 203.1486557965464499, 21.35113791807856742 ) ) ;
#32017=CARTESIAN_POINT ( 'NONE',  ( 8.118202686958039038, 212.8392687619912635, 67.70113791807858661 ) ) ;
#32018=CARTESIAN_POINT ( 'NONE',  ( 3.135527875058820690, 216.4958274776887492, 40.40113791807857524 ) ) ;
#32021=CARTESIAN_POINT ( 'NONE',  ( -3.662846001189865142, 195.5725841191952838, 1.898862081921434131 ) ) ;
#32022=CARTESIAN_POINT ( 'NONE',  ( -8.118202686958138514, 212.8392687619910930, 5.798862081921434708 ) ) ;
#32025=CARTESIAN_POINT ( 'NONE',  ( 9.680171189290831535, 199.9079932115568852, 44.30113791807857382 ) ) ;
#32028=CARTESIAN_POINT ( 'NONE',  ( 3.135527875058981895, 197.5041725223112792, 22.59886208192143542 ) ) ;
#32033=CARTESIAN_POINT ( 'NONE',  ( -6.220909254589537696, 198.5229672870051161, 78.05113791807858092 ) ) ;
#32039=CARTESIAN_POINT ( 'NONE',  ( -2.426778023690262742, 214.6231898156240163, 19.10113791807856742 ) ) ;
#32042=CARTESIAN_POINT ( 'NONE',  ( -8.062137200540822946, 201.0835637161416400, 5.198862081921435063 ) ) ;
#32050=CARTESIAN_POINT ( 'NONE',  ( 3.135527875058981895, 197.5041725223112792, 88.59886208192143897 ) ) ;
#32052=CARTESIAN_POINT ( 'NONE',  ( 6.139770520408368348, 198.4640165459539674, 23.45113791807856884 ) ) ;
#32055=CARTESIAN_POINT ( 'NONE',  ( 0.05014649552828288198, 194.3824533091408000, 76.74886208192144466 ) ) ;
#32059=CARTESIAN_POINT ( 'NONE',  ( -8.062137200540920645, 212.9164362838581894, 93.80113791807858092 ) ) ;
#32063=CARTESIAN_POINT ( 'NONE',  ( -6.220909254589537696, 198.5229672870051161, 36.05113791807857382 ) ) ;
#32067=CARTESIAN_POINT ( 'NONE',  ( 4.102348501002488490, 207.3577873115561943, -8.835681806194324750 ) ) ;
#32069=CARTESIAN_POINT ( 'NONE',  ( -12.00000000000000711, 207.0476921513413515, 24.50113791807856600 ) ) ;
#32073=CARTESIAN_POINT ( 'NONE',  ( 12.00000000000000711, 207.0476921513415220, 30.99886208192143400 ) ) ;
#32076=CARTESIAN_POINT ( 'NONE',  ( 6.220909254589536808, 215.4770327129947702, 52.55113791807858092 ) ) ;
#32078=CARTESIAN_POINT ( 'NONE',  ( -0.05014649552828365914, 215.4116977939061144, 12.24886208192143577 ) ) ;
#32081=CARTESIAN_POINT ( 'NONE',  ( -8.000000000000008882, 206.9523078486584780, 95.49886208192144466 ) ) ;
#32083=CARTESIAN_POINT ( 'NONE',  ( 6.444103211791042618, 202.2591342207267644, 41.30113791807857382 ) ) ;
#32087=CARTESIAN_POINT ( 'NONE',  ( 0.05014649552828275708, 196.4853777576173002, 61.74886208192143755 ) ) ;
#32090=CARTESIAN_POINT ( 'NONE',  ( 0.05014649552807626948, 215.4116977939061144, 97.25113791807856956 ) ) ;
#32093=CARTESIAN_POINT ( 'NONE',  ( 4.903702542908435547, 213.8346818373419751, 72.54886208192141339 ) ) ;
#32096=CARTESIAN_POINT ( 'NONE',  ( 10.01549611932653860, 210.2015048109876716, 13.85113791807856742 ) ) ;
#32101=CARTESIAN_POINT ( 'NONE',  ( 3.662846001190051659, 195.5725841191953691, 77.60113791807854966 ) ) ;
#32102=CARTESIAN_POINT ( 'NONE',  ( -6.220909254589537696, 198.5229672870051445, 99.05113791807858092 ) ) ;
#32105=CARTESIAN_POINT ( 'NONE',  ( 6.220909254589681581, 198.5229672870052582, 1.448862081921434397 ) ) ;
#32106=CARTESIAN_POINT ( 'NONE',  ( -12.00000000000000711, 206.9523078486584780, 65.49886208192144466 ) ) ;
#32107=CARTESIAN_POINT ( 'NONE',  ( 3.044812012439969795, 216.5253028482143520, 63.39886208192144323 ) ) ;
#32108=CARTESIAN_POINT ( 'NONE',  ( 3.662846001190051659, 195.5725841191953691, 101.6011379180785781 ) ) ;
#32110=CARTESIAN_POINT ( 'NONE',  ( -10.01549611932653860, 203.7984951890123284, 27.35113791807856742 ) ) ;
#32111=CARTESIAN_POINT ( 'NONE',  ( 8.118202686958138514, 201.1607312380088501, 91.29886208192144181 ) ) ;
#32113=CARTESIAN_POINT ( 'NONE',  ( 10.20891672561132424, 208.8253170565643302, -1.573594014082846382 ) ) ;
#32116=CARTESIAN_POINT ( 'NONE',  ( 8.015496119326595448, 204.4483345814782638, 73.14886208192142192 ) ) ;
#32122=CARTESIAN_POINT ( 'NONE',  ( 8.000000000000008882, 206.9523078486586485, 65.00113791807856956 ) ) ;
#32128=CARTESIAN_POINT ( 'NONE',  ( -4.903702542908436435, 200.1653181626580249, 44.04886208192144181 ) ) ;
#32129=CARTESIAN_POINT ( 'NONE',  ( 6.139770520408368348, 198.4640165459539674, 86.45113791807854398 ) ) ;
#32130=CARTESIAN_POINT ( 'NONE',  ( 0.05014649552810505201, 217.5146222423826714, 67.25113791807856956 ) ) ;
#32132=CARTESIAN_POINT ( 'NONE',  ( 4.984841277089725686, 213.7757310962907411, 25.55113791807857027 ) ) ;
#32136=CARTESIAN_POINT ( 'NONE',  ( -3.662846001190052991, 218.4274158808045740, 52.10113791807857808 ) ) ;
#32137=DIRECTION ( 'NONE',  ( -0.9891821073486148919, -0.1466927349985451545, 0.000000000000000000 ) ) ;
#32138=CARTESIAN_POINT ( 'NONE',  ( 10.01549611932653860, 210.2015048109876716, 97.85113791807857808 ) ) ;
#32139=CARTESIAN_POINT ( 'NONE',  ( 3.135527875058820690, 216.4958274776887492, 70.40113791807857524 ) ) ;
#32140=CARTESIAN_POINT ( 'NONE',  ( -0.05014649552828442242, 219.6175466908591716, 30.24886208192143755 ) ) ;
#32141=CARTESIAN_POINT ( 'NONE',  ( -10.00000000000000711, 206.9523078486584495, 35.49886208192143044 ) ) ;
#32143=CARTESIAN_POINT ( 'NONE',  ( 3.753561863808689836, 218.3979405102790565, 76.40113791807856103 ) ) ;
#32144=CARTESIAN_POINT ( 'NONE',  ( 7.984503880673485376, 204.3529502787953902, 95.15113791807856103 ) ) ;
#32145=CARTESIAN_POINT ( 'NONE',  ( -6.139770520408224463, 198.4640165459539389, 62.04886208192142050 ) ) ;
#32148=CARTESIAN_POINT ( 'NONE',  ( -3.753561863808878130, 218.3979405102790281, 57.09886208192143897 ) ) ;
#32152=CARTESIAN_POINT ( 'NONE',  ( 6.500168698208244500, 202.3363017425938324, 43.29886208192144181 ) ) ;
#32157=CARTESIAN_POINT ( 'NONE',  ( 2.517493886308900919, 214.5937144450984420, 52.40113791807858235 ) ) ;
#32159=CARTESIAN_POINT ( 'NONE',  ( 3.135527875058981895, 197.5041725223112792, 37.59886208192143187 ) ) ;
#32163=SURFACE_SIDE_STYLE ('',( #17168 ) ) ;
#32166=CARTESIAN_POINT ( 'NONE',  ( 0.05014649552828262524, 198.5883022060938572, 19.74886208192143400 ) ) ;
#32167=CARTESIAN_POINT ( 'NONE',  ( 3.135527875058820690, 216.4958274776887492, 55.40113791807857524 ) ) ;
#32169=CARTESIAN_POINT ( 'NONE',  ( -3.135527875058821579, 197.5041725223112223, 41.90113791807856813 ) ) ;
#32173=CARTESIAN_POINT ( 'NONE',  ( -6.444103211790928043, 202.2591342207265939, 101.1988620819214475 ) ) ;
#32177=CARTESIAN_POINT ( 'NONE',  ( 3.662846001190051659, 195.5725841191953691, 17.60113791807856742 ) ) ;
#32181=CARTESIAN_POINT ( 'NONE',  ( 3.044812012440130555, 197.4746971517856764, 68.60113791807857808 ) ) ;
#32182=CARTESIAN_POINT ( 'NONE',  ( -3.135527875058821579, 197.5041725223112223, 41.90113791807856813 ) ) ;
#32185=CARTESIAN_POINT ( 'NONE',  ( -0.05014649552807705357, 194.3824533091408000, 101.7511379180785696 ) ) ;
#32186=CARTESIAN_POINT ( 'NONE',  ( 0.05014649552828275014, 196.4853777576173002, 4.748862081921433997 ) ) ;
#32190=CARTESIAN_POINT ( 'NONE',  ( -3.662846001190052991, 218.4274158808045740, 49.10113791807857808 ) ) ;
#32191=CARTESIAN_POINT ( 'NONE',  ( 2.517493886308900919, 214.5937144450984420, 70.40113791807856103 ) ) ;
#32192=CARTESIAN_POINT ( 'NONE',  ( -0.05014649552828403384, 217.5146222423826714, 33.24886208192142334 ) ) ;
#32195=CARTESIAN_POINT ( 'NONE',  ( 8.118202686958039038, 212.8392687619912635, 79.70113791807857240 ) ) ;
#32200=CARTESIAN_POINT ( 'NONE',  ( 2.426778023690261410, 199.3768101843759837, 23.60113791807857098 ) ) ;
#32203=CARTESIAN_POINT ( 'NONE',  ( 0.05014649552828275708, 196.4853777576173002, 4.748862081921434886 ) ) ;
#32210=CARTESIAN_POINT ( 'NONE',  ( 8.062137200540822946, 212.9164362838583315, 93.69886208192143329 ) ) ;
#32212=CARTESIAN_POINT ( 'NONE',  ( 6.220909254589536808, 215.4770327129947702, 25.55113791807856671 ) ) ;
#32215=CARTESIAN_POINT ( 'NONE',  ( 11.98450388067341876, 210.9467285061363953, 78.84886208192143897 ) ) ;
#32218=LINE ( 'NONE', #16376, #9892 ) ;
#32219=CARTESIAN_POINT ( 'NONE',  ( -6.220909254589537696, 198.5229672870051161, 93.05113791807853829 ) ) ;
#32222=CARTESIAN_POINT ( 'NONE',  ( 6.139770520408368348, 198.4640165459539674, 41.45113791807857240 ) ) ;
#32229=CARTESIAN_POINT ( 'NONE',  ( -7.375838497908182134, 217.2372850707499765, 21.95113791807856884 ) ) ;
#32232=CARTESIAN_POINT ( 'NONE',  ( 9.680171189290716072, 214.0920067884432854, 30.69886208192143684 ) ) ;
#32234=CARTESIAN_POINT ( 'NONE',  ( 6.139770520408368348, 198.4640165459539674, 47.45113791807857950 ) ) ;
#32237=EDGE_CURVE ( 'NONE', #14046, #20137, #26276, .T. ) ;
#32238=CARTESIAN_POINT ( 'NONE',  ( -4.903702542908436435, 200.1653181626580249, 17.04886208192143471 ) ) ;
#32242=CARTESIAN_POINT ( 'NONE',  ( 4.903702542908435547, 213.8346818373419751, 96.54886208192142760 ) ) ;
#32244=CARTESIAN_POINT ( 'NONE',  ( 4.984841277089725686, 213.7757310962907411, 43.55113791807857382 ) ) ;
#32249=CARTESIAN_POINT ( 'NONE',  ( -3.135527875058982783, 216.4958274776886924, 60.09886208192143897 ) ) ;
#32252=CARTESIAN_POINT ( 'NONE',  ( -8.015496119326531499, 204.4483345814780364, 93.35113791807857808 ) ) ;
#32257=CARTESIAN_POINT ( 'NONE',  ( 0.05014649552828262524, 198.5883022060938572, 73.74886208192144466 ) ) ;
#32260=AXIS2_PLACEMENT_3D ( 'NONE', #28062, #20404, #4724 ) ;
#32262=CARTESIAN_POINT ( 'NONE',  ( 6.139770520408367460, 198.4640165459539389, 11.45113791807856707 ) ) ;
#32266=CARTESIAN_POINT ( 'NONE',  ( -7.456977232089304408, 196.8216656703010301, 81.05113791807856671 ) ) ;
#32269=CARTESIAN_POINT ( 'NONE',  ( -6.220909254589537696, 198.5229672870051445, 96.05113791807858092 ) ) ;
#32272=CARTESIAN_POINT ( 'NONE',  ( -10.01549611932659722, 210.2015048109875011, 5.648862081921435241 ) ) ;
#32273=CARTESIAN_POINT ( 'NONE',  ( 7.375838497908012492, 217.2372850707501186, 57.54886208192142760 ) ) ;
#32275=CARTESIAN_POINT ( 'NONE',  ( 8.062137200540822946, 212.9164362838583315, 75.69886208192143329 ) ) ;
#32276=CARTESIAN_POINT ( 'NONE',  ( 9.736236675708031640, 199.9851607334238963, 7.298862081921434708 ) ) ;
#32278=CARTESIAN_POINT ( 'NONE',  ( 10.00000000000000711, 206.9523078486586201, 26.00113791807856956 ) ) ;
#32281=CARTESIAN_POINT ( 'NONE',  ( -9.984503880673420539, 203.7031108863293980, 92.34886208192141055 ) ) ;
#32287=CARTESIAN_POINT ( 'NONE',  ( 6.500168698208244500, 202.3363017425938324, 73.29886208192142760 ) ) ;
#32294=DIRECTION ( 'NONE',  ( -0.8289387912553660698, 0.000000000000000000, 0.5593393248754217062 ) ) ;
#32296=CARTESIAN_POINT ( 'NONE',  ( -0.05014649552807731031, 198.5883022060938572, 71.75113791807856956 ) ) ;
#32300=CARTESIAN_POINT ( 'NONE',  ( 2.517493886309087436, 199.4062855549015865, 43.59886208192144608 ) ) ;
#32301=CARTESIAN_POINT ( 'NONE',  ( 3.135527875058820690, 216.4958274776887492, 88.40113791807857524 ) ) ;
#32302=CARTESIAN_POINT ( 'NONE',  ( 8.062137200540920645, 201.0835637161417822, 62.30113791807858092 ) ) ;
#32308=CARTESIAN_POINT ( 'NONE',  ( 7.375838497908181246, 196.7627149292499666, 50.45113791807855819 ) ) ;
#32310=CARTESIAN_POINT ( 'NONE',  ( -10.00000000000000711, 207.0476921513413515, 90.50113791807858377 ) ) ;
#32311=CARTESIAN_POINT ( 'NONE',  ( -9.984503880673475606, 210.2968891136704315, 69.65113791807856103 ) ) ;
#32312=CARTESIAN_POINT ( 'NONE',  ( -12.00000000000000711, 206.9523078486584780, 35.49886208192143044 ) ) ;
#32313=CARTESIAN_POINT ( 'NONE',  ( -3.135527875058982783, 216.4958274776886924, 42.09886208192143897 ) ) ;
#32315=CARTESIAN_POINT ( 'NONE',  ( 9.680171189290831535, 199.9079932115568852, 77.30113791807858092 ) ) ;
#32316=CARTESIAN_POINT ( 'NONE',  ( -4.984841277089726574, 200.2242689037092305, 96.05113791807858092 ) ) ;
#32317=CARTESIAN_POINT ( 'NONE',  ( -3.044812012439970683, 197.4746971517856196, 58.89886208192143613 ) ) ;
#32319=CARTESIAN_POINT ( 'NONE',  ( -12.00000000000000711, 206.9523078486584780, 65.49886208192144466 ) ) ;
#32323=CARTESIAN_POINT ( 'NONE',  ( -4.903702542908436435, 200.1653181626580249, 44.04886208192144181 ) ) ;
#32324=EDGE_LOOP ( 'NONE', ( #21102, #29353, #10109, #26496 ) ) ;
#32328=CARTESIAN_POINT ( 'NONE',  ( -7.984503880673488041, 209.6470497212046098, 48.65113791807857524 ) ) ;
#32330=CARTESIAN_POINT ( 'NONE',  ( 6.220909254589681581, 198.5229672870052582, 34.44886208192143329 ) ) ;
#32338=CARTESIAN_POINT ( 'NONE',  ( 4.903702542908435547, 213.8346818373419751, 15.54886208192143826 ) ) ;
#32339=CARTESIAN_POINT ( 'NONE',  ( 3.135527875058820690, 216.4958274776887492, 58.40113791807857524 ) ) ;
#32340=CARTESIAN_POINT ( 'NONE',  ( -10.00000000000000711, 207.0476921513413515, 36.50113791807857666 ) ) ;
#32344=CARTESIAN_POINT ( 'NONE',  ( 6.500168698208244500, 202.3363017425938324, 100.2988620819214276 ) ) ;
#32348=CARTESIAN_POINT ( 'NONE',  ( 9.736236675707914401, 214.0148392665762458, 16.70113791807856529 ) ) ;
#32350=CARTESIAN_POINT ( 'NONE',  ( -0.05014649552810635652, 196.4853777576173002, 65.75113791807856956 ) ) ;
#32351=CARTESIAN_POINT ( 'NONE',  ( 3.135527875058820690, 216.4958274776887492, 37.40113791807857524 ) ) ;
#32354=CARTESIAN_POINT ( 'NONE',  ( -7.375838497908014268, 196.7627149292498530, 8.048862081921434708 ) ) ;
#32355=CARTESIAN_POINT ( 'NONE',  ( 10.00000000000000711, 207.0476921513415220, 6.998862081921434886 ) ) ;
#32358=CARTESIAN_POINT ( 'NONE',  ( 12.01549611932652972, 210.8513442034534933, 52.85113791807857098 ) ) ;
#32359=CARTESIAN_POINT ( 'NONE',  ( 2.426778023690261410, 199.3768101843759837, 71.60113791807857808 ) ) ;
#32361=CARTESIAN_POINT ( 'NONE',  ( -3.044812012439970683, 197.4746971517856196, 31.89886208192143613 ) ) ;
#32363=CARTESIAN_POINT ( 'NONE',  ( -6.139770520408369237, 215.5359834540460042, 75.95113791807857240 ) ) ;
#32369=CARTESIAN_POINT ( 'NONE',  ( -6.500168698208129925, 202.3363017425936050, 18.20113791807856529 ) ) ;
#32371=CARTESIAN_POINT ( 'NONE',  ( -9.984503880673420539, 203.7031108863293980, 8.348862081921435419 ) ) ;
#32375=CARTESIAN_POINT ( 'NONE',  ( 4.984841277089725686, 213.7757310962907411, 49.55113791807858092 ) ) ;
#32379=CARTESIAN_POINT ( 'NONE',  ( 10.01549611932659545, 203.7984951890123853, 94.14886208192143613 ) ) ;
#32381=CARTESIAN_POINT ( 'NONE',  ( 8.118202686958039038, 212.8392687619912635, 28.70113791807856884 ) ) ;
#32383=CARTESIAN_POINT ( 'NONE',  ( -12.00000000000000711, 206.9523078486584780, 83.49886208192144466 ) ) ;
#32387=CARTESIAN_POINT ( 'NONE',  ( 10.01549611932653860, 210.2015048109876716, 97.85113791807857808 ) ) ;
#32390=CARTESIAN_POINT ( 'NONE',  ( -0.05014649552810635652, 196.4853777576173002, 32.75113791807856956 ) ) ;
#32396=CARTESIAN_POINT ( 'NONE',  ( -7.456977232089304408, 196.8216656703010301, 18.05113791807856316 ) ) ;
#32397=CARTESIAN_POINT ( 'NONE',  ( -10.79277039317867271, 207.6632728202857550, 102.8962892815882668 ) ) ;
#32400=CARTESIAN_POINT ( 'NONE',  ( 12.01549611932659367, 203.1486557965466773, 43.14886208192143613 ) ) ;
#32401=CARTESIAN_POINT ( 'NONE',  ( 8.062137200540920645, 201.0835637161417822, 5.301137918078566713 ) ) ;
#32402=CARTESIAN_POINT ( 'NONE',  ( 10.00000000000000711, 206.9523078486586201, 56.00113791807856956 ) ) ;
#32403=CARTESIAN_POINT ( 'NONE',  ( -8.015496119326597224, 209.5516654185217362, 11.64886208192143613 ) ) ;
#32407=CARTESIAN_POINT ( 'NONE',  ( -8.015496119326597224, 209.5516654185217362, 95.64886208192143613 ) ) ;
#32409=CARTESIAN_POINT ( 'NONE',  ( -4.903702542908602524, 213.8346818373418898, 36.95113791807857950 ) ) ;
#32413=CARTESIAN_POINT ( 'NONE',  ( -0.3755270751584372513, 206.7692714347155629, 108.3323677711371573 ) ) ;
#32416=CARTESIAN_POINT ( 'NONE',  ( 3.135527875058981895, 197.5041725223112792, 64.59886208192143897 ) ) ;
#32418=DIRECTION ( 'NONE',  ( 5.170793409489829447E-18, -0.9988620819214357738, 0.04769215134144141888 ) ) ;
#32419=CARTESIAN_POINT ( 'NONE',  ( 6.500168698208129925, 211.6636982574063381, 94.70113791807858661 ) ) ;
#32422=CARTESIAN_POINT ( 'NONE',  ( -0.05014649552828365914, 215.4116977939061144, 78.24886208192144466 ) ) ;
#32427=CARTESIAN_POINT ( 'NONE',  ( -9.984503880673475606, 210.2968891136704315, 21.65113791807856103 ) ) ;
#32431=CARTESIAN_POINT ( 'NONE',  ( 7.375838497908181246, 196.7627149292499666, 86.45113791807858661 ) ) ;
#32436=ORIENTED_EDGE ( 'NONE', *, *, #30545, .T. ) ;
#32437=CARTESIAN_POINT ( 'NONE',  ( -11.98450388067341876, 203.0532714938636047, 71.34886208192142476 ) ) ;
#32438=CARTESIAN_POINT ( 'NONE',  ( -8.062137200540822946, 201.0835637161416400, 77.19886208192143329 ) ) ;
#32439=CARTESIAN_POINT ( 'NONE',  ( 12.00000000000000711, 207.0476921513415220, 9.998862081921435774 ) ) ;
#32441=CARTESIAN_POINT ( 'NONE',  ( 9.984503880673470277, 203.7031108863295401, 23.15113791807856813 ) ) ;
#32442=CARTESIAN_POINT ( 'NONE',  ( -3.044812012439970683, 197.4746971517856196, 91.89886208192143613 ) ) ;
#32448=CARTESIAN_POINT ( 'NONE',  ( 4.903702542908435547, 213.8346818373419751, 75.54886208192142760 ) ) ;
#32449=ORIENTED_EDGE ( 'NONE', *, *, #367, .T. ) ;
#32455=CARTESIAN_POINT ( 'NONE',  ( 8.015496119326531499, 209.5516654185219636, 67.85113791807857808 ) ) ;
#32461=CARTESIAN_POINT ( 'NONE',  ( -0.05014649552828365914, 215.4116977939061144, 48.24886208192144466 ) ) ;
#32463=CARTESIAN_POINT ( 'NONE',  ( 10.00000000000000711, 206.9523078486586201, 77.00113791807858377 ) ) ;
#32469=CARTESIAN_POINT ( 'NONE',  ( 9.736236675707914401, 214.0148392665762458, 55.70113791807856529 ) ) ;
#32472=CARTESIAN_POINT ( 'NONE',  ( 0.05014649552810505201, 217.5146222423826714, 100.2511379180785838 ) ) ;
#32473=CARTESIAN_POINT ( 'NONE',  ( -6.139770520408368348, 215.5359834540460042, 63.95113791807857950 ) ) ;
#32474=CARTESIAN_POINT ( 'NONE',  ( 3.753561863808876797, 195.6020594897209719, 31.59886208192143187 ) ) ;
#32475=CARTESIAN_POINT ( 'NONE',  ( -10.01549611932659545, 210.2015048109875011, 50.64886208192143613 ) ) ;
#32477=CARTESIAN_POINT ( 'NONE',  ( -7.375838497908182134, 217.2372850707499765, 72.95113791807857240 ) ) ;
#32479=CARTESIAN_POINT ( 'NONE',  ( -7.984503880673488041, 209.6470497212046098, 99.65113791807858945 ) ) ;
#32480=CARTESIAN_POINT ( 'NONE',  ( -8.118202686958138514, 212.8392687619910930, 56.79886208192143471 ) ) ;
#32484=CARTESIAN_POINT ( 'NONE',  ( -9.680171189290716072, 199.9079932115567146, 65.19886208192143329 ) ) ;
#32487=CARTESIAN_POINT ( 'NONE',  ( 6.444103211790928043, 211.7408657792734061, 39.69886208192144750 ) ) ;
#32493=CARTESIAN_POINT ( 'NONE',  ( -2.426778023690262742, 214.6231898156240163, 58.10113791807857808 ) ) ;
#32495=CARTESIAN_POINT ( 'NONE',  ( 6.220909254589681581, 198.5229672870052582, 46.44886208192141908 ) ) ;
#32502=CARTESIAN_POINT ( 'NONE',  ( 0.05014649552828262524, 198.5883022060938572, 16.74886208192143755 ) ) ;
#32503=CARTESIAN_POINT ( 'NONE',  ( 3.135527875058820690, 216.4958274776887492, 61.40113791807857524 ) ) ;
#32505=CARTESIAN_POINT ( 'NONE',  ( 3.135527875058820690, 216.4958274776887492, 46.40113791807857524 ) ) ;
#32508=( GEOMETRIC_REPRESENTATION_CONTEXT ( 3 ) GLOBAL_UNCERTAINTY_ASSIGNED_CONTEXT ( ( #18520 ) ) GLOBAL_UNIT_ASSIGNED_CONTEXT ( ( #23960, #16449, #31472 ) ) REPRESENTATION_CONTEXT ( 'NONE', 'WORKASPACE' ) );
#32509=CARTESIAN_POINT ( 'NONE',  ( -0.05014649552810635652, 196.4853777576173002, 14.75113791807856245 ) ) ;
#32510=CARTESIAN_POINT ( 'NONE',  ( 8.000000000000008882, 206.9523078486586485, -0.9988620819214343305 ) ) ;
#32513=CARTESIAN_POINT ( 'NONE',  ( 0.05014649552807549926, 219.6175466908591716, 22.25113791807856956 ) ) ;
#32515=CARTESIAN_POINT ( 'NONE',  ( 8.062137200540920645, 201.0835637161417822, 77.30113791807858092 ) ) ;
#32516=CARTESIAN_POINT ( 'NONE',  ( 6.139770520408367460, 198.4640165459539389, 38.45113791807856529 ) ) ;
#32519=CARTESIAN_POINT ( 'NONE',  ( -7.375838497908014268, 196.7627149292498530, 5.048862081921433820 ) ) ;
#32520=CARTESIAN_POINT ( 'NONE',  ( 10.00000000000000711, 207.0476921513415220, 21.99886208192143755 ) ) ;
#32523=CARTESIAN_POINT ( 'NONE',  ( -3.753561863808691168, 195.6020594897209435, 47.90113791807857524 ) ) ;
#32524=CARTESIAN_POINT ( 'NONE',  ( 2.517493886308900919, 214.5937144450984420, 73.40113791807856103 ) ) ;
#32525=CARTESIAN_POINT ( 'NONE',  ( 9.984503880673420539, 210.2968891136705167, 30.84886208192142831 ) ) ;
#32527=CARTESIAN_POINT ( 'NONE',  ( 10.01549611932653860, 210.2015048109876716, 91.85113791807853545 ) ) ;
#32530=AXIS2_PLACEMENT_3D ( 'NONE', #9160, #6604, #16987 ) ;
#32534=CARTESIAN_POINT ( 'NONE',  ( -6.500168698208129925, 202.3363017425936050, 24.20113791807856529 ) ) ;
#32536=CARTESIAN_POINT ( 'NONE',  ( 10.01549611932659545, 203.7984951890123853, 7.148862081921433465 ) ) ;
#32540=CARTESIAN_POINT ( 'NONE',  ( 6.500168698208129925, 211.6636982574063381, 52.70113791807857240 ) ) ;
#32544=CARTESIAN_POINT ( 'NONE',  ( -6.220909254589682469, 215.4770327129946850, 86.94886208192141908 ) ) ;
#32546=CARTESIAN_POINT ( 'NONE',  ( 0.05014649552810505201, 217.5146222423826714, 28.25113791807855890 ) ) ;
#32548=CARTESIAN_POINT ( 'NONE',  ( -0.05014649552828442242, 219.6175466908591716, 78.24886208192144466 ) ) ;
#32553=CARTESIAN_POINT ( 'NONE',  ( -10.00000000000000711, 207.0476921513413515, 90.50113791807858377 ) ) ;
#32557=CARTESIAN_POINT ( 'NONE',  ( -6.220909254589537696, 198.5229672870051161, 39.05113791807856671 ) ) ;
#32566=CARTESIAN_POINT ( 'NONE',  ( -9.736236675707914401, 199.9851607334237542, 15.20113791807857062 ) ) ;
#32571=CARTESIAN_POINT ( 'NONE',  ( -3.753561863808878130, 218.3979405102790281, 39.09886208192143187 ) ) ;
#32572=CARTESIAN_POINT ( 'NONE',  ( 3.044812012440130555, 197.4746971517856764, -0.3988620819214342972 ) ) ;
#32573=CARTESIAN_POINT ( 'NONE',  ( 3.044812012440130555, 197.4746971517856764, 59.60113791807857808 ) ) ;
#32574=CARTESIAN_POINT ( 'NONE',  ( 2.517493886309087436, 199.4062855549015865, 10.59886208192143542 ) ) ;
#32578=CARTESIAN_POINT ( 'NONE',  ( 8.000000000000008882, 207.0476921513415220, 96.99886208192143044 ) ) ;
#32581=CARTESIAN_POINT ( 'NONE',  ( 8.000000000000008882, 206.9523078486586485, 38.00113791807857666 ) ) ;
#32589=CARTESIAN_POINT ( 'NONE',  ( 10.00000000000000711, 207.0476921513415220, 63.99886208192143044 ) ) ;
#32592=CARTESIAN_POINT ( 'NONE',  ( -0.05014649552810635652, 196.4853777576173002, 5.751137918078563338 ) ) ;
#32596=CARTESIAN_POINT ( 'NONE',  ( -6.444103211790928043, 202.2591342207265939, 83.19886208192144750 ) ) ;
#32601=CARTESIAN_POINT ( 'NONE',  ( 8.118202686958039038, 212.8392687619912635, 16.70113791807856529 ) ) ;
#32605=CARTESIAN_POINT ( 'NONE',  ( -7.375838497908182134, 217.2372850707499765, 87.95113791807857240 ) ) ;
#32610=CARTESIAN_POINT ( 'NONE',  ( -12.00000000000000711, 206.9523078486584780, 71.49886208192144466 ) ) ;
#32611=CARTESIAN_POINT ( 'NONE',  ( 0.05014649552828275014, 196.4853777576173002, 76.74886208192143044 ) ) ;
#32612=CARTESIAN_POINT ( 'NONE',  ( -7.456977232089471386, 217.1783343296987709, 11.94886208192143506 ) ) ;
#32614=CARTESIAN_POINT ( 'NONE',  ( -6.139770520408369237, 215.5359834540460042, 24.95113791807855819 ) ) ;
#32616=CARTESIAN_POINT ( 'NONE',  ( -0.05014649552828403384, 217.5146222423826714, 84.24886208192143044 ) ) ;
#32621=CARTESIAN_POINT ( 'NONE',  ( 8.000000000000008882, 207.0476921513415220, 69.99886208192144466 ) ) ;
#32630=CARTESIAN_POINT ( 'NONE',  ( -4.903702542908602524, 213.8346818373418898, 75.95113791807857240 ) ) ;
#32634=CARTESIAN_POINT ( 'NONE',  ( -4.903702542908436435, 200.1653181626580249, 53.04886208192144181 ) ) ;
#32641=CARTESIAN_POINT ( 'NONE',  ( -9.736236675707914401, 199.9851607334237542, 57.20113791807856529 ) ) ;
#32643=CARTESIAN_POINT ( 'NONE',  ( -12.00000000000000711, 207.0476921513413515, 3.501137918078566003 ) ) ;
#32644=CARTESIAN_POINT ( 'NONE',  ( -8.118202686958039038, 201.1607312380087080, 75.20113791807857240 ) ) ;
#32646=CARTESIAN_POINT ( 'NONE',  ( -12.00000000000000711, 206.9523078486584780, 41.49886208192143044 ) ) ;
#32647=CARTESIAN_POINT ( 'NONE',  ( -10.01549611932659545, 210.2015048109875011, 47.64886208192142902 ) ) ;
#32649=CARTESIAN_POINT ( 'NONE',  ( -7.375838497908182134, 217.2372850707499765, 90.95113791807855819 ) ) ;
#32650=CARTESIAN_POINT ( 'NONE',  ( -8.000000000000008882, 207.0476921513413515, 99.50113791807856956 ) ) ;
#32651=CARTESIAN_POINT ( 'NONE',  ( 0.05014649552828275708, 196.4853777576173002, 61.74886208192143755 ) ) ;
#32653=CARTESIAN_POINT ( 'NONE',  ( -11.98450388067341876, 203.0532714938636047, 68.34886208192142476 ) ) ;
#32656=CARTESIAN_POINT ( 'NONE',  ( -4.984841277089891776, 213.7757310962905990, 38.94886208192144039 ) ) ;
#32662=CARTESIAN_POINT ( 'NONE',  ( -6.500168698208129925, 202.3363017425936050, 60.20113791807857240 ) ) ;
#32664=CARTESIAN_POINT ( 'NONE',  ( -8.062137200540822946, 201.0835637161416400, 41.19886208192144039 ) ) ;
#32667=AXIS2_PLACEMENT_3D ( 'NONE', #16336, #26730, #6108 ) ;
#32670=CARTESIAN_POINT ( 'NONE',  ( -8.000000000000008882, 206.9523078486584780, 23.49886208192144110 ) ) ;
#32671=CARTESIAN_POINT ( 'NONE',  ( 3.135527875058820690, 216.4958274776887492, 64.40113791807857524 ) ) ;
#32672=CARTESIAN_POINT ( 'NONE',  ( -0.05014649552810635652, 196.4853777576173002, 47.75113791807855534 ) ) ;
#32674=CARTESIAN_POINT ( 'NONE',  ( 8.118202686958039038, 212.8392687619912635, 13.70113791807856707 ) ) ;
#32675=CARTESIAN_POINT ( 'NONE',  ( -6.444103211790928043, 202.2591342207265939, 98.19886208192144750 ) ) ;
#32678=CARTESIAN_POINT ( 'NONE',  ( -3.753561863808691168, 195.6020594897209435, 29.90113791807857169 ) ) ;
#32680=CARTESIAN_POINT ( 'NONE',  ( -0.05014649552810635652, 196.4853777576173002, 71.75113791807858377 ) ) ;
#32681=CARTESIAN_POINT ( 'NONE',  ( 6.139770520408367460, 198.4640165459539389, 47.45113791807856529 ) ) ;
#32683=CARTESIAN_POINT ( 'NONE',  ( -9.736236675708031640, 214.0148392665760753, 17.79886208192143471 ) ) ;
#32684=CARTESIAN_POINT ( 'NONE',  ( -10.01549611932659545, 210.2015048109875011, 14.64886208192143435 ) ) ;
#32688=CARTESIAN_POINT ( 'NONE',  ( 3.662846001190051659, 195.5725841191953691, 59.60113791807857808 ) ) ;
#32689=CARTESIAN_POINT ( 'NONE',  ( -8.015496119326531499, 204.4483345814780364, 69.35113791807857808 ) ) ;
#32691=CARTESIAN_POINT ( 'NONE',  ( -3.044812012439970683, 197.4746971517856196, 28.89886208192143613 ) ) ;
#32695=CARTESIAN_POINT ( 'NONE',  ( 8.062137200540920645, 201.0835637161417822, 86.30113791807856671 ) ) ;
#32703=CARTESIAN_POINT ( 'NONE',  ( 2.426778023690261410, 199.3768101843759837, 29.60113791807856742 ) ) ;
#32705=CARTESIAN_POINT ( 'NONE',  ( -10.00000000000000711, 206.9523078486584495, 11.49886208192143577 ) ) ;
#32708=CARTESIAN_POINT ( 'NONE',  ( 8.000000000000008882, 206.9523078486586485, 53.00113791807857666 ) ) ;
#32713=CARTESIAN_POINT ( 'NONE',  ( -8.062137200540822946, 201.0835637161416400, 98.19886208192143329 ) ) ;
#32715=CARTESIAN_POINT ( 'NONE',  ( 9.984503880673470277, 203.7031108863295401, 35.15113791807856813 ) ) ;
#32717=CARTESIAN_POINT ( 'NONE',  ( -8.118202686958039038, 201.1607312380087080, 18.20113791807856884 ) ) ;
#32722=CARTESIAN_POINT ( 'NONE',  ( -3.135527875058821579, 197.5041725223112223, 101.9011379180785752 ) ) ;
#32725=CARTESIAN_POINT ( 'NONE',  ( -8.118202686958039038, 201.1607312380087080, 42.20113791807857240 ) ) ;
#32732=CARTESIAN_POINT ( 'NONE',  ( 12.00000000000000711, 206.9523078486586485, 29.00113791807856956 ) ) ;
#32737=CARTESIAN_POINT ( 'NONE',  ( 3.753561863808876797, 195.6020594897209719, 40.59886208192143187 ) ) ;
#32738=CARTESIAN_POINT ( 'NONE',  ( -8.062137200540920645, 212.9164362838581894, 3.801137918078565825 ) ) ;
#32739=CARTESIAN_POINT ( 'NONE',  ( 6.220909254589536808, 215.4770327129947702, 61.55113791807858092 ) ) ;
#32740=CARTESIAN_POINT ( 'NONE',  ( -7.984503880673422316, 204.3529502787951628, 26.34886208192143897 ) ) ;
#32744=CARTESIAN_POINT ( 'NONE',  ( 4.903702542908601636, 200.1653181626581102, 8.451137918078563516 ) ) ;
#32746=CARTESIAN_POINT ( 'NONE',  ( 3.753561863808876797, 195.6020594897209719, 85.59886208192143897 ) ) ;
#32752=CARTESIAN_POINT ( 'NONE',  ( -3.044812012439970683, 197.4746971517856196, 61.89886208192143613 ) ) ;
#32755=CARTESIAN_POINT ( 'NONE',  ( -10.01549611932653860, 203.7984951890123284, 0.3511379180785655363 ) ) ;
#32760=CARTESIAN_POINT ( 'NONE',  ( -4.903702542908436435, 200.1653181626580249, 86.04886208192145602 ) ) ;
#32763=CARTESIAN_POINT ( 'NONE',  ( 9.680171189290716072, 214.0920067884432854, 84.69886208192144750 ) ) ;
#32765=CARTESIAN_POINT ( 'NONE',  ( 0.05014649552810506589, 217.5146222423826714, 25.25113791807856600 ) ) ;
#32770=CARTESIAN_POINT ( 'NONE',  ( 12.01549611932652972, 210.8513442034534933, 82.85113791807857808 ) ) ;
#32774=CARTESIAN_POINT ( 'NONE',  ( 3.753561863808876797, 195.6020594897209719, 67.59886208192143897 ) ) ;
#32775=CARTESIAN_POINT ( 'NONE',  ( 8.062137200540822946, 212.9164362838583315, 72.69886208192143329 ) ) ;
#32776=CARTESIAN_POINT ( 'NONE',  ( -3.753561863808878130, 218.3979405102790281, 18.09886208192143187 ) ) ;
#32778=CARTESIAN_POINT ( 'NONE',  ( 9.984503880673470277, 203.7031108863295401, 29.15113791807856103 ) ) ;
#32780=CARTESIAN_POINT ( 'NONE',  ( 9.984503880673420539, 210.2968891136705167, 102.8488620819214390 ) ) ;
#32785=CARTESIAN_POINT ( 'NONE',  ( -0.05014649552828365914, 215.4116977939061144, 72.24886208192143044 ) ) ;
#32795=CARTESIAN_POINT ( 'NONE',  ( -2.517493886308901807, 199.4062855549015012, 74.90113791807856103 ) ) ;
#32800=CARTESIAN_POINT ( 'NONE',  ( -6.500168698208244500, 211.6636982574061676, 56.79886208192143471 ) ) ;
#32807=CARTESIAN_POINT ( 'NONE',  ( -9.736236675707914401, 199.9851607334237542, 60.20113791807857240 ) ) ;
#32810=CARTESIAN_POINT ( 'NONE',  ( 7.375838497908181246, 196.7627149292499666, -0.5488620819214343749 ) ) ;
#32811=CARTESIAN_POINT ( 'NONE',  ( -10.01549611932653860, 203.7984951890123000, 81.35113791807857808 ) ) ;
#32812=CARTESIAN_POINT ( 'NONE',  ( 7.375838497908012492, 217.2372850707501186, 42.54886208192143471 ) ) ;
#32813=CARTESIAN_POINT ( 'NONE',  ( -10.00000000000000711, 206.9523078486584495, 44.49886208192143755 ) ) ;
#32816=CARTESIAN_POINT ( 'NONE',  ( 0.05014649552807549926, 219.6175466908591716, 82.25113791807856956 ) ) ;
#32817=CARTESIAN_POINT ( 'NONE',  ( -3.044812012440131443, 216.5253028482142952, 1.101137918078565869 ) ) ;
#32819=CARTESIAN_POINT ( 'NONE',  ( 3.044812012439969795, 216.5253028482143520, 60.39886208192143613 ) ) ;
#32823=CARTESIAN_POINT ( 'NONE',  ( 9.736236675708031640, 199.9851607334238963, 73.29886208192142760 ) ) ;
#32826=CARTESIAN_POINT ( 'NONE',  ( 2.426778023690075337, 214.6231898156240447, 39.39886208192144323 ) ) ;
#32832=CARTESIAN_POINT ( 'NONE',  ( -9.040084412992170471, 207.3449885071057395, 103.1858979897393738 ) ) ;
#32833=CARTESIAN_POINT ( 'NONE',  ( 2.517493886308900919, 214.5937144450984420, 61.40113791807856813 ) ) ;
#32835=CARTESIAN_POINT ( 'NONE',  ( 3.044812012439969795, 216.5253028482143520, 39.39886208192143613 ) ) ;
#32842=CARTESIAN_POINT ( 'NONE',  ( 7.984503880673422316, 209.6470497212048372, 21.84886208192143542 ) ) ;
#32843=CARTESIAN_POINT ( 'NONE',  ( 10.01549611932653860, 210.2015048109876716, 64.85113791807857808 ) ) ;
#32844=CARTESIAN_POINT ( 'NONE',  ( -3.044812012440131443, 216.5253028482142952, 43.10113791807857808 ) ) ;
#32847=CARTESIAN_POINT ( 'NONE',  ( 10.00000000000000711, 206.9523078486586201, 14.00113791807856600 ) ) ;
#32848=CARTESIAN_POINT ( 'NONE',  ( -2.517493886308901807, 199.4062855549015012, 8.901137918078566358 ) ) ;
#32852=CARTESIAN_POINT ( 'NONE',  ( 12.01549611932652972, 210.8513442034534933, 25.85113791807856742 ) ) ;
#32855=CARTESIAN_POINT ( 'NONE',  ( -8.118202686958039038, 201.1607312380087080, 78.20113791807857240 ) ) ;
#32856=CARTESIAN_POINT ( 'NONE',  ( -6.220909254589537696, 198.5229672870051445, 45.05113791807856671 ) ) ;
#32860=CARTESIAN_POINT ( 'NONE',  ( -9.736236675708031640, 214.0148392665760753, 11.79886208192143648 ) ) ;
#32861=CARTESIAN_POINT ( 'NONE',  ( 10.01549611932659367, 203.7984951890124421, 16.14886208192143613 ) ) ;
#32864=CARTESIAN_POINT ( 'NONE',  ( -11.98450388067348804, 210.9467285061362247, 54.65113791807857524 ) ) ;
#32865=CARTESIAN_POINT ( 'NONE',  ( 2.426778023690261410, 199.3768101843759837, 80.60113791807857808 ) ) ;
#32867=CARTESIAN_POINT ( 'NONE',  ( 8.062137200540822946, 212.9164362838583315, 30.69886208192144039 ) ) ;
#32877=CARTESIAN_POINT ( 'NONE',  ( 8.015496119326531499, 209.5516654185219636, 28.85113791807856032 ) ) ;
#32879=CARTESIAN_POINT ( 'NONE',  ( -8.062137200540822946, 201.0835637161416400, 17.19886208192143684 ) ) ;
#32882=CARTESIAN_POINT ( 'NONE',  ( -7.984503880673488041, 209.6470497212046098, 54.65113791807857524 ) ) ;
#32886=CARTESIAN_POINT ( 'NONE',  ( 10.00000000000000711, 207.0476921513415220, 102.9988620819214447 ) ) ;
#32888=CARTESIAN_POINT ( 'NONE',  ( -10.00000000000000711, 207.0476921513413515, 36.50113791807857666 ) ) ;
#32891=CARTESIAN_POINT ( 'NONE',  ( -8.118202686958039038, 201.1607312380087080, 21.20113791807856529 ) ) ;
#32896=CARTESIAN_POINT ( 'NONE',  ( 3.044812012440130555, 197.4746971517856764, 101.6011379180785781 ) ) ;
#32901=CARTESIAN_POINT ( 'NONE',  ( -10.01549611932653860, 203.7984951890123284, 48.35113791807855677 ) ) ;
#32907=CARTESIAN_POINT ( 'NONE',  ( -7.375838497908182134, 217.2372850707499765, 27.95113791807857240 ) ) ;
#32910=CARTESIAN_POINT ( 'NONE',  ( 0.05014649552828275708, 196.4853777576173002, 1.748862081921434219 ) ) ;
#32914=CARTESIAN_POINT ( 'NONE',  ( 10.01549611932653860, 210.2015048109876716, 1.851137918078565203 ) ) ;
#32915=CARTESIAN_POINT ( 'NONE',  ( 3.135527875058820690, 216.4958274776887492, 64.40113791807857524 ) ) ;
#32916=CARTESIAN_POINT ( 'NONE',  ( 6.444103211790928043, 211.7408657792734061, 18.69886208192143684 ) ) ;
#32919=CARTESIAN_POINT ( 'NONE',  ( 4.984841277089725686, 213.7757310962907411, 7.551137918078564049 ) ) ;
#32921=CARTESIAN_POINT ( 'NONE',  ( -9.680171189290716072, 199.9079932115567146, 89.19886208192144750 ) ) ;
#32927=CARTESIAN_POINT ( 'NONE',  ( -9.984503880673420539, 203.7031108863293980, 71.34886208192142476 ) ) ;
#32930=CARTESIAN_POINT ( 'NONE',  ( 6.220909254589536808, 215.4770327129947702, 1.551137918078565825 ) ) ;
#32934=CARTESIAN_POINT ( 'NONE',  ( 10.00000000000000711, 206.9523078486586201, 89.00113791807858377 ) ) ;
#32936=CARTESIAN_POINT ( 'NONE',  ( 0.05014649552828262524, 198.5883022060938572, 82.74886208192144466 ) ) ;
#32939=CARTESIAN_POINT ( 'NONE',  ( -3.662846001189865142, 195.5725841191952838, 85.89886208192143613 ) ) ;
#32941=CARTESIAN_POINT ( 'NONE',  ( -6.139770520408368348, 215.5359834540460042, 18.95113791807856884 ) ) ;
#32945=CARTESIAN_POINT ( 'NONE',  ( 9.736236675707914401, 214.0148392665762458, 85.70113791807858661 ) ) ;
#32948=CARTESIAN_POINT ( 'NONE',  ( 12.01549611932659367, 203.1486557965466773, 70.14886208192142192 ) ) ;
#32949=CARTESIAN_POINT ( 'NONE',  ( 10.01549611932659367, 203.7984951890124421, 79.14886208192140771 ) ) ;
#32950=CARTESIAN_POINT ( 'NONE',  ( 12.00000000000000711, 207.0476921513415220, 15.99886208192143400 ) ) ;
#32952=CARTESIAN_POINT ( 'NONE',  ( 6.220909254589536808, 215.4770327129947702, 31.55113791807857382 ) ) ;
#32954=CARTESIAN_POINT ( 'NONE',  ( 8.118202686958138514, 201.1607312380088501, 100.2988620819214418 ) ) ;
#32958=CARTESIAN_POINT ( 'NONE',  ( 2.517493886309087436, 199.4062855549015865, 85.59886208192143897 ) ) ;
#32965=CARTESIAN_POINT ( 'NONE',  ( 4.903702542908601636, 200.1653181626581102, 80.45113791807857240 ) ) ;
#32968=CARTESIAN_POINT ( 'NONE',  ( 6.444103211790928043, 211.7408657792734061, 57.69886208192144039 ) ) ;
#32970=DIRECTION ( 'NONE',  ( -1.000000000000000000, 0.000000000000000000, 0.000000000000000000 ) ) ;
#32975=CARTESIAN_POINT ( 'NONE',  ( 12.00000000000000711, 206.9523078486586485, 59.00113791807856956 ) ) ;
#32977=CARTESIAN_POINT ( 'NONE',  ( 8.118202686958039038, 212.8392687619912635, 100.7011379180785866 ) ) ;
#32979=CARTESIAN_POINT ( 'NONE',  ( -0.05014649552810635652, 196.4853777576173002, 77.75113791807856956 ) ) ;
#32981=CARTESIAN_POINT ( 'NONE',  ( 9.680171189290716072, 214.0920067884432854, 45.69886208192143329 ) ) ;
#32982=CARTESIAN_POINT ( 'NONE',  ( 0.05014649552828275014, 196.4853777576173002, 43.74886208192143044 ) ) ;
#32984=CARTESIAN_POINT ( 'NONE',  ( -7.456977232089304408, 196.8216656703010301, 90.05113791807858092 ) ) ;
#32986=CARTESIAN_POINT ( 'NONE',  ( -6.139770520408369237, 215.5359834540460042, 3.951137918078566180 ) ) ;
#32987=CARTESIAN_POINT ( 'NONE',  ( 0.05014649552828275708, 196.4853777576173002, 67.74886208192140202 ) ) ;
#32990=CARTESIAN_POINT ( 'NONE',  ( 0.05014649552828288198, 194.3824533091408000, 67.74886208192143044 ) ) ;
#32993=CARTESIAN_POINT ( 'NONE',  ( -8.000000000000008882, 206.9523078486584780, 53.49886208192144466 ) ) ;
#33001=CARTESIAN_POINT ( 'NONE',  ( 9.984503880673420539, 210.2968891136705167, 42.84886208192143897 ) ) ;
#33007=CARTESIAN_POINT ( 'NONE',  ( -7.984503880673422316, 204.3529502787951628, 26.34886208192143897 ) ) ;
#33008=CARTESIAN_POINT ( 'NONE',  ( -9.984503880673473830, 210.2968891136704315, 57.65113791807858235 ) ) ;
#33009=CARTESIAN_POINT ( 'NONE',  ( 6.139770520408368348, 198.4640165459539674, 47.45113791807857950 ) ) ;
#33010=CARTESIAN_POINT ( 'NONE',  ( -8.118202686958039038, 201.1607312380087080, 21.20113791807856529 ) ) ;
#33011=CARTESIAN_POINT ( 'NONE',  ( 0.05014649552807626948, 215.4116977939061144, 1.251137918078566225 ) ) ;
#33015=CARTESIAN_POINT ( 'NONE',  ( -7.456977232089304408, 196.8216656703010301, 33.05113791807856671 ) ) ;
#33018=CARTESIAN_POINT ( 'NONE',  ( 10.01549611932653860, 210.2015048109876716, 76.85113791807857808 ) ) ;
#33020=CARTESIAN_POINT ( 'NONE',  ( 0.05014649552810506589, 217.5146222423826714, 52.25113791807856956 ) ) ;
#33024=CARTESIAN_POINT ( 'NONE',  ( 12.00000000000000711, 207.0476921513415220, 9.998862081921435774 ) ) ;
#33025=CARTESIAN_POINT ( 'NONE',  ( -10.01549611932659545, 210.2015048109875011, 20.64886208192143613 ) ) ;
#33028=CARTESIAN_POINT ( 'NONE',  ( 12.00000000000000711, 206.9523078486586485, 59.00113791807856956 ) ) ;
#33030=CARTESIAN_POINT ( 'NONE',  ( -4.984841277089726574, 200.2242689037092305, 75.05113791807858092 ) ) ;
#33031=CARTESIAN_POINT ( 'NONE',  ( 3.044812012439969795, 216.5253028482143520, 45.39886208192143613 ) ) ;
#33035=ADVANCED_FACE ( 'NONE', ( #12358 ), #31741, .T. ) ;
#33041=CARTESIAN_POINT ( 'NONE',  ( 0.05014649552807626948, 215.4116977939061144, 34.25113791807857666 ) ) ;
#33045=CARTESIAN_POINT ( 'NONE',  ( -8.062137200540822946, 201.0835637161416400, 14.19886208192143684 ) ) ;
#33048=CARTESIAN_POINT ( 'NONE',  ( 8.015496119326531499, 209.5516654185219636, 49.85113791807857808 ) ) ;
#33052=CARTESIAN_POINT ( 'NONE',  ( -0.05014649552828403384, 217.5146222423826714, 99.24886208192143044 ) ) ;
#33055=CARTESIAN_POINT ( 'NONE',  ( 3.044812012440130555, 197.4746971517856764, 32.60113791807857098 ) ) ;
#33057=CARTESIAN_POINT ( 'NONE',  ( -10.01549611932653860, 203.7984951890123284, 21.35113791807855677 ) ) ;
#33062=CARTESIAN_POINT ( 'NONE',  ( -9.984503880673473830, 210.2968891136704315, 99.65113791807853261 ) ) ;
#33065=CARTESIAN_POINT ( 'NONE',  ( -10.01549611932653860, 203.7984951890123284, 51.35113791807858519 ) ) ;
#33072=CARTESIAN_POINT ( 'NONE',  ( -12.01549611932652972, 203.1486557965464499, 30.35113791807856742 ) ) ;
#33075=CARTESIAN_POINT ( 'NONE',  ( -6.220909254589682469, 215.4770327129946850, 5.948862081921435063 ) ) ;
#33080=CARTESIAN_POINT ( 'NONE',  ( 9.984503880673470277, 203.7031108863295401, -0.8488620819214341973 ) ) ;
#33081=CARTESIAN_POINT ( 'NONE',  ( -9.984503880673473830, 210.2968891136704315, 63.65113791807857524 ) ) ;
#33084=CARTESIAN_POINT ( 'NONE',  ( -8.015496119326597224, 209.5516654185217362, 23.64886208192143968 ) ) ;
#33089=CARTESIAN_POINT ( 'NONE',  ( 2.426778023690261410, 199.3768101843759837, 2.601137918078566535 ) ) ;
#33092=CARTESIAN_POINT ( 'NONE',  ( -9.680171189290716072, 199.9079932115567146, 86.19886208192144750 ) ) ;
#33097=CARTESIAN_POINT ( 'NONE',  ( 3.135527875058820690, 216.4958274776887492, 1.401137918078565914 ) ) ;
#33098=CARTESIAN_POINT ( 'NONE',  ( -6.139770520408224463, 198.4640165459539389, 68.04886208192142760 ) ) ;
#33102=CARTESIAN_POINT ( 'NONE',  ( -6.220909254589537696, 198.5229672870051161, 6.051137918078566713 ) ) ;
#33107=CARTESIAN_POINT ( 'NONE',  ( -8.062137200540920645, 212.9164362838581894, 90.80113791807858092 ) ) ;
#33109=CARTESIAN_POINT ( 'NONE',  ( -10.00000000000000711, 207.0476921513413515, 78.50113791807856956 ) ) ;
#33112=CARTESIAN_POINT ( 'NONE',  ( 11.98450388067341876, 210.9467285061363953, 90.84886208192142476 ) ) ;
#33113=TOROIDAL_SURFACE ( 'NONE', #30939, 9.624472924841564136, 1.000000000000000444 ) ;
#33115=CARTESIAN_POINT ( 'NONE',  ( 8.118202686958039038, 212.8392687619912635, 25.70113791807856529 ) ) ;
#33119=CARTESIAN_POINT ( 'NONE',  ( -7.375838497908182134, 217.2372850707499765, 90.95113791807855819 ) ) ;
#33122=CARTESIAN_POINT ( 'NONE',  ( 12.01549611932659367, 203.1486557965466773, 73.14886208192142192 ) ) ;
#33123=CARTESIAN_POINT ( 'NONE',  ( -10.01549611932659545, 210.2015048109875011, 89.64886208192143613 ) ) ;
#33124=CARTESIAN_POINT ( 'NONE',  ( -3.753561863808878130, 218.3979405102790281, 9.098862081921435419 ) ) ;
#33127=CARTESIAN_POINT ( 'NONE',  ( -3.044812012440131443, 216.5253028482142952, 28.10113791807857098 ) ) ;
#33129=CARTESIAN_POINT ( 'NONE',  ( 3.044812012439969795, 216.5253028482143520, 96.39886208192145034 ) ) ;
#33137=CARTESIAN_POINT ( 'NONE',  ( -7.984503880673422316, 204.3529502787951628, 77.34886208192143897 ) ) ;
#33148=CARTESIAN_POINT ( 'NONE',  ( 6.444103211791042618, 202.2591342207267644, 83.30113791807858092 ) ) ;
#33152=CARTESIAN_POINT ( 'NONE',  ( -7.984503880673422316, 204.3529502787951628, 50.34886208192144608 ) ) ;
#33159=CARTESIAN_POINT ( 'NONE',  ( -7.456977232089304408, 196.8216656703010301, 54.05113791807856671 ) ) ;
#33160=DIRECTION ( 'NONE',  ( 0.000000000000000000, 0.9988620819214347746, -0.04769215134146093105 ) ) ;
#33161=CARTESIAN_POINT ( 'NONE',  ( 9.680171189290831535, 199.9079932115568852, -0.6988620819214345081 ) ) ;
#33163=CARTESIAN_POINT ( 'NONE',  ( -10.01549611932653860, 203.7984951890123000, 75.35113791807854966 ) ) ;
#33164=CARTESIAN_POINT ( 'NONE',  ( 12.00000000000000711, 207.0476921513415220, 39.99886208192143755 ) ) ;
#33165=CARTESIAN_POINT ( 'NONE',  ( -0.05014649552828402690, 217.5146222423826714, 51.24886208192143755 ) ) ;
#33167=CARTESIAN_POINT ( 'NONE',  ( -7.375838497908182134, 217.2372850707499765, 84.95113791807858661 ) ) ;
#33169=CARTESIAN_POINT ( 'NONE',  ( -3.044812012440131443, 216.5253028482142952, 7.101137918078566535 ) ) ;
#33170=CARTESIAN_POINT ( 'NONE',  ( 8.062137200540822946, 212.9164362838583315, 72.69886208192143329 ) ) ;
#33173=CARTESIAN_POINT ( 'NONE',  ( 3.662846001189864698, 218.4274158808046593, 69.39886208192143613 ) ) ;
#33176=CARTESIAN_POINT ( 'NONE',  ( -6.500168698208244500, 211.6636982574061676, 47.79886208192144181 ) ) ;
#33185=CARTESIAN_POINT ( 'NONE',  ( 10.00000000000000711, 207.0476921513415220, 39.99886208192143755 ) ) ;
#33190=CARTESIAN_POINT ( 'NONE',  ( -8.000000000000008882, 206.9523078486584780, 29.49886208192143400 ) ) ;
#33191=CARTESIAN_POINT ( 'NONE',  ( -8.118202686958039038, 201.1607312380087080, 72.20113791807857240 ) ) ;
#33193=CARTESIAN_POINT ( 'NONE',  ( -9.984503880673473830, 210.2968891136704315, 48.65113791807858235 ) ) ;
#33194=CARTESIAN_POINT ( 'NONE',  ( 6.139770520408368348, 198.4640165459539674, 14.45113791807856352 ) ) ;
#33195=CARTESIAN_POINT ( 'NONE',  ( -6.500168698208129925, 202.3363017425936050, 6.201137918078567068 ) ) ;
#33199=CARTESIAN_POINT ( 'NONE',  ( -12.00000000000000711, 207.0476921513413515, 27.50113791807856956 ) ) ;
#33201=CARTESIAN_POINT ( 'NONE',  ( -10.01549611932653860, 203.7984951890123284, 75.35113791807853545 ) ) ;
#33202=CARTESIAN_POINT ( 'NONE',  ( 10.01549611932653860, 210.2015048109876716, 49.85113791807857808 ) ) ;
#33205=CARTESIAN_POINT ( 'NONE',  ( 7.456977232089471386, 196.8216656703012006, 13.44886208192143684 ) ) ;
#33206=CARTESIAN_POINT ( 'NONE',  ( -8.062137200540822946, 201.0835637161416400, 23.19886208192143684 ) ) ;
#33209=CARTESIAN_POINT ( 'NONE',  ( 3.753561863808689836, 218.3979405102790565, 61.40113791807856103 ) ) ;
#33210=CARTESIAN_POINT ( 'NONE',  ( -6.444103211791042618, 211.7408657792732356, 81.80113791807858092 ) ) ;
#33211=CARTESIAN_POINT ( 'NONE',  ( 8.062137200540822946, 212.9164362838583315, 39.69886208192143329 ) ) ;
#33218=CARTESIAN_POINT ( 'NONE',  ( 10.00000000000000711, 207.0476921513415220, 0.9988620819214341084 ) ) ;
#33220=CARTESIAN_POINT ( 'NONE',  ( -4.903702542908602524, 213.8346818373418898, 27.95113791807857240 ) ) ;
#33223=CARTESIAN_POINT ( 'NONE',  ( -3.135527875058982783, 216.4958274776886924, 15.09886208192143542 ) ) ;
#33226=CARTESIAN_POINT ( 'NONE',  ( -6.500168698208129925, 202.3363017425936050, 63.20113791807857240 ) ) ;
#33229=CARTESIAN_POINT ( 'NONE',  ( -10.00000000000000711, 206.9523078486584495, 104.4988620819214447 ) ) ;
#33231=CARTESIAN_POINT ( 'NONE',  ( 6.220909254589536808, 215.4770327129947702, 46.55113791807856671 ) ) ;
#33233=CARTESIAN_POINT ( 'NONE',  ( -6.220909254589537696, 198.5229672870051161, 15.05113791807856671 ) ) ;
#33240=CARTESIAN_POINT ( 'NONE',  ( 7.375838497908181246, 196.7627149292499666, -0.5488620819214343749 ) ) ;
#33243=CARTESIAN_POINT ( 'NONE',  ( -9.984503880673473830, 210.2968891136704315, 51.65113791807855392 ) ) ;
#33249=CARTESIAN_POINT ( 'NONE',  ( 7.456977232089302632, 217.1783343296989131, 28.55113791807857027 ) ) ;
#33251=CARTESIAN_POINT ( 'NONE',  ( 3.135527875058981895, 197.5041725223112792, 10.59886208192143542 ) ) ;
#33254=CARTESIAN_POINT ( 'NONE',  ( -6.139770520408369237, 215.5359834540460042, 6.951137918078566180 ) ) ;
#33255=CARTESIAN_POINT ( 'NONE',  ( 8.118202686958039038, 212.8392687619912635, 58.70113791807857240 ) ) ;
#33258=CARTESIAN_POINT ( 'NONE',  ( 0.05014649552828262524, 198.5883022060938572, 22.74886208192143755 ) ) ;
#33262=CARTESIAN_POINT ( 'NONE',  ( -8.000000000000008882, 207.0476921513413515, 0.5011379180785658916 ) ) ;
#33264=CARTESIAN_POINT ( 'NONE',  ( -3.753561863808878130, 218.3979405102790281, 93.09886208192145318 ) ) ;
#33270=CARTESIAN_POINT ( 'NONE',  ( 8.062137200540822946, 212.9164362838583315, 69.69886208192144750 ) ) ;
#33273=CARTESIAN_POINT ( 'NONE',  ( -7.898309971686851227, 224.1054302408387287, 103.4854814124441447 ) ) ;
#33277=CARTESIAN_POINT ( 'NONE',  ( 6.139770520408368348, 198.4640165459539674, 89.45113791807857240 ) ) ;
#33279=CARTESIAN_POINT ( 'NONE',  ( 3.135527875058820690, 216.4958274776887492, 79.40113791807857524 ) ) ;
#33282=CARTESIAN_POINT ( 'NONE',  ( 0.05014649552828288198, 194.3824533091408000, 88.74886208192143044 ) ) ;
#33284=CARTESIAN_POINT ( 'NONE',  ( 9.984503880673473830, 203.7031108863295401, 32.15113791807857524 ) ) ;
#33289=CARTESIAN_POINT ( 'NONE',  ( -7.456977232089304408, 196.8216656703010301, 96.05113791807858092 ) ) ;
#33294=CARTESIAN_POINT ( 'NONE',  ( 8.118202686958138514, 201.1607312380088501, 82.29886208192144181 ) ) ;
#33296=CARTESIAN_POINT ( 'NONE',  ( 12.01549611932659367, 203.1486557965466773, 28.14886208192143968 ) ) ;
#33298=CARTESIAN_POINT ( 'NONE',  ( -3.044812012440131443, 216.5253028482142952, 31.10113791807856742 ) ) ;
#33301=CARTESIAN_POINT ( 'NONE',  ( 6.220909254589681581, 198.5229672870052582, 94.44886208192140487 ) ) ;
#33305=CARTESIAN_POINT ( 'NONE',  ( -7.984503880673422316, 204.3529502787951628, 83.34886208192143897 ) ) ;
#33312=CARTESIAN_POINT ( 'NONE',  ( -4.984841277089726574, 200.2242689037092305, 75.05113791807858092 ) ) ;
#33317=CARTESIAN_POINT ( 'NONE',  ( -4.984841277089891776, 213.7757310962905990, 62.94886208192144039 ) ) ;
#33320=CARTESIAN_POINT ( 'NONE',  ( 6.139770520408367460, 198.4640165459539389, 2.451137918078566180 ) ) ;
#33325=CARTESIAN_POINT ( 'NONE',  ( -3.753561863808691168, 195.6020594897209435, 68.90113791807856103 ) ) ;
#33327=CARTESIAN_POINT ( 'NONE',  ( 12.00000000000000711, 206.9523078486586485, 11.00113791807856600 ) ) ;
#33329=CARTESIAN_POINT ( 'NONE',  ( 3.135527875058820690, 216.4958274776887492, 76.40113791807857524 ) ) ;
#33330=CARTESIAN_POINT ( 'NONE',  ( 11.98450388067341876, 210.9467285061363953, 39.84886208192143187 ) ) ;
#33332=CARTESIAN_POINT ( 'NONE',  ( 6.220909254589680693, 198.5229672870052582, 58.44886208192144039 ) ) ;
#33334=CARTESIAN_POINT ( 'NONE',  ( -3.753561863808691168, 195.6020594897209435, 92.90113791807857524 ) ) ;
#33336=CARTESIAN_POINT ( 'NONE',  ( -6.220909254589537696, 198.5229672870051161, 3.051137918078564937 ) ) ;
#33338=CARTESIAN_POINT ( 'NONE',  ( 8.118202686958138514, 201.1607312380088501, 73.29886208192142760 ) ) ;
#33341=CARTESIAN_POINT ( 'NONE',  ( 3.753561863808876797, 195.6020594897209719, 70.59886208192142476 ) ) ;
#33342=CARTESIAN_POINT ( 'NONE',  ( 8.062137200540920645, 201.0835637161417822, 89.30113791807858092 ) ) ;
#33346=CARTESIAN_POINT ( 'NONE',  ( -2.517493886309087880, 214.5937144450984135, 54.09886208192143897 ) ) ;
#33354=CARTESIAN_POINT ( 'NONE',  ( 8.118202686958138514, 201.1607312380088501, 49.29886208192143471 ) ) ;
#33361=CARTESIAN_POINT ( 'NONE',  ( 4.903702542908435547, 213.8346818373419751, 27.54886208192144181 ) ) ;
#33362=CARTESIAN_POINT ( 'NONE',  ( 8.118202686958039038, 212.8392687619912635, 73.70113791807857240 ) ) ;
#33364=CARTESIAN_POINT ( 'NONE',  ( 8.118202686958039038, 212.8392687619912635, 52.70113791807857240 ) ) ;
#33366=CARTESIAN_POINT ( 'NONE',  ( -10.00000000000000711, 207.0476921513413515, 30.50113791807856600 ) ) ;
#33367=CARTESIAN_POINT ( 'NONE',  ( 8.015496119326531499, 209.5516654185219636, 1.851137918078566091 ) ) ;
#33371=CARTESIAN_POINT ( 'NONE',  ( -9.680171189290831535, 214.0920067884431148, 33.80113791807856671 ) ) ;
#33374=CARTESIAN_POINT ( 'NONE',  ( -3.044812012440131443, 216.5253028482142952, 88.10113791807857808 ) ) ;
#33375=CARTESIAN_POINT ( 'NONE',  ( -8.062137200540920645, 212.9164362838581894, 45.80113791807856671 ) ) ;
#33377=CARTESIAN_POINT ( 'NONE',  ( 3.753561863808876797, 195.6020594897209719, 10.59886208192143542 ) ) ;
#33378=CARTESIAN_POINT ( 'NONE',  ( -6.139770520408224463, 198.4640165459539105, 26.04886208192143826 ) ) ;
#33380=VERTEX_POINT ( 'NONE', #13196 ) ;
#33381=CARTESIAN_POINT ( 'NONE',  ( -3.662846001190052991, 218.4274158808045740, 58.10113791807857808 ) ) ;
#33382=CARTESIAN_POINT ( 'NONE',  ( 2.426778023690261410, 199.3768101843759837, 77.60113791807854966 ) ) ;
#33383=CARTESIAN_POINT ( 'NONE',  ( -10.01549611932659722, 210.2015048109875011, 41.64886208192144323 ) ) ;
#33386=CARTESIAN_POINT ( 'NONE',  ( -12.01549611932659722, 210.8513442034533227, 38.64886208192143613 ) ) ;
#33394=CARTESIAN_POINT ( 'NONE',  ( 8.000000000000008882, 206.9523078486586485, 29.00113791807856956 ) ) ;
#33397=CARTESIAN_POINT ( 'NONE',  ( 8.062137200540822946, 212.9164362838583315, 12.69886208192143506 ) ) ;
#33401=CARTESIAN_POINT ( 'NONE',  ( -7.984503880673488041, 209.6470497212046098, 57.65113791807858945 ) ) ;
#33403=CARTESIAN_POINT ( 'NONE',  ( -10.00000000000000711, 206.9523078486584495, 101.4988620819214304 ) ) ;
#33405=CARTESIAN_POINT ( 'NONE',  ( 9.984503880673470277, 203.7031108863295401, 41.15113791807855392 ) ) ;
#33406=CARTESIAN_POINT ( 'NONE',  ( -6.220909254589537696, 198.5229672870051161, 21.05113791807855961 ) ) ;
#33412=CARTESIAN_POINT ( 'NONE',  ( -12.01549611932652972, 203.1486557965464499, 0.3511379180785654808 ) ) ;
#33415=CARTESIAN_POINT ( 'NONE',  ( 8.118202686958039038, 212.8392687619912635, 43.70113791807857240 ) ) ;
#33421=CARTESIAN_POINT ( 'NONE',  ( -3.753561863808691168, 195.6020594897209435, 26.90113791807856813 ) ) ;
#33425=CARTESIAN_POINT ( 'NONE',  ( 8.118202686958138514, 201.1607312380088501, 7.298862081921435596 ) ) ;
#33427=CARTESIAN_POINT ( 'NONE',  ( 8.062137200540920645, 201.0835637161417822, 11.30113791807856671 ) ) ;
#33428=CARTESIAN_POINT ( 'NONE',  ( 0.05014649552810505201, 217.5146222423826714, 67.25113791807856956 ) ) ;
#33430=CARTESIAN_POINT ( 'NONE',  ( -6.500168698208244500, 211.6636982574061676, 20.79886208192143826 ) ) ;
#33433=ORIENTED_EDGE ( 'NONE', *, *, #30736, .T. ) ;
#33434=CARTESIAN_POINT ( 'NONE',  ( 8.015496119326531499, 209.5516654185219636, 7.851137918078565647 ) ) ;
#33435=CARTESIAN_POINT ( 'NONE',  ( -12.00000000000000711, 206.9523078486584780, 89.49886208192144466 ) ) ;
#33440=CARTESIAN_POINT ( 'NONE',  ( -0.05014649552810635652, 196.4853777576173002, 11.75113791807856778 ) ) ;
#33442=CARTESIAN_POINT ( 'NONE',  ( 9.984503880673420539, 210.2968891136705167, 72.84886208192143897 ) ) ;
#33445=CARTESIAN_POINT ( 'NONE',  ( -3.135527875058821579, 197.5041725223112223, 17.90113791807856458 ) ) ;
#33448=CARTESIAN_POINT ( 'NONE',  ( -10.01549611932653860, 203.7984951890123284, 102.3511379180785781 ) ) ;
#33451=CARTESIAN_POINT ( 'NONE',  ( -0.05014649552810635652, 196.4853777576173002, 77.75113791807856956 ) ) ;
#33453=CARTESIAN_POINT ( 'NONE',  ( -3.753561863808878130, 218.3979405102790281, 87.09886208192143897 ) ) ;
#33458=CARTESIAN_POINT ( 'NONE',  ( -3.662846001190052991, 218.4274158808045740, 94.10113791807857808 ) ) ;
#33462=CARTESIAN_POINT ( 'NONE',  ( -0.05014649552828402690, 217.5146222423826714, 84.24886208192143044 ) ) ;
#33463=CARTESIAN_POINT ( 'NONE',  ( -9.736236675708031640, 214.0148392665760753, 23.79886208192143826 ) ) ;
#33466=CARTESIAN_POINT ( 'NONE',  ( -0.05014649552810635652, 196.4853777576173002, 38.75113791807856956 ) ) ;
#33468=CARTESIAN_POINT ( 'NONE',  ( 9.984503880673420539, 210.2968891136705167, 99.84886208192141055 ) ) ;
#33473=CARTESIAN_POINT ( 'NONE',  ( -6.500168698208244500, 211.6636982574061676, 80.79886208192144181 ) ) ;
#33478=CARTESIAN_POINT ( 'NONE',  ( -4.984841277089726574, 200.2242689037092305, 60.05113791807858092 ) ) ;
#33482=CARTESIAN_POINT ( 'NONE',  ( -2.426778023690262742, 214.6231898156240163, 91.10113791807859229 ) ) ;
#33485=CARTESIAN_POINT ( 'NONE',  ( 0.05014649552828262524, 198.5883022060938572, 61.74886208192144466 ) ) ;
#33488=CARTESIAN_POINT ( 'NONE',  ( -10.01549611932653860, 203.7984951890123000, 0.3511379180785656473 ) ) ;
#33493=CARTESIAN_POINT ( 'NONE',  ( -3.753561863808691168, 195.6020594897209435, 65.90113791807856103 ) ) ;
#33495=CARTESIAN_POINT ( 'NONE',  ( 12.00000000000000711, 206.9523078486586485, 14.00113791807856600 ) ) ;
#33496=CARTESIAN_POINT ( 'NONE',  ( -6.139770520408368348, 215.5359834540460042, 87.95113791807858661 ) ) ;
#33497=CARTESIAN_POINT ( 'NONE',  ( -7.375838497908014268, 196.7627149292498530, 53.04886208192142760 ) ) ;
#33498=CARTESIAN_POINT ( 'NONE',  ( -0.05014649552828402690, 217.5146222423826714, 54.24886208192143044 ) ) ;
#33500=CARTESIAN_POINT ( 'NONE',  ( 9.680171189290831535, 199.9079932115568852, 92.30113791807858092 ) ) ;
#33502=CARTESIAN_POINT ( 'NONE',  ( -9.984503880673473830, 210.2968891136704315, 6.651137918078564581 ) ) ;
#33503=CARTESIAN_POINT ( 'NONE',  ( -6.220909254589682469, 215.4770327129946850, 65.94886208192144750 ) ) ;
#33505=CARTESIAN_POINT ( 'NONE',  ( 11.98450388067341876, 210.9467285061363953, 81.84886208192142476 ) ) ;
#33506=CARTESIAN_POINT ( 'NONE',  ( -10.01549611932653860, 203.7984951890123284, 87.35113791807854966 ) ) ;
#33509=CARTESIAN_POINT ( 'NONE',  ( 4.984841277089891776, 200.2242689037093726, 52.44886208192144039 ) ) ;
#33518=CARTESIAN_POINT ( 'NONE',  ( 9.984503880673420539, 210.2968891136705167, 48.84886208192143187 ) ) ;
#33525=CARTESIAN_POINT ( 'NONE',  ( -8.015496119326597224, 209.5516654185217362, 35.64886208192143613 ) ) ;
#33527=CARTESIAN_POINT ( 'NONE',  ( 8.062137200540920645, 201.0835637161417822, 71.30113791807856671 ) ) ;
#33529=CARTESIAN_POINT ( 'NONE',  ( 3.135527875058820690, 216.4958274776887492, 55.40113791807857524 ) ) ;
#33530=CARTESIAN_POINT ( 'NONE',  ( 8.062137200540920645, 201.0835637161417822, 26.30113791807856671 ) ) ;
#33531=CARTESIAN_POINT ( 'NONE',  ( -4.903702542908602524, 213.8346818373418898, 9.951137918078567068 ) ) ;
#33535=CARTESIAN_POINT ( 'NONE',  ( -9.680171189290831535, 214.0920067884431148, 39.80113791807857382 ) ) ;
#33537=CARTESIAN_POINT ( 'NONE',  ( -8.062137200540920645, 212.9164362838581894, 87.80113791807856671 ) ) ;
#33538=CARTESIAN_POINT ( 'NONE',  ( -3.135527875058821579, 197.5041725223112223, 62.90113791807858235 ) ) ;
#33540=CARTESIAN_POINT ( 'NONE',  ( -0.05014649552828442242, 219.6175466908591716, 27.24886208192143755 ) ) ;
#33541=CARTESIAN_POINT ( 'NONE',  ( 8.118202686958138514, 201.1607312380088501, 28.29886208192143471 ) ) ;
#33544=CARTESIAN_POINT ( 'NONE',  ( 9.680171189290831535, 199.9079932115568852, 68.30113791807856671 ) ) ;
#33545=CARTESIAN_POINT ( 'NONE',  ( 8.015496119326531499, 209.5516654185219636, 82.85113791807857808 ) ) ;
#33546=CARTESIAN_POINT ( 'NONE',  ( -10.00000000000000711, 206.9523078486584495, 41.49886208192143044 ) ) ;
#33550=CARTESIAN_POINT ( 'NONE',  ( -12.00000000000000711, 206.9523078486584780, 44.49886208192143755 ) ) ;
#33551=AXIS2_PLACEMENT_3D ( 'NONE', #30064, #6894, #17121 ) ;
#33559=CARTESIAN_POINT ( 'NONE',  ( 6.444103211791042618, 202.2591342207267644, 44.30113791807857382 ) ) ;
#33562=CARTESIAN_POINT ( 'NONE',  ( 3.044812012439969795, 216.5253028482143520, 24.39886208192143613 ) ) ;
#33567=CARTESIAN_POINT ( 'NONE',  ( -6.500168698208244500, 211.6636982574061676, 5.798862081921435596 ) ) ;
#33568=CARTESIAN_POINT ( 'NONE',  ( 10.01549611932653860, 210.2015048109876716, 40.85113791807857098 ) ) ;
#33570=CARTESIAN_POINT ( 'NONE',  ( -6.139770520408369237, 215.5359834540460042, 24.95113791807855819 ) ) ;
#33571=CARTESIAN_POINT ( 'NONE',  ( -10.00000000000000178, 206.9999999999998863, 103.5000000000000426 ) ) ;
#33575=CARTESIAN_POINT ( 'NONE',  ( 6.500168698208244500, 202.3363017425938324, 82.29886208192144181 ) ) ;
#33579=CARTESIAN_POINT ( 'NONE',  ( -9.736236675707914401, 199.9851607334237542, 6.201137918078565292 ) ) ;
#33582=CARTESIAN_POINT ( 'NONE',  ( 6.220909254589536808, 215.4770327129947702, 55.55113791807855961 ) ) ;
#33586=CARTESIAN_POINT ( 'NONE',  ( 8.118202686958138514, 201.1607312380088501, 4.298862081921434708 ) ) ;
#33589=CARTESIAN_POINT ( 'NONE',  ( 9.736236675707914401, 214.0148392665762458, 40.70113791807857240 ) ) ;
#33591=CARTESIAN_POINT ( 'NONE',  ( -8.062137200540822946, 201.0835637161416400, 14.19886208192143684 ) ) ;
#33594=CARTESIAN_POINT ( 'NONE',  ( -0.05014649552810635652, 196.4853777576173002, 8.751137918078562450 ) ) ;
#33595=CARTESIAN_POINT ( 'NONE',  ( -0.05014649552810635652, 196.4853777576173002, 68.75113791807855534 ) ) ;
#33598=CARTESIAN_POINT ( 'NONE',  ( -0.05014649552828365914, 215.4116977939061144, 33.24886208192144466 ) ) ;
#33604=CARTESIAN_POINT ( 'NONE',  ( -8.000000000000008882, 207.0476921513413515, 15.50113791807856600 ) ) ;
#33605=CARTESIAN_POINT ( 'NONE',  ( -3.753561863808878130, 218.3979405102790281, 96.09886208192143897 ) ) ;
#33607=ORIENTED_EDGE ( 'NONE', *, *, #22607, .T. ) ;
#33610=CARTESIAN_POINT ( 'NONE',  ( 10.00000000000000711, 206.9523078486586201, 11.00113791807856600 ) ) ;
#33611=CARTESIAN_POINT ( 'NONE',  ( 8.062137200540822946, 212.9164362838583315, 75.69886208192143329 ) ) ;
#33614=CARTESIAN_POINT ( 'NONE',  ( -10.01549611932653860, 203.7984951890123284, 15.35113791807856565 ) ) ;
#33617=CARTESIAN_POINT ( 'NONE',  ( -8.118202686958039038, 201.1607312380087080, 102.2011379180785866 ) ) ;
#33619=CARTESIAN_POINT ( 'NONE',  ( 9.984503880673470277, 203.7031108863295401, 80.15113791807858945 ) ) ;
#33623=CARTESIAN_POINT ( 'NONE',  ( 12.00000000000000711, 207.0476921513415220, 99.99886208192143044 ) ) ;
#33630=CARTESIAN_POINT ( 'NONE',  ( 3.662846001190051659, 195.5725841191953691, 92.60113791807857808 ) ) ;
#33631=CARTESIAN_POINT ( 'NONE',  ( -10.84125907834625480, 206.4200127656791039, 104.0062660280915026 ) ) ;
#33633=CARTESIAN_POINT ( 'NONE',  ( -3.135527875058982783, 216.4958274776886924, 87.09886208192143897 ) ) ;
#33634=CARTESIAN_POINT ( 'NONE',  ( -12.01549611932659722, 210.8513442034533227, 20.64886208192143613 ) ) ;
#33636=CARTESIAN_POINT ( 'NONE',  ( 3.044812012440130555, 197.4746971517856764, 38.60113791807857098 ) ) ;
#33637=ORIENTED_EDGE ( 'NONE', *, *, #9983, .T. ) ;
#33638=CARTESIAN_POINT ( 'NONE',  ( -4.984841277089891776, 213.7757310962905990, 2.948862081921435063 ) ) ;
#33641=CARTESIAN_POINT ( 'NONE',  ( 6.500168698208244500, 202.3363017425938324, 79.29886208192144181 ) ) ;
#33644=DIRECTION ( 'NONE',  ( 5.620504062164857944E-16, -0.9988620819214347746, 0.04769215134146256169 ) ) ;
#33647=CARTESIAN_POINT ( 'NONE',  ( -7.984503880673488041, 209.6470497212046098, 57.65113791807858945 ) ) ;
#33650=CARTESIAN_POINT ( 'NONE',  ( -6.500168698208129925, 202.3363017425936050, 90.20113791807857240 ) ) ;
#33656=CARTESIAN_POINT ( 'NONE',  ( -6.444103211790928043, 202.2591342207265939, 68.19886208192143329 ) ) ;
#33661=CARTESIAN_POINT ( 'NONE',  ( -0.05014649552810635652, 196.4853777576173002, 2.751137918078565558 ) ) ;
#33665=CARTESIAN_POINT ( 'NONE',  ( 3.662846001190051659, 195.5725841191953691, 65.60113791807857808 ) ) ;
#33669=CARTESIAN_POINT ( 'NONE',  ( -7.375838497908182134, 217.2372850707499765, 9.951137918078567068 ) ) ;
#33670=CARTESIAN_POINT ( 'NONE',  ( 0.05014649552810506589, 217.5146222423826714, 85.25113791807855534 ) ) ;
#33671=CARTESIAN_POINT ( 'NONE',  ( -11.98450388067341876, 203.0532714938636047, 47.34886208192143897 ) ) ;
#33672=CARTESIAN_POINT ( 'NONE',  ( -3.044812012439970683, 197.4746971517856196, 52.89886208192143613 ) ) ;
#33674=CARTESIAN_POINT ( 'NONE',  ( -7.375838497908182134, 217.2372850707499765, 93.95113791807857240 ) ) ;
#33676=CARTESIAN_POINT ( 'NONE',  ( 0.05014649552810505201, 217.5146222423826714, 10.25113791807856778 ) ) ;
#33677=CARTESIAN_POINT ( 'NONE',  ( -6.220909254589682469, 215.4770327129946850, 68.94886208192140487 ) ) ;
#33679=CARTESIAN_POINT ( 'NONE',  ( 0.05014649552828288198, 194.3824533091408000, 76.74886208192144466 ) ) ;
#33680=CARTESIAN_POINT ( 'NONE',  ( -3.044812012440131443, 216.5253028482142952, 94.10113791807857808 ) ) ;
#33683=CARTESIAN_POINT ( 'NONE',  ( -8.000000000000008882, 206.9523078486584780, 50.49886208192144466 ) ) ;
ENDSEC;
END-ISO-10303-21;
